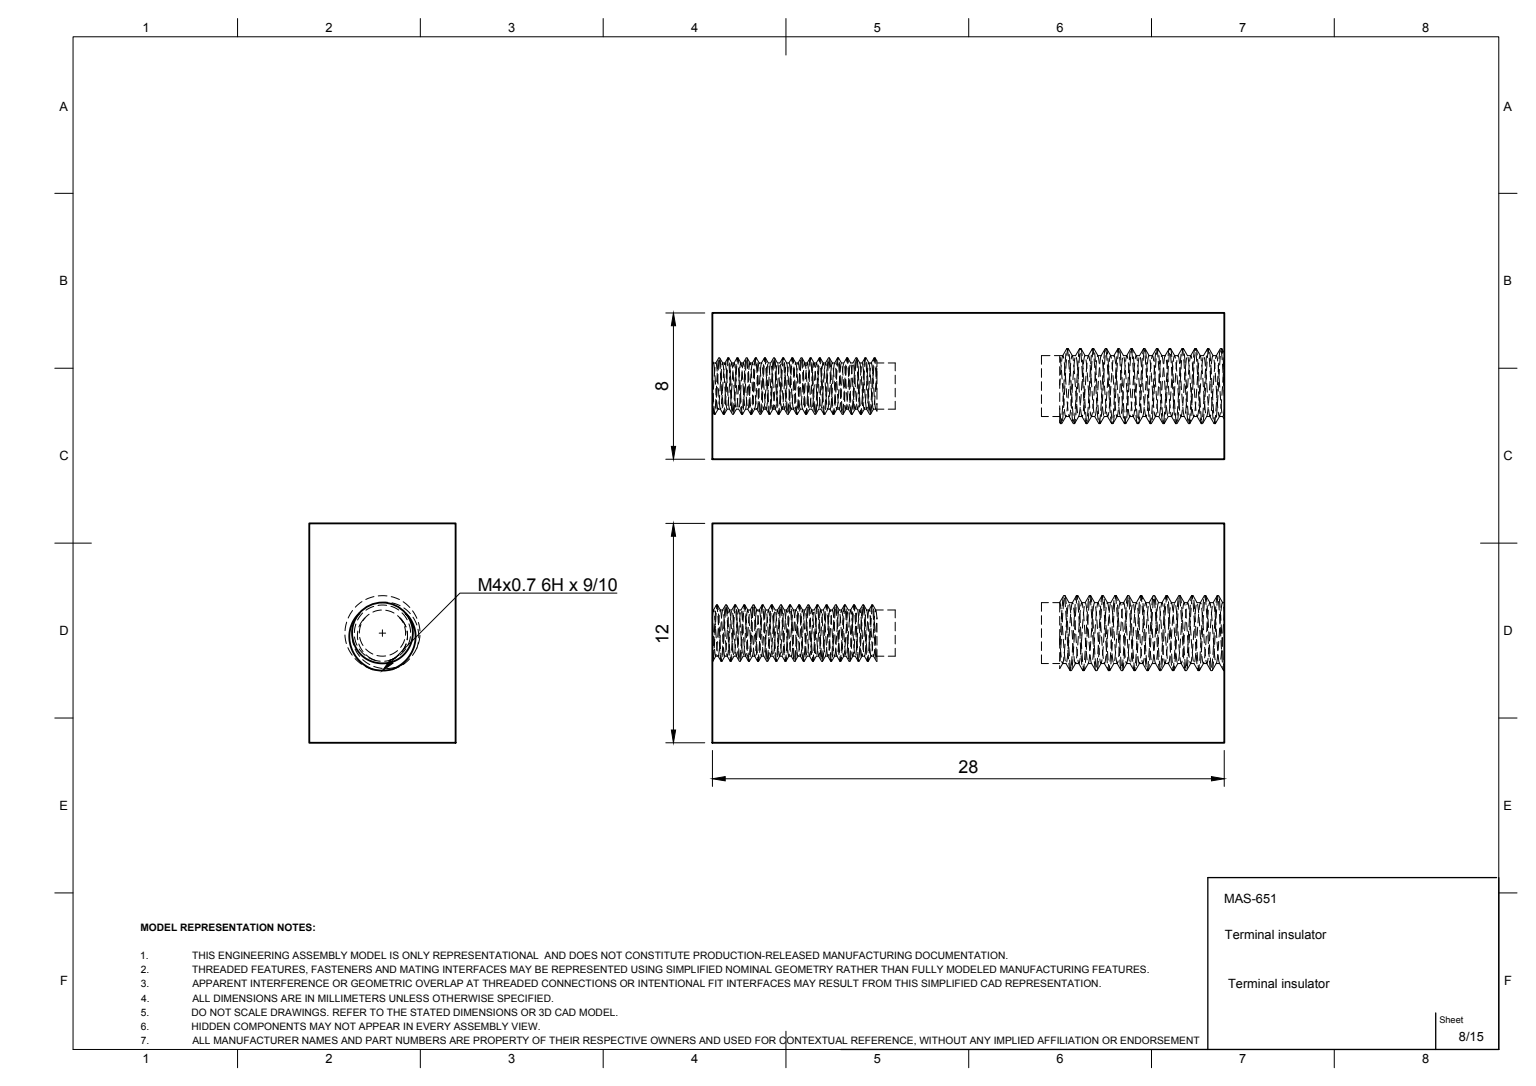
ISO-10303-21;
HEADER;
/* Generated by software containing ST-Developer
 * from STEP Tools, Inc. (www.steptools.com) 
 */

FILE_DESCRIPTION(
/* description */ ('Independent direct-acting normally-closed roller-plunger limit-switch
 CAD. Removable cover, insulated terminal supports, captured bus/conta
ct bridge, native Coil return spring, integral lower travel stop, reus
able instanced hardware and free roller. Manual geometric contact open
ing4mm; no snap-action/contact-force, electrical/current/voltage, envi
ronmental seal, safety-switch, wear, load or life certification. Exter
nal wiring and anchors omitted; fits and application engineering requi
red.'),
/* implementation_level */ '2;1');

FILE_NAME(
/* name */ 'Terminal insulator.step',
/* time_stamp */ '2026-11-08T07:32:43-08:00',
/* author */ (''),
/* organization */ (''),
/* preprocessor_version */ 'ST-DEVELOPER v20.2',
/* originating_system */ 'Autodesk Translation Framework v15.17.0.0',
/* authorisation */ '');

FILE_SCHEMA (('AUTOMOTIVE_DESIGN { 1 0 10303 214 3 1 1 }'));
ENDSEC;

DATA;
#10=MECHANICAL_DESIGN_GEOMETRIC_PRESENTATION_REPRESENTATION('',(#182),#36482);
#148=SHAPE_REPRESENTATION_RELATIONSHIP('SRR','None',#36561,#165);
#165=ADVANCED_BREP_SHAPE_REPRESENTATION('',(#199),#36471);
#182=STYLED_ITEM('',(#36655),#199);
#199=MANIFOLD_SOLID_BREP('Body1',#9773);
#222=B_SPLINE_SURFACE_WITH_KNOTS('',3,3,((#25543,#25544,#25545,#25546,#25547,
#25548,#25549,#25550,#25551,#25552,#25553,#25554,#25555,#25556,#25557,#25558,
#25559,#25560,#25561,#25562,#25563,#25564,#25565,#25566,#25567,#25568,#25569,
#25570,#25571,#25572,#25573,#25574,#25575,#25576,#25577,#25578,#25579,#25580,
#25581,#25582,#25583,#25584,#25585,#25586,#25587,#25588,#25589,#25590,#25591,
#25592,#25593,#25594,#25595,#25596,#25597,#25598,#25599,#25600,#25601,#25602,
#25603,#25604,#25605,#25606,#25607,#25608,#25609,#25610,#25611,#25612,#25613,
#25614,#25615,#25616,#25617,#25618,#25619,#25620,#25621,#25622,#25623,#25624,
#25625,#25626,#25627,#25628,#25629,#25630,#25631,#25632,#25633,#25634,#25635,
#25636,#25637,#25638,#25639,#25640,#25641,#25642,#25643,#25644,#25645,#25646,
#25647,#25648,#25649,#25650,#25651,#25652,#25653,#25654,#25655,#25656,#25657,
#25658,#25659,#25660,#25661),(#25662,#25663,#25664,#25665,#25666,#25667,
#25668,#25669,#25670,#25671,#25672,#25673,#25674,#25675,#25676,#25677,#25678,
#25679,#25680,#25681,#25682,#25683,#25684,#25685,#25686,#25687,#25688,#25689,
#25690,#25691,#25692,#25693,#25694,#25695,#25696,#25697,#25698,#25699,#25700,
#25701,#25702,#25703,#25704,#25705,#25706,#25707,#25708,#25709,#25710,#25711,
#25712,#25713,#25714,#25715,#25716,#25717,#25718,#25719,#25720,#25721,#25722,
#25723,#25724,#25725,#25726,#25727,#25728,#25729,#25730,#25731,#25732,#25733,
#25734,#25735,#25736,#25737,#25738,#25739,#25740,#25741,#25742,#25743,#25744,
#25745,#25746,#25747,#25748,#25749,#25750,#25751,#25752,#25753,#25754,#25755,
#25756,#25757,#25758,#25759,#25760,#25761,#25762,#25763,#25764,#25765,#25766,
#25767,#25768,#25769,#25770,#25771,#25772,#25773,#25774,#25775,#25776,#25777,
#25778,#25779,#25780),(#25781,#25782,#25783,#25784,#25785,#25786,#25787,
#25788,#25789,#25790,#25791,#25792,#25793,#25794,#25795,#25796,#25797,#25798,
#25799,#25800,#25801,#25802,#25803,#25804,#25805,#25806,#25807,#25808,#25809,
#25810,#25811,#25812,#25813,#25814,#25815,#25816,#25817,#25818,#25819,#25820,
#25821,#25822,#25823,#25824,#25825,#25826,#25827,#25828,#25829,#25830,#25831,
#25832,#25833,#25834,#25835,#25836,#25837,#25838,#25839,#25840,#25841,#25842,
#25843,#25844,#25845,#25846,#25847,#25848,#25849,#25850,#25851,#25852,#25853,
#25854,#25855,#25856,#25857,#25858,#25859,#25860,#25861,#25862,#25863,#25864,
#25865,#25866,#25867,#25868,#25869,#25870,#25871,#25872,#25873,#25874,#25875,
#25876,#25877,#25878,#25879,#25880,#25881,#25882,#25883,#25884,#25885,#25886,
#25887,#25888,#25889,#25890,#25891,#25892,#25893,#25894,#25895,#25896,#25897,
#25898,#25899),(#25900,#25901,#25902,#25903,#25904,#25905,#25906,#25907,
#25908,#25909,#25910,#25911,#25912,#25913,#25914,#25915,#25916,#25917,#25918,
#25919,#25920,#25921,#25922,#25923,#25924,#25925,#25926,#25927,#25928,#25929,
#25930,#25931,#25932,#25933,#25934,#25935,#25936,#25937,#25938,#25939,#25940,
#25941,#25942,#25943,#25944,#25945,#25946,#25947,#25948,#25949,#25950,#25951,
#25952,#25953,#25954,#25955,#25956,#25957,#25958,#25959,#25960,#25961,#25962,
#25963,#25964,#25965,#25966,#25967,#25968,#25969,#25970,#25971,#25972,#25973,
#25974,#25975,#25976,#25977,#25978,#25979,#25980,#25981,#25982,#25983,#25984,
#25985,#25986,#25987,#25988,#25989,#25990,#25991,#25992,#25993,#25994,#25995,
#25996,#25997,#25998,#25999,#26000,#26001,#26002,#26003,#26004,#26005,#26006,
#26007,#26008,#26009,#26010,#26011,#26012,#26013,#26014,#26015,#26016,#26017,
#26018)),.UNSPECIFIED.,.F.,.F.,.F.,(4,4),(4,1,1,1,1,1,1,1,1,1,1,1,1,1,1,
1,1,1,1,1,1,1,1,1,1,1,1,1,1,1,1,1,1,1,1,1,1,1,1,1,1,1,1,1,1,1,1,1,1,1,1,
1,1,1,1,1,1,1,1,1,1,1,1,1,1,1,1,1,1,1,1,1,1,1,1,1,1,1,1,1,1,1,1,1,1,1,1,
1,1,1,1,1,1,1,1,1,1,1,1,1,1,1,1,1,1,1,1,1,1,1,1,1,1,1,1,1,4),(0.,0.0321584099938621),
(11.8553612635792,12.8477570223809,13.8401527811825,14.8325485399841,15.8249442987858,
16.8173400575874,17.809735816389,18.8021315751907,19.7945273339923,20.7869230927939,
21.7793188515956,22.7717146103972,23.7641103691988,24.7565061280005,25.7489018868021,
26.7412976456037,27.7336934044054,28.726089163207,29.7184849220086,30.7108806808103,
31.7032764396119,32.6956721984135,33.6880679572152,34.6804637160168,35.6728594748184,
36.6652552336201,37.6576509924217,38.6500467512233,39.642442510025,40.6348382688266,
41.6272340276282,42.6196297864299,43.6120255452315,44.6044213040331,45.5968170628348,
46.5892128216364,47.581608580438,48.5740043392397,49.5664000980413,50.5587958568429,
51.5511916156446,52.5435873744462,53.5359831332478,54.5283788920495,55.5207746508511,
56.5131704096527,57.5055661684544,58.497961927256,59.4903576860576,60.4827534448593,
61.4751492036609,62.4675449624625,63.4599407212642,64.4523364800658,65.4447322388674,
66.4371279976691,67.4295237564707,68.4219195152723,69.4143152740739,70.4067110328756,
71.3991067916772,72.3915025504788,73.3838983092805,74.3762940680821,75.3686898268838,
76.3610855856854,77.353481344487,78.3458771032886,79.3382728620903,80.3306686208919,
81.3230643796935,82.3154601384952,83.3078558972968,84.3002516560985,85.2926474149001,
86.2850431737017,87.2774389325033,88.269834691305,89.2622304501066,90.2546262089082,
91.2470219677099,92.2394177265115,93.2318134853131,94.2242092441148,95.2166050029164,
96.209000761718,97.2013965205197,98.1937922793213,99.1861880381229,100.178583796925,
101.170979555726,102.163375314528,103.155771073329,104.148166832131,105.140562590933,
106.132958349734,107.125354108536,108.117749867338,109.110145626139,110.102541384941,
111.094937143743,112.087332902544,113.079728661346,114.072124420147,115.064520178949,
116.056915937751,117.049311696552,118.041707455354,119.034103214156,120.026498972957,
121.018894731759,122.01129049056,123.003686249362,123.996082008164,124.988477766965,
125.980873525767,126.973269284569),.UNSPECIFIED.);
#223=B_SPLINE_SURFACE_WITH_KNOTS('',3,3,((#26093,#26094,#26095,#26096,#26097,
#26098,#26099,#26100,#26101,#26102,#26103,#26104,#26105,#26106,#26107,#26108,
#26109,#26110,#26111,#26112,#26113,#26114,#26115,#26116,#26117,#26118,#26119,
#26120,#26121,#26122,#26123,#26124,#26125,#26126,#26127,#26128,#26129,#26130,
#26131,#26132,#26133,#26134,#26135,#26136,#26137,#26138,#26139,#26140,#26141,
#26142,#26143,#26144,#26145,#26146,#26147,#26148,#26149,#26150,#26151,#26152,
#26153,#26154,#26155,#26156,#26157,#26158,#26159,#26160,#26161,#26162,#26163,
#26164,#26165,#26166,#26167,#26168,#26169,#26170,#26171,#26172,#26173,#26174,
#26175,#26176,#26177,#26178,#26179,#26180,#26181,#26182,#26183,#26184,#26185,
#26186,#26187,#26188,#26189,#26190,#26191,#26192,#26193,#26194,#26195,#26196,
#26197,#26198,#26199,#26200,#26201,#26202,#26203,#26204,#26205,#26206,#26207,
#26208,#26209,#26210,#26211),(#26212,#26213,#26214,#26215,#26216,#26217,
#26218,#26219,#26220,#26221,#26222,#26223,#26224,#26225,#26226,#26227,#26228,
#26229,#26230,#26231,#26232,#26233,#26234,#26235,#26236,#26237,#26238,#26239,
#26240,#26241,#26242,#26243,#26244,#26245,#26246,#26247,#26248,#26249,#26250,
#26251,#26252,#26253,#26254,#26255,#26256,#26257,#26258,#26259,#26260,#26261,
#26262,#26263,#26264,#26265,#26266,#26267,#26268,#26269,#26270,#26271,#26272,
#26273,#26274,#26275,#26276,#26277,#26278,#26279,#26280,#26281,#26282,#26283,
#26284,#26285,#26286,#26287,#26288,#26289,#26290,#26291,#26292,#26293,#26294,
#26295,#26296,#26297,#26298,#26299,#26300,#26301,#26302,#26303,#26304,#26305,
#26306,#26307,#26308,#26309,#26310,#26311,#26312,#26313,#26314,#26315,#26316,
#26317,#26318,#26319,#26320,#26321,#26322,#26323,#26324,#26325,#26326,#26327,
#26328,#26329,#26330),(#26331,#26332,#26333,#26334,#26335,#26336,#26337,
#26338,#26339,#26340,#26341,#26342,#26343,#26344,#26345,#26346,#26347,#26348,
#26349,#26350,#26351,#26352,#26353,#26354,#26355,#26356,#26357,#26358,#26359,
#26360,#26361,#26362,#26363,#26364,#26365,#26366,#26367,#26368,#26369,#26370,
#26371,#26372,#26373,#26374,#26375,#26376,#26377,#26378,#26379,#26380,#26381,
#26382,#26383,#26384,#26385,#26386,#26387,#26388,#26389,#26390,#26391,#26392,
#26393,#26394,#26395,#26396,#26397,#26398,#26399,#26400,#26401,#26402,#26403,
#26404,#26405,#26406,#26407,#26408,#26409,#26410,#26411,#26412,#26413,#26414,
#26415,#26416,#26417,#26418,#26419,#26420,#26421,#26422,#26423,#26424,#26425,
#26426,#26427,#26428,#26429,#26430,#26431,#26432,#26433,#26434,#26435,#26436,
#26437,#26438,#26439,#26440,#26441,#26442,#26443,#26444,#26445,#26446,#26447,
#26448,#26449),(#26450,#26451,#26452,#26453,#26454,#26455,#26456,#26457,
#26458,#26459,#26460,#26461,#26462,#26463,#26464,#26465,#26466,#26467,#26468,
#26469,#26470,#26471,#26472,#26473,#26474,#26475,#26476,#26477,#26478,#26479,
#26480,#26481,#26482,#26483,#26484,#26485,#26486,#26487,#26488,#26489,#26490,
#26491,#26492,#26493,#26494,#26495,#26496,#26497,#26498,#26499,#26500,#26501,
#26502,#26503,#26504,#26505,#26506,#26507,#26508,#26509,#26510,#26511,#26512,
#26513,#26514,#26515,#26516,#26517,#26518,#26519,#26520,#26521,#26522,#26523,
#26524,#26525,#26526,#26527,#26528,#26529,#26530,#26531,#26532,#26533,#26534,
#26535,#26536,#26537,#26538,#26539,#26540,#26541,#26542,#26543,#26544,#26545,
#26546,#26547,#26548,#26549,#26550,#26551,#26552,#26553,#26554,#26555,#26556,
#26557,#26558,#26559,#26560,#26561,#26562,#26563,#26564,#26565,#26566,#26567,
#26568)),.UNSPECIFIED.,.F.,.F.,.F.,(4,4),(4,1,1,1,1,1,1,1,1,1,1,1,1,1,1,
1,1,1,1,1,1,1,1,1,1,1,1,1,1,1,1,1,1,1,1,1,1,1,1,1,1,1,1,1,1,1,1,1,1,1,1,
1,1,1,1,1,1,1,1,1,1,1,1,1,1,1,1,1,1,1,1,1,1,1,1,1,1,1,1,1,1,1,1,1,1,1,1,
1,1,1,1,1,1,1,1,1,1,1,1,1,1,1,1,1,1,1,1,1,1,1,1,1,1,1,1,1,4),(0.,0.0321584099938621),
(14.3984001269718,15.3907958857734,16.383191644575,17.3755874033767,18.3679831621783,
19.3603789209799,20.3527746797816,21.3451704385832,22.3375661973848,23.3299619561865,
24.3223577149881,25.3147534737897,26.3071492325914,27.299544991393,28.2919407501946,
29.2843365089963,30.2767322677979,31.2691280265995,32.2615237854012,33.2539195442028,
34.2463153030044,35.2387110618061,36.2311068206077,37.2235025794093,38.215898338211,
39.2082940970126,40.2006898558142,41.1930856146159,42.1854813734175,43.1778771322191,
44.1702728910208,45.1626686498224,46.155064408624,47.1474601674257,48.1398559262273,
49.1322516850289,50.1246474438306,51.1170432026322,52.1094389614338,53.1018347202355,
54.0942304790371,55.0866262378387,56.0790219966403,57.071417755442,58.0638135142436,
59.0562092730452,60.0486050318469,61.0410007906485,62.0333965494501,63.0257923082518,
64.0181880670534,65.010583825855,66.0029795846567,66.9953753434583,67.9877711022599,
68.9801668610616,69.9725626198632,70.9649583786648,71.9573541374665,72.9497498962681,
73.9421456550697,74.9345414138714,75.926937172673,76.9193329314746,77.9117286902763,
78.9041244490779,79.8965202078795,80.8889159666812,81.8813117254828,82.8737074842844,
83.8661032430861,84.8584990018877,85.8508947606893,86.8432905194909,87.8356862782926,
88.8280820370942,89.8204777958959,90.8128735546975,91.8052693134991,92.7976650723007,
93.7900608311024,94.782456589904,95.7748523487057,96.7672481075073,97.7596438663089,
98.7520396251105,99.7444353839122,100.736831142714,101.729226901515,102.721622660317,
103.714018419119,104.70641417792,105.698809936722,106.691205695524,107.683601454325,
108.675997213127,109.668392971929,110.66078873073,111.653184489532,112.645580248333,
113.637976007135,114.630371765937,115.622767524738,116.61516328354,117.607559042342,
118.599954801143,119.592350559945,120.584746318746,121.577142077548,122.56953783635,
123.561933595151,124.554329353953,125.546725112755,126.539120871556,127.531516630358,
128.52391238916,129.516308147961),.UNSPECIFIED.);
#224=B_SPLINE_SURFACE_WITH_KNOTS('',3,3,((#26775,#26776,#26777,#26778,#26779,
#26780,#26781,#26782,#26783,#26784,#26785,#26786,#26787,#26788,#26789,#26790,
#26791,#26792,#26793,#26794,#26795,#26796,#26797,#26798,#26799,#26800,#26801,
#26802,#26803,#26804,#26805,#26806,#26807,#26808,#26809,#26810,#26811,#26812,
#26813,#26814,#26815,#26816,#26817,#26818,#26819,#26820,#26821,#26822,#26823,
#26824,#26825,#26826,#26827,#26828,#26829,#26830,#26831,#26832,#26833,#26834,
#26835,#26836,#26837,#26838,#26839,#26840,#26841,#26842,#26843,#26844,#26845,
#26846,#26847,#26848,#26849,#26850,#26851,#26852,#26853,#26854,#26855,#26856,
#26857,#26858,#26859,#26860),(#26861,#26862,#26863,#26864,#26865,#26866,
#26867,#26868,#26869,#26870,#26871,#26872,#26873,#26874,#26875,#26876,#26877,
#26878,#26879,#26880,#26881,#26882,#26883,#26884,#26885,#26886,#26887,#26888,
#26889,#26890,#26891,#26892,#26893,#26894,#26895,#26896,#26897,#26898,#26899,
#26900,#26901,#26902,#26903,#26904,#26905,#26906,#26907,#26908,#26909,#26910,
#26911,#26912,#26913,#26914,#26915,#26916,#26917,#26918,#26919,#26920,#26921,
#26922,#26923,#26924,#26925,#26926,#26927,#26928,#26929,#26930,#26931,#26932,
#26933,#26934,#26935,#26936,#26937,#26938,#26939,#26940,#26941,#26942,#26943,
#26944,#26945,#26946),(#26947,#26948,#26949,#26950,#26951,#26952,#26953,
#26954,#26955,#26956,#26957,#26958,#26959,#26960,#26961,#26962,#26963,#26964,
#26965,#26966,#26967,#26968,#26969,#26970,#26971,#26972,#26973,#26974,#26975,
#26976,#26977,#26978,#26979,#26980,#26981,#26982,#26983,#26984,#26985,#26986,
#26987,#26988,#26989,#26990,#26991,#26992,#26993,#26994,#26995,#26996,#26997,
#26998,#26999,#27000,#27001,#27002,#27003,#27004,#27005,#27006,#27007,#27008,
#27009,#27010,#27011,#27012,#27013,#27014,#27015,#27016,#27017,#27018,#27019,
#27020,#27021,#27022,#27023,#27024,#27025,#27026,#27027,#27028,#27029,#27030,
#27031,#27032),(#27033,#27034,#27035,#27036,#27037,#27038,#27039,#27040,
#27041,#27042,#27043,#27044,#27045,#27046,#27047,#27048,#27049,#27050,#27051,
#27052,#27053,#27054,#27055,#27056,#27057,#27058,#27059,#27060,#27061,#27062,
#27063,#27064,#27065,#27066,#27067,#27068,#27069,#27070,#27071,#27072,#27073,
#27074,#27075,#27076,#27077,#27078,#27079,#27080,#27081,#27082,#27083,#27084,
#27085,#27086,#27087,#27088,#27089,#27090,#27091,#27092,#27093,#27094,#27095,
#27096,#27097,#27098,#27099,#27100,#27101,#27102,#27103,#27104,#27105,#27106,
#27107,#27108,#27109,#27110,#27111,#27112,#27113,#27114,#27115,#27116,#27117,
#27118)),.UNSPECIFIED.,.F.,.F.,.F.,(4,4),(4,1,1,1,1,1,1,1,1,1,1,1,1,1,1,
1,1,1,1,1,1,1,1,1,1,1,1,1,1,1,1,1,1,1,1,1,1,1,1,1,1,1,1,1,1,1,1,1,1,1,1,
1,1,1,1,1,1,1,1,1,1,1,1,1,1,1,1,1,1,1,1,1,1,1,1,1,1,1,1,1,1,1,1,4),(0.,
0.0448889834294934),(11.8615800042567,12.8591513772396,13.8567227502225,
14.8542941232054,15.8518654961884,16.8494368691713,17.8470082421542,18.8445796151372,
19.8421509881201,20.839722361103,21.837293734086,22.8348651070689,23.8324364800518,
24.8300078530348,25.8275792260177,26.8251505990006,27.8227219719836,28.8202933449665,
29.8178647179494,30.8154360909324,31.8130074639153,32.8105788368982,33.8081502098812,
34.8057215828641,35.803292955847,36.80086432883,37.7984357018129,38.7960070747958,
39.7935784477788,40.7911498207617,41.7887211937446,42.7862925667276,43.7838639397105,
44.7814353126934,45.7790066856764,46.7765780586593,47.7741494316422,48.7717208046252,
49.7692921776081,50.766863550591,51.764434923574,52.7620062965569,53.7595776695398,
54.7571490425228,55.7547204155057,56.7522917884886,57.7498631614716,58.7474345344545,
59.7450059074374,60.7425772804204,61.7401486534033,62.7377200263862,63.7352913993692,
64.7328627723521,65.730434145335,66.728005518318,67.7255768913009,68.7231482642838,
69.7207196372668,70.7182910102497,71.7158623832326,72.7134337562156,73.7110051291985,
74.7085765021814,75.7061478751643,76.7037192481473,77.7012906211302,78.6988619941132,
79.6964333670961,80.694004740079,81.691576113062,82.6891474860449,83.6867188590278,
84.6842902320108,85.6818616049937,86.6794329779766,87.6770043509595,88.6745757239425,
89.6721470969254,90.6697184699083,91.6672898428913,92.6648612158742,93.6624325888571,
94.6600039618401),.UNSPECIFIED.);
#225=B_SPLINE_SURFACE_WITH_KNOTS('',3,3,((#27196,#27197,#27198,#27199,#27200,
#27201,#27202,#27203,#27204,#27205,#27206,#27207,#27208,#27209,#27210,#27211,
#27212,#27213,#27214,#27215,#27216,#27217,#27218,#27219,#27220,#27221,#27222,
#27223,#27224,#27225,#27226,#27227,#27228,#27229,#27230,#27231,#27232,#27233,
#27234,#27235,#27236,#27237,#27238,#27239,#27240,#27241,#27242,#27243,#27244,
#27245,#27246,#27247,#27248,#27249,#27250,#27251,#27252,#27253,#27254,#27255,
#27256,#27257,#27258,#27259,#27260,#27261,#27262,#27263,#27264,#27265,#27266,
#27267,#27268,#27269,#27270,#27271,#27272,#27273,#27274,#27275,#27276,#27277,
#27278,#27279,#27280,#27281),(#27282,#27283,#27284,#27285,#27286,#27287,
#27288,#27289,#27290,#27291,#27292,#27293,#27294,#27295,#27296,#27297,#27298,
#27299,#27300,#27301,#27302,#27303,#27304,#27305,#27306,#27307,#27308,#27309,
#27310,#27311,#27312,#27313,#27314,#27315,#27316,#27317,#27318,#27319,#27320,
#27321,#27322,#27323,#27324,#27325,#27326,#27327,#27328,#27329,#27330,#27331,
#27332,#27333,#27334,#27335,#27336,#27337,#27338,#27339,#27340,#27341,#27342,
#27343,#27344,#27345,#27346,#27347,#27348,#27349,#27350,#27351,#27352,#27353,
#27354,#27355,#27356,#27357,#27358,#27359,#27360,#27361,#27362,#27363,#27364,
#27365,#27366,#27367),(#27368,#27369,#27370,#27371,#27372,#27373,#27374,
#27375,#27376,#27377,#27378,#27379,#27380,#27381,#27382,#27383,#27384,#27385,
#27386,#27387,#27388,#27389,#27390,#27391,#27392,#27393,#27394,#27395,#27396,
#27397,#27398,#27399,#27400,#27401,#27402,#27403,#27404,#27405,#27406,#27407,
#27408,#27409,#27410,#27411,#27412,#27413,#27414,#27415,#27416,#27417,#27418,
#27419,#27420,#27421,#27422,#27423,#27424,#27425,#27426,#27427,#27428,#27429,
#27430,#27431,#27432,#27433,#27434,#27435,#27436,#27437,#27438,#27439,#27440,
#27441,#27442,#27443,#27444,#27445,#27446,#27447,#27448,#27449,#27450,#27451,
#27452,#27453),(#27454,#27455,#27456,#27457,#27458,#27459,#27460,#27461,
#27462,#27463,#27464,#27465,#27466,#27467,#27468,#27469,#27470,#27471,#27472,
#27473,#27474,#27475,#27476,#27477,#27478,#27479,#27480,#27481,#27482,#27483,
#27484,#27485,#27486,#27487,#27488,#27489,#27490,#27491,#27492,#27493,#27494,
#27495,#27496,#27497,#27498,#27499,#27500,#27501,#27502,#27503,#27504,#27505,
#27506,#27507,#27508,#27509,#27510,#27511,#27512,#27513,#27514,#27515,#27516,
#27517,#27518,#27519,#27520,#27521,#27522,#27523,#27524,#27525,#27526,#27527,
#27528,#27529,#27530,#27531,#27532,#27533,#27534,#27535,#27536,#27537,#27538,
#27539)),.UNSPECIFIED.,.F.,.F.,.F.,(4,4),(4,1,1,1,1,1,1,1,1,1,1,1,1,1,1,
1,1,1,1,1,1,1,1,1,1,1,1,1,1,1,1,1,1,1,1,1,1,1,1,1,1,1,1,1,1,1,1,1,1,1,1,
1,1,1,1,1,1,1,1,1,1,1,1,1,1,1,1,1,1,1,1,1,1,1,1,1,1,1,1,1,1,1,1,4),(0.,
0.0448889834294934),(14.3981410127769,15.3957123857598,16.3932837587428,
17.3908551317257,18.3884265047086,19.3859978776916,20.3835692506745,21.3811406236574,
22.3787119966404,23.3762833696233,24.3738547426062,25.3714261155892,26.3689974885721,
27.366568861555,28.364140234538,29.3617116075209,30.3592829805038,31.3568543534868,
32.3544257264697,33.3519970994526,34.3495684724355,35.3471398454185,36.3447112184014,
37.3422825913843,38.3398539643673,39.3374253373502,40.3349967103331,41.3325680833161,
42.330139456299,43.3277108292819,44.3252822022649,45.3228535752478,46.3204249482307,
47.3179963212137,48.3155676941966,49.3131390671795,50.3107104401625,51.3082818131454,
52.3058531861283,53.3034245591113,54.3009959320942,55.2985673050771,56.2961386780601,
57.293710051043,58.2912814240259,59.2888527970089,60.2864241699918,61.2839955429747,
62.2815669159577,63.2791382889406,64.2767096619235,65.2742810349065,66.2718524078894,
67.2694237808723,68.2669951538553,69.2645665268382,70.2621378998211,71.2597092728041,
72.257280645787,73.2548520187699,74.2524233917529,75.2499947647358,76.2475661377187,
77.2451375107017,78.2427088836846,79.2402802566675,80.2378516296505,81.2354230026334,
82.2329943756163,83.2305657485993,84.2281371215822,85.2257084945651,86.2232798675481,
87.220851240531,88.2184226135139,89.2159939864969,90.2135653594798,91.2111367324627,
92.2087081054457,93.2062794784286,94.2038508514115,95.2014222243944,96.1989935973774,
97.1965649703603),.UNSPECIFIED.);
#282=FACE_BOUND('',#1357,.T.);
#283=FACE_BOUND('',#1359,.T.);
#368=PLANE('',#10387);
#369=PLANE('',#10390);
#370=PLANE('',#10391);
#371=PLANE('',#10394);
#372=PLANE('',#10395);
#373=PLANE('',#10396);
#374=PLANE('',#10397);
#375=PLANE('',#10398);
#376=PLANE('',#10399);
#377=PLANE('',#10400);
#694=FACE_OUTER_BOUND('',#1279,.T.);
#695=FACE_OUTER_BOUND('',#1280,.T.);
#696=FACE_OUTER_BOUND('',#1281,.T.);
#697=FACE_OUTER_BOUND('',#1282,.T.);
#698=FACE_OUTER_BOUND('',#1283,.T.);
#699=FACE_OUTER_BOUND('',#1284,.T.);
#700=FACE_OUTER_BOUND('',#1285,.T.);
#701=FACE_OUTER_BOUND('',#1286,.T.);
#702=FACE_OUTER_BOUND('',#1287,.T.);
#703=FACE_OUTER_BOUND('',#1288,.T.);
#704=FACE_OUTER_BOUND('',#1289,.T.);
#705=FACE_OUTER_BOUND('',#1290,.T.);
#706=FACE_OUTER_BOUND('',#1291,.T.);
#707=FACE_OUTER_BOUND('',#1292,.T.);
#708=FACE_OUTER_BOUND('',#1293,.T.);
#709=FACE_OUTER_BOUND('',#1294,.T.);
#710=FACE_OUTER_BOUND('',#1295,.T.);
#711=FACE_OUTER_BOUND('',#1296,.T.);
#712=FACE_OUTER_BOUND('',#1297,.T.);
#713=FACE_OUTER_BOUND('',#1298,.T.);
#714=FACE_OUTER_BOUND('',#1299,.T.);
#715=FACE_OUTER_BOUND('',#1300,.T.);
#716=FACE_OUTER_BOUND('',#1301,.T.);
#717=FACE_OUTER_BOUND('',#1302,.T.);
#718=FACE_OUTER_BOUND('',#1303,.T.);
#719=FACE_OUTER_BOUND('',#1304,.T.);
#720=FACE_OUTER_BOUND('',#1305,.T.);
#721=FACE_OUTER_BOUND('',#1306,.T.);
#722=FACE_OUTER_BOUND('',#1307,.T.);
#723=FACE_OUTER_BOUND('',#1308,.T.);
#724=FACE_OUTER_BOUND('',#1309,.T.);
#725=FACE_OUTER_BOUND('',#1310,.T.);
#726=FACE_OUTER_BOUND('',#1311,.T.);
#727=FACE_OUTER_BOUND('',#1312,.T.);
#728=FACE_OUTER_BOUND('',#1313,.T.);
#729=FACE_OUTER_BOUND('',#1314,.T.);
#730=FACE_OUTER_BOUND('',#1315,.T.);
#731=FACE_OUTER_BOUND('',#1316,.T.);
#732=FACE_OUTER_BOUND('',#1317,.T.);
#733=FACE_OUTER_BOUND('',#1318,.T.);
#734=FACE_OUTER_BOUND('',#1319,.T.);
#735=FACE_OUTER_BOUND('',#1320,.T.);
#736=FACE_OUTER_BOUND('',#1321,.T.);
#737=FACE_OUTER_BOUND('',#1322,.T.);
#738=FACE_OUTER_BOUND('',#1323,.T.);
#739=FACE_OUTER_BOUND('',#1324,.T.);
#740=FACE_OUTER_BOUND('',#1325,.T.);
#741=FACE_OUTER_BOUND('',#1326,.T.);
#742=FACE_OUTER_BOUND('',#1327,.T.);
#743=FACE_OUTER_BOUND('',#1328,.T.);
#744=FACE_OUTER_BOUND('',#1329,.T.);
#745=FACE_OUTER_BOUND('',#1330,.T.);
#746=FACE_OUTER_BOUND('',#1331,.T.);
#747=FACE_OUTER_BOUND('',#1332,.T.);
#748=FACE_OUTER_BOUND('',#1333,.T.);
#749=FACE_OUTER_BOUND('',#1334,.T.);
#750=FACE_OUTER_BOUND('',#1335,.T.);
#751=FACE_OUTER_BOUND('',#1336,.T.);
#752=FACE_OUTER_BOUND('',#1337,.T.);
#753=FACE_OUTER_BOUND('',#1338,.T.);
#754=FACE_OUTER_BOUND('',#1339,.T.);
#755=FACE_OUTER_BOUND('',#1340,.T.);
#756=FACE_OUTER_BOUND('',#1341,.T.);
#757=FACE_OUTER_BOUND('',#1342,.T.);
#758=FACE_OUTER_BOUND('',#1343,.T.);
#759=FACE_OUTER_BOUND('',#1344,.T.);
#760=FACE_OUTER_BOUND('',#1345,.T.);
#761=FACE_OUTER_BOUND('',#1346,.T.);
#762=FACE_OUTER_BOUND('',#1347,.T.);
#763=FACE_OUTER_BOUND('',#1348,.T.);
#764=FACE_OUTER_BOUND('',#1349,.T.);
#765=FACE_OUTER_BOUND('',#1350,.T.);
#766=FACE_OUTER_BOUND('',#1351,.T.);
#767=FACE_OUTER_BOUND('',#1352,.T.);
#768=FACE_OUTER_BOUND('',#1353,.T.);
#769=FACE_OUTER_BOUND('',#1354,.T.);
#770=FACE_OUTER_BOUND('',#1355,.T.);
#771=FACE_OUTER_BOUND('',#1356,.T.);
#772=FACE_OUTER_BOUND('',#1358,.T.);
#1279=EDGE_LOOP('',(#7366,#7367,#7368,#7369,#7370,#7371,#7372,#7373));
#1280=EDGE_LOOP('',(#7374,#7375,#7376,#7377));
#1281=EDGE_LOOP('',(#7378,#7379,#7380,#7381));
#1282=EDGE_LOOP('',(#7382,#7383,#7384,#7385));
#1283=EDGE_LOOP('',(#7386,#7387,#7388,#7389));
#1284=EDGE_LOOP('',(#7390,#7391,#7392,#7393));
#1285=EDGE_LOOP('',(#7394,#7395,#7396,#7397));
#1286=EDGE_LOOP('',(#7398,#7399,#7400,#7401));
#1287=EDGE_LOOP('',(#7402,#7403,#7404,#7405));
#1288=EDGE_LOOP('',(#7406,#7407,#7408,#7409));
#1289=EDGE_LOOP('',(#7410,#7411,#7412,#7413));
#1290=EDGE_LOOP('',(#7414,#7415,#7416,#7417));
#1291=EDGE_LOOP('',(#7418,#7419,#7420,#7421));
#1292=EDGE_LOOP('',(#7422,#7423,#7424,#7425));
#1293=EDGE_LOOP('',(#7426,#7427,#7428,#7429));
#1294=EDGE_LOOP('',(#7430,#7431,#7432,#7433));
#1295=EDGE_LOOP('',(#7434,#7435,#7436,#7437));
#1296=EDGE_LOOP('',(#7438,#7439,#7440,#7441));
#1297=EDGE_LOOP('',(#7442,#7443,#7444,#7445));
#1298=EDGE_LOOP('',(#7446,#7447,#7448,#7449));
#1299=EDGE_LOOP('',(#7450,#7451,#7452,#7453));
#1300=EDGE_LOOP('',(#7454,#7455,#7456,#7457));
#1301=EDGE_LOOP('',(#7458,#7459,#7460,#7461));
#1302=EDGE_LOOP('',(#7462,#7463,#7464,#7465));
#1303=EDGE_LOOP('',(#7466,#7467,#7468,#7469));
#1304=EDGE_LOOP('',(#7470,#7471,#7472,#7473,#7474,#7475,#7476,#7477));
#1305=EDGE_LOOP('',(#7478,#7479,#7480,#7481));
#1306=EDGE_LOOP('',(#7482,#7483,#7484,#7485));
#1307=EDGE_LOOP('',(#7486,#7487,#7488,#7489));
#1308=EDGE_LOOP('',(#7490,#7491,#7492,#7493));
#1309=EDGE_LOOP('',(#7494,#7495,#7496,#7497));
#1310=EDGE_LOOP('',(#7498,#7499,#7500,#7501));
#1311=EDGE_LOOP('',(#7502,#7503,#7504,#7505));
#1312=EDGE_LOOP('',(#7506,#7507,#7508,#7509));
#1313=EDGE_LOOP('',(#7510,#7511,#7512,#7513));
#1314=EDGE_LOOP('',(#7514,#7515,#7516,#7517));
#1315=EDGE_LOOP('',(#7518,#7519,#7520,#7521));
#1316=EDGE_LOOP('',(#7522,#7523,#7524,#7525));
#1317=EDGE_LOOP('',(#7526,#7527,#7528,#7529));
#1318=EDGE_LOOP('',(#7530,#7531,#7532,#7533));
#1319=EDGE_LOOP('',(#7534,#7535,#7536,#7537));
#1320=EDGE_LOOP('',(#7538,#7539,#7540,#7541));
#1321=EDGE_LOOP('',(#7542,#7543,#7544,#7545));
#1322=EDGE_LOOP('',(#7546,#7547,#7548,#7549));
#1323=EDGE_LOOP('',(#7550,#7551,#7552,#7553));
#1324=EDGE_LOOP('',(#7554,#7555,#7556,#7557));
#1325=EDGE_LOOP('',(#7558,#7559,#7560,#7561));
#1326=EDGE_LOOP('',(#7562,#7563,#7564,#7565));
#1327=EDGE_LOOP('',(#7566,#7567,#7568,#7569));
#1328=EDGE_LOOP('',(#7570,#7571,#7572,#7573));
#1329=EDGE_LOOP('',(#7574,#7575,#7576,#7577));
#1330=EDGE_LOOP('',(#7578,#7579,#7580,#7581));
#1331=EDGE_LOOP('',(#7582,#7583,#7584,#7585));
#1332=EDGE_LOOP('',(#7586,#7587,#7588,#7589));
#1333=EDGE_LOOP('',(#7590,#7591,#7592,#7593));
#1334=EDGE_LOOP('',(#7594,#7595,#7596,#7597));
#1335=EDGE_LOOP('',(#7598,#7599,#7600,#7601));
#1336=EDGE_LOOP('',(#7602,#7603,#7604,#7605));
#1337=EDGE_LOOP('',(#7606,#7607,#7608,#7609));
#1338=EDGE_LOOP('',(#7610,#7611,#7612,#7613));
#1339=EDGE_LOOP('',(#7614,#7615,#7616,#7617));
#1340=EDGE_LOOP('',(#7618,#7619,#7620,#7621,#7622));
#1341=EDGE_LOOP('',(#7623,#7624,#7625,#7626));
#1342=EDGE_LOOP('',(#7627,#7628,#7629,#7630,#7631,#7632,#7633,#7634,#7635,
#7636,#7637,#7638,#7639,#7640,#7641,#7642,#7643,#7644,#7645,#7646,#7647,
#7648,#7649,#7650,#7651,#7652,#7653,#7654,#7655,#7656,#7657,#7658,#7659,
#7660,#7661,#7662,#7663,#7664,#7665,#7666));
#1343=EDGE_LOOP('',(#7667,#7668,#7669,#7670,#7671,#7672,#7673,#7674,#7675,
#7676,#7677,#7678,#7679,#7680,#7681,#7682,#7683,#7684,#7685,#7686,#7687,
#7688,#7689,#7690,#7691,#7692,#7693,#7694,#7695,#7696,#7697,#7698,#7699,
#7700,#7701,#7702,#7703,#7704,#7705,#7706));
#1344=EDGE_LOOP('',(#7707,#7708,#7709,#7710));
#1345=EDGE_LOOP('',(#7711));
#1346=EDGE_LOOP('',(#7712,#7713,#7714,#7715));
#1347=EDGE_LOOP('',(#7716,#7717,#7718,#7719));
#1348=EDGE_LOOP('',(#7720,#7721,#7722,#7723,#7724,#7725,#7726,#7727,#7728,
#7729,#7730,#7731,#7732,#7733,#7734,#7735,#7736,#7737,#7738,#7739,#7740,
#7741,#7742,#7743,#7744,#7745,#7746,#7747,#7748,#7749));
#1349=EDGE_LOOP('',(#7750,#7751,#7752,#7753,#7754,#7755,#7756,#7757,#7758,
#7759,#7760,#7761,#7762,#7763,#7764,#7765,#7766,#7767,#7768,#7769,#7770,
#7771,#7772,#7773,#7774,#7775,#7776,#7777,#7778));
#1350=EDGE_LOOP('',(#7779,#7780,#7781,#7782));
#1351=EDGE_LOOP('',(#7783));
#1352=EDGE_LOOP('',(#7784,#7785,#7786,#7787));
#1353=EDGE_LOOP('',(#7788,#7789,#7790,#7791));
#1354=EDGE_LOOP('',(#7792,#7793,#7794,#7795));
#1355=EDGE_LOOP('',(#7796,#7797,#7798,#7799));
#1356=EDGE_LOOP('',(#7800,#7801,#7802,#7803));
#1357=EDGE_LOOP('',(#7804,#7805,#7806,#7807));
#1358=EDGE_LOOP('',(#7808,#7809,#7810,#7811));
#1359=EDGE_LOOP('',(#7812,#7813,#7814,#7815));
#1674=CIRCLE('',#10316,0.1666);
#1675=CIRCLE('',#10317,0.1666);
#1676=CIRCLE('',#10329,0.1666);
#1677=CIRCLE('',#10331,0.205475);
#1678=CIRCLE('',#10344,0.205475);
#1679=CIRCLE('',#10346,0.12645);
#1680=CIRCLE('',#10347,0.12645);
#1681=CIRCLE('',#10348,0.12645);
#1682=CIRCLE('',#10366,0.12645);
#1683=CIRCLE('',#10368,0.1543);
#1684=CIRCLE('',#10386,0.1543);
#2054=B_SPLINE_CURVE_WITH_KNOTS('',3,(#23212,#23213,#23214,#23215,#23216,
#23217,#23218,#23219,#23220,#23221,#23222,#23223,#23224,#23225,#23226,#23227,
#23228,#23229,#23230,#23231,#23232,#23233),.UNSPECIFIED.,.F.,.F.,(4,3,3,
3,3,3,3,4),(76.7080459413271,76.8129957196858,77.8105670926688,78.8081384656517,
79.8057098386346,80.8032812116176,81.8008525846005,82.7984239575834),
 .UNSPECIFIED.);
#2055=B_SPLINE_CURVE_WITH_KNOTS('',3,(#23237,#23238,#23239,#23240,#23241,
#23242,#23243),.UNSPECIFIED.,.F.,.F.,(4,3,4),(-80.783811092309,-79.8057098386346,
-79.2446069498474),.UNSPECIFIED.);
#2056=B_SPLINE_CURVE_WITH_KNOTS('',3,(#23247,#23248,#23249,#23250,#23251,
#23252,#23253,#23254,#23255,#23256,#23257,#23258,#23259,#23260,#23261,#23262,
#23263,#23264,#23265,#23266,#23267,#23268),.UNSPECIFIED.,.F.,.F.,(4,3,3,
3,3,3,3,4),(-79.2446069498474,-78.8081384656517,-77.8105670926688,-76.8129957196858,
-75.8154243467029,-74.81785297372,-73.820281600737,-72.9614216426678),
 .UNSPECIFIED.);
#2057=B_SPLINE_CURVE_WITH_KNOTS('',3,(#23273,#23274,#23275,#23276,#23277,
#23278,#23279,#23280,#23281,#23282,#23283,#23284,#23285,#23286,#23287,#23288,
#23289,#23290,#23291,#23292,#23293,#23294),.UNSPECIFIED.,.F.,.F.,(4,3,3,
3,3,3,3,4),(70.4248606341475,70.8275674817882,71.8251388547712,72.8227102277541,
73.820281600737,74.81785297372,75.8154243467029,76.7080459413271),
 .UNSPECIFIED.);
#2058=B_SPLINE_CURVE_WITH_KNOTS('',3,(#23295,#23296,#23297,#23298,#23299,
#23300,#23301,#23302,#23303,#23304,#23305,#23306,#23307,#23308,#23309,#23310,
#23311,#23312,#23313,#23314,#23315,#23316,#23317,#23318,#23319),
 .UNSPECIFIED.,.F.,.F.,(4,3,3,3,3,3,3,3,4),(-72.9614216426678,-72.8227102277541,
-71.8251388547712,-70.8275674817882,-69.8299961088053,-68.8324247358224,
-67.8348533628394,-66.8372819898565,-66.6782363354882),.UNSPECIFIED.);
#2059=B_SPLINE_CURVE_WITH_KNOTS('',3,(#23324,#23325,#23326,#23327,#23328,
#23329,#23330,#23331,#23332,#23333,#23334,#23335,#23336,#23337,#23338,#23339,
#23340,#23341,#23342,#23343,#23344,#23345),.UNSPECIFIED.,.F.,.F.,(4,3,3,
3,3,3,3,4),(64.1416753269679,64.8421392438906,65.8397106168736,66.8372819898565,
67.8348533628394,68.8324247358224,69.8299961088053,70.4248606341475),
 .UNSPECIFIED.);
#2060=B_SPLINE_CURVE_WITH_KNOTS('',3,(#23346,#23347,#23348,#23349,#23350,
#23351,#23352,#23353,#23354,#23355,#23356,#23357,#23358,#23359,#23360,#23361,
#23362,#23363,#23364,#23365,#23366,#23367),.UNSPECIFIED.,.F.,.F.,(4,3,3,
3,3,3,3,4),(-66.6782363354882,-65.8397106168736,-64.8421392438907,-63.8445678709077,
-62.8469964979248,-61.8494251249419,-60.8518537519589,-60.3950510283086),
 .UNSPECIFIED.);
#2061=B_SPLINE_CURVE_WITH_KNOTS('',3,(#23372,#23373,#23374,#23375,#23376,
#23377,#23378,#23379,#23380,#23381,#23382,#23383,#23384,#23385,#23386,#23387,
#23388,#23389,#23390,#23391,#23392,#23393),.UNSPECIFIED.,.F.,.F.,(4,3,3,
3,3,3,3,4),(57.8584900197883,58.856711005993,59.854282378976,60.8518537519589,
61.8494251249418,62.8469964979247,63.8445678709077,64.1416753269679),
 .UNSPECIFIED.);
#2062=B_SPLINE_CURVE_WITH_KNOTS('',3,(#23394,#23395,#23396,#23397,#23398,
#23399,#23400,#23401,#23402,#23403,#23404,#23405,#23406,#23407,#23408,#23409,
#23410,#23411,#23412,#23413,#23414,#23415),.UNSPECIFIED.,.F.,.F.,(4,3,3,
3,3,3,3,4),(-60.3950510283086,-59.854282378976,-58.856711005993,-57.8591396330101,
-56.8615682600272,-55.8639968870442,-54.8664255140613,-54.111865721129),
 .UNSPECIFIED.);
#2063=B_SPLINE_CURVE_WITH_KNOTS('',3,(#23420,#23421,#23422,#23423,#23424,
#23425,#23426,#23427,#23428,#23429,#23430,#23431,#23432,#23433,#23434,#23435,
#23436,#23437,#23438,#23439,#23440,#23441),.UNSPECIFIED.,.F.,.F.,(4,3,3,
3,3,3,3,4),(51.5753047126087,51.8737113951125,52.8712827680954,53.8688541410784,
54.8664255140613,55.8639968870442,56.8615682600272,57.8584900197883),
 .UNSPECIFIED.);
#2064=B_SPLINE_CURVE_WITH_KNOTS('',3,(#23442,#23443,#23444,#23445,#23446,
#23447,#23448,#23449,#23450,#23451,#23452,#23453,#23454,#23455,#23456,#23457,
#23458,#23459,#23460,#23461,#23462,#23463,#23464,#23465,#23466),
 .UNSPECIFIED.,.F.,.F.,(4,3,3,3,3,3,3,3,4),(-54.111865721129,-53.8688541410784,
-52.8712827680954,-51.8737113951125,-50.8761400221296,-49.8785686491466,
-48.8809972761637,-47.8834259031808,-47.8286804139494),.UNSPECIFIED.);
#2065=B_SPLINE_CURVE_WITH_KNOTS('',3,(#23471,#23472,#23473,#23474,#23475,
#23476,#23477,#23478,#23479,#23480,#23481,#23482,#23483,#23484,#23485,#23486,
#23487,#23488,#23489,#23490,#23491,#23492),.UNSPECIFIED.,.F.,.F.,(4,3,3,
3,3,3,3,4),(45.2921194054291,45.8882831572149,46.8858545301978,47.8834259031808,
48.8809972761637,49.8785686491466,50.8761400221296,51.5753047126087),
 .UNSPECIFIED.);
#2066=B_SPLINE_CURVE_WITH_KNOTS('',3,(#23493,#23494,#23495,#23496,#23497,
#23498,#23499,#23500,#23501,#23502,#23503,#23504,#23505,#23506,#23507,#23508,
#23509,#23510,#23511,#23512,#23513,#23514),.UNSPECIFIED.,.F.,.F.,(4,3,3,
3,3,3,3,4),(-47.8286804139494,-46.8858545301979,-45.8882831572149,-44.890711784232,
-43.893140411249,-42.8955690382661,-41.8979976652832,-41.5454951067698),
 .UNSPECIFIED.);
#2067=B_SPLINE_CURVE_WITH_KNOTS('',3,(#23519,#23520,#23521,#23522,#23523,
#23524,#23525,#23526,#23527,#23528,#23529,#23530,#23531,#23532,#23533,#23534,
#23535,#23536,#23537,#23538,#23539,#23540),.UNSPECIFIED.,.F.,.F.,(4,3,3,
3,3,3,3,4),(39.0089340982495,39.9028549193173,40.9004262923002,41.8979976652832,
42.8955690382661,43.893140411249,44.890711784232,45.2921194054291),
 .UNSPECIFIED.);
#2068=B_SPLINE_CURVE_WITH_KNOTS('',3,(#23541,#23542,#23543,#23544,#23545,
#23546,#23547,#23548,#23549,#23550,#23551,#23552,#23553,#23554,#23555,#23556,
#23557,#23558,#23559,#23560,#23561,#23562),.UNSPECIFIED.,.F.,.F.,(4,3,3,
3,3,3,3,4),(-41.5454951067698,-40.9004262923003,-39.9028549193173,-38.9052835463344,
-37.9077121733515,-36.9101408003685,-35.9125694273856,-35.2623097995902),
 .UNSPECIFIED.);
#2069=B_SPLINE_CURVE_WITH_KNOTS('',3,(#23567,#23568,#23569,#23570,#23571,
#23572,#23573,#23574,#23575,#23576,#23577,#23578,#23579,#23580,#23581,#23582,
#23583,#23584,#23585,#23586,#23587,#23588,#23589,#23590,#23591),
 .UNSPECIFIED.,.F.,.F.,(4,3,3,3,3,3,3,3,4),(32.7257487910699,32.9198553084368,
33.9174266814197,34.9149980544027,35.9125694273856,36.9101408003685,37.9077121733514,
38.9052835463344,39.0089340982495),.UNSPECIFIED.);
#2070=B_SPLINE_CURVE_WITH_KNOTS('',3,(#23592,#23593,#23594,#23595,#23596,
#23597,#23598,#23599,#23600,#23601,#23602,#23603,#23604,#23605,#23606,#23607,
#23608,#23609,#23610,#23611,#23612,#23613),.UNSPECIFIED.,.F.,.F.,(4,3,3,
3,3,3,3,4),(-35.2623097995902,-34.9149980544027,-33.9174266814197,-32.9198553084368,
-31.9222839354538,-30.9247125624709,-29.927141189488,-28.9791244924106),
 .UNSPECIFIED.);
#2071=B_SPLINE_CURVE_WITH_KNOTS('',3,(#23618,#23619,#23620,#23621,#23622,
#23623,#23624,#23625,#23626,#23627,#23628,#23629,#23630,#23631,#23632,#23633,
#23634,#23635,#23636,#23637,#23638,#23639),.UNSPECIFIED.,.F.,.F.,(4,3,3,
3,3,3,3,4),(26.4425634838903,26.9344270705392,27.9319984435221,28.929569816505,
29.927141189488,30.9247125624709,31.9222839354538,32.7257487910699),
 .UNSPECIFIED.);
#2072=B_SPLINE_CURVE_WITH_KNOTS('',3,(#23640,#23641,#23642,#23643,#23644,
#23645,#23646,#23647,#23648,#23649,#23650,#23651,#23652,#23653,#23654,#23655,
#23656,#23657,#23658,#23659,#23660,#23661,#23662,#23663,#23664),
 .UNSPECIFIED.,.F.,.F.,(4,3,3,3,3,3,3,3,4),(-28.9791244924106,-28.929569816505,
-27.9319984435221,-26.9344270705392,-25.9368556975562,-24.9392843245733,
-23.9417129515904,-22.9441415786075,-22.695939185231),.UNSPECIFIED.);
#2073=B_SPLINE_CURVE_WITH_KNOTS('',3,(#23669,#23670,#23671,#23672,#23673,
#23674,#23675,#23676,#23677,#23678,#23679,#23680,#23681,#23682,#23683,#23684,
#23685,#23686,#23687,#23688,#23689,#23690),.UNSPECIFIED.,.F.,.F.,(4,3,3,
3,3,3,3,4),(20.1593781767107,20.9489988326416,21.9465702056245,22.9441415786074,
23.9417129515904,24.9392843245733,25.9368556975562,26.4425634838903),
 .UNSPECIFIED.);
#2074=B_SPLINE_CURVE_WITH_KNOTS('',3,(#23691,#23692,#23693,#23694,#23695,
#23696,#23697,#23698,#23699,#23700,#23701,#23702,#23703,#23704,#23705,#23706,
#23707,#23708,#23709,#23710,#23711,#23712),.UNSPECIFIED.,.F.,.F.,(4,3,3,
3,3,3,3,4),(-22.695939185231,-21.9465702056245,-20.9489988326416,-19.9514274596586,
-18.9538560866757,-17.9562847136928,-16.9587133407099,-16.4127538780514),
 .UNSPECIFIED.);
#2075=B_SPLINE_CURVE_WITH_KNOTS('',3,(#23717,#23718,#23719,#23720,#23721,
#23722,#23723,#23724,#23725,#23726,#23727,#23728,#23729,#23730,#23731,#23732,
#23733,#23734,#23735,#23736,#23737,#23738,#23739,#23740,#23741),
 .UNSPECIFIED.,.F.,.F.,(4,3,3,3,3,3,3,3,4),(13.8761928695311,13.9659992217611,
14.963570594744,15.9611419677269,16.9587133407099,17.9562847136928,18.9538560866757,
19.9514274596586,20.1593781767107),.UNSPECIFIED.);
#2076=B_SPLINE_CURVE_WITH_KNOTS('',3,(#23742,#23743,#23744,#23745,#23746,
#23747,#23748,#23749,#23750,#23751,#23752,#23753,#23754,#23755,#23756,#23757,
#23758,#23759,#23760,#23761,#23762,#23763),.UNSPECIFIED.,.F.,.F.,(4,3,3,
3,3,3,3,4),(-16.4127538780514,-15.9611419677269,-14.963570594744,-13.9659992217611,
-12.9684278487781,-11.9708564757952,-10.9732851028123,-10.1295685708718),
 .UNSPECIFIED.);
#2077=B_SPLINE_CURVE_WITH_KNOTS('',3,(#23769,#23770,#23771,#23772,#23773,
#23774,#23775,#23776,#23777,#23778,#23779,#23780,#23781),.UNSPECIFIED.,
 .F.,.F.,(4,3,3,3,4),(-3.84638326369226,-2.9927141189488,-1.99514274596587,
-0.997571372982931,0.),.UNSPECIFIED.);
#2078=B_SPLINE_CURVE_WITH_KNOTS('',3,(#23784,#23785,#23786,#23787,#23788,
#23789,#23790,#23791,#23792,#23793,#23794,#23795,#23796,#23797,#23798,#23799,
#23800,#23801,#23802),.UNSPECIFIED.,.F.,.F.,(4,3,3,3,3,3,4),(2.01461286527445,
2.9927141189488,3.99028549193173,4.98785686491467,5.9854282378976,6.98299961088053,
7.59300756235155),.UNSPECIFIED.);
#2079=B_SPLINE_CURVE_WITH_KNOTS('',3,(#23808,#23809,#23810,#23811,#23812,
#23813,#23814),.UNSPECIFIED.,.F.,.F.,(4,1,1,1,4),(91.106186954104,91.6672898428913,
92.6648612158742,93.6624325888571,94.6600039618401),.UNSPECIFIED.);
#2080=B_SPLINE_CURVE_WITH_KNOTS('',3,(#23817,#23818,#23819,#23820,#23821,
#23822,#23823,#23824),.UNSPECIFIED.,.F.,.F.,(4,1,1,1,1,4),(91.106186954104,
91.2111367324627,92.2087081054457,93.2062794784286,94.2038508514115,95.1819521050859),
 .UNSPECIFIED.);
#2081=B_SPLINE_CURVE_WITH_KNOTS('',3,(#23829,#23830,#23831,#23832,#23833,
#23834,#23835,#23836,#23837,#23838),.UNSPECIFIED.,.F.,.F.,(4,1,1,1,1,1,
1,4),(84.8230016469244,85.6818616049937,86.6794329779766,87.6770043509595,
88.6745757239425,89.6721470969254,90.6697184699083,91.106186954104),
 .UNSPECIFIED.);
#2082=B_SPLINE_CURVE_WITH_KNOTS('',3,(#23839,#23840,#23841,#23842,#23843,
#23844,#23845,#23846,#23847,#23848),.UNSPECIFIED.,.F.,.F.,(4,1,1,1,1,1,
1,4),(84.8230016469244,85.2257084945651,86.2232798675481,87.220851240531,
88.2184226135139,89.2159939864969,90.2135653594798,91.106186954104),
 .UNSPECIFIED.);
#2083=B_SPLINE_CURVE_WITH_KNOTS('',3,(#23853,#23854,#23855,#23856,#23857,
#23858,#23859,#23860,#23861,#23862,#23863),.UNSPECIFIED.,.F.,.F.,(4,1,1,
1,1,1,1,1,4),(78.5398163397448,78.6988619941132,79.6964333670961,80.694004740079,
81.691576113062,82.6891474860449,83.6867188590278,84.6842902320108,84.8230016469244),
 .UNSPECIFIED.);
#2084=B_SPLINE_CURVE_WITH_KNOTS('',3,(#23864,#23865,#23866,#23867,#23868,
#23869,#23870,#23871,#23872,#23873),.UNSPECIFIED.,.F.,.F.,(4,1,1,1,1,1,
1,4),(78.5398163397448,79.2402802566675,80.2378516296505,81.2354230026334,
82.2329943756163,83.2305657485993,84.2281371215822,84.8230016469244),
 .UNSPECIFIED.);
#2085=B_SPLINE_CURVE_WITH_KNOTS('',3,(#23878,#23879,#23880,#23881,#23882,
#23883,#23884,#23885,#23886,#23887),.UNSPECIFIED.,.F.,.F.,(4,1,1,1,1,1,
1,4),(72.2566310325652,72.7134337562156,73.7110051291985,74.7085765021814,
75.7061478751643,76.7037192481473,77.7012906211302,78.5398163397448),
 .UNSPECIFIED.);
#2086=B_SPLINE_CURVE_WITH_KNOTS('',3,(#23888,#23889,#23890,#23891,#23892,
#23893,#23894,#23895,#23896,#23897,#23898),.UNSPECIFIED.,.F.,.F.,(4,1,1,
1,1,1,1,1,4),(72.2566310325652,72.257280645787,73.2548520187699,74.2524233917529,
75.2499947647358,76.2475661377187,77.2451375107017,78.2427088836846,78.5398163397448),
 .UNSPECIFIED.);
#2087=B_SPLINE_CURVE_WITH_KNOTS('',3,(#23903,#23904,#23905,#23906,#23907,
#23908,#23909,#23910,#23911,#23912),.UNSPECIFIED.,.F.,.F.,(4,1,1,1,1,1,
1,4),(65.9734457253856,66.728005518318,67.7255768913009,68.7231482642838,
69.7207196372668,70.7182910102497,71.7158623832326,72.2566310325652),
 .UNSPECIFIED.);
#2088=B_SPLINE_CURVE_WITH_KNOTS('',3,(#23913,#23914,#23915,#23916,#23917,
#23918,#23919,#23920,#23921,#23922),.UNSPECIFIED.,.F.,.F.,(4,1,1,1,1,1,
1,4),(65.9734457253856,66.2718524078894,67.2694237808723,68.2669951538553,
69.2645665268382,70.2621378998211,71.2597092728041,72.2566310325652),
 .UNSPECIFIED.);
#2089=B_SPLINE_CURVE_WITH_KNOTS('',3,(#23927,#23928,#23929,#23930,#23931,
#23932,#23933,#23934,#23935,#23936,#23937),.UNSPECIFIED.,.F.,.F.,(4,1,1,
1,1,1,1,1,4),(59.690260418206,59.7450059074374,60.7425772804204,61.7401486534033,
62.7377200263862,63.7352913993692,64.7328627723521,65.730434145335,65.9734457253856),
 .UNSPECIFIED.);
#2090=B_SPLINE_CURVE_WITH_KNOTS('',3,(#23938,#23939,#23940,#23941,#23942,
#23943,#23944,#23945,#23946,#23947),.UNSPECIFIED.,.F.,.F.,(4,1,1,1,1,1,
1,4),(59.690260418206,60.2864241699918,61.2839955429747,62.2815669159577,
63.2791382889406,64.2767096619235,65.2742810349065,65.9734457253856),
 .UNSPECIFIED.);
#2091=B_SPLINE_CURVE_WITH_KNOTS('',3,(#23952,#23953,#23954,#23955,#23956,
#23957,#23958,#23959,#23960,#23961),.UNSPECIFIED.,.F.,.F.,(4,1,1,1,1,1,
1,4),(53.4070751110264,53.7595776695398,54.7571490425228,55.7547204155057,
56.7522917884886,57.7498631614716,58.7474345344545,59.690260418206),
 .UNSPECIFIED.);
#2092=B_SPLINE_CURVE_WITH_KNOTS('',3,(#23962,#23963,#23964,#23965,#23966,
#23967,#23968,#23969,#23970,#23971),.UNSPECIFIED.,.F.,.F.,(4,1,1,1,1,1,
1,4),(53.4070751110264,54.3009959320942,55.2985673050771,56.2961386780601,
57.293710051043,58.2912814240259,59.2888527970089,59.690260418206),
 .UNSPECIFIED.);
#2093=B_SPLINE_CURVE_WITH_KNOTS('',3,(#23976,#23977,#23978,#23979,#23980,
#23981,#23982,#23983,#23984,#23985),.UNSPECIFIED.,.F.,.F.,(4,1,1,1,1,1,
1,4),(47.1238898038468,47.7741494316422,48.7717208046252,49.7692921776081,
50.766863550591,51.764434923574,52.7620062965569,53.4070751110264),
 .UNSPECIFIED.);
#2094=B_SPLINE_CURVE_WITH_KNOTS('',3,(#23986,#23987,#23988,#23989,#23990,
#23991,#23992,#23993,#23994,#23995,#23996),.UNSPECIFIED.,.F.,.F.,(4,1,1,
1,1,1,1,1,4),(47.1238898038468,47.3179963212137,48.3155676941966,49.3131390671795,
50.3107104401625,51.3082818131454,52.3058531861283,53.3034245591113,53.4070751110264),
 .UNSPECIFIED.);
#2095=B_SPLINE_CURVE_WITH_KNOTS('',3,(#24001,#24002,#24003,#24004,#24005,
#24006,#24007,#24008,#24009,#24010),.UNSPECIFIED.,.F.,.F.,(4,1,1,1,1,1,
1,4),(40.8407044966673,41.7887211937446,42.7862925667276,43.7838639397105,
44.7814353126934,45.7790066856764,46.7765780586593,47.1238898038468),
 .UNSPECIFIED.);
#2096=B_SPLINE_CURVE_WITH_KNOTS('',3,(#24011,#24012,#24013,#24014,#24015,
#24016,#24017,#24018,#24019,#24020),.UNSPECIFIED.,.F.,.F.,(4,1,1,1,1,1,
1,4),(40.8407044966673,41.3325680833161,42.330139456299,43.3277108292819,
44.3252822022649,45.3228535752478,46.3204249482307,47.1238898038468),
 .UNSPECIFIED.);
#2097=B_SPLINE_CURVE_WITH_KNOTS('',3,(#24025,#24026,#24027,#24028,#24029,
#24030,#24031,#24032,#24033,#24034,#24035),.UNSPECIFIED.,.F.,.F.,(4,1,1,
1,1,1,1,1,4),(34.5575191894876,34.8057215828641,35.803292955847,36.80086432883,
37.7984357018129,38.7960070747958,39.7935784477788,40.7911498207617,40.8407044966673),
 .UNSPECIFIED.);
#2098=B_SPLINE_CURVE_WITH_KNOTS('',3,(#24036,#24037,#24038,#24039,#24040,
#24041,#24042,#24043,#24044,#24045),.UNSPECIFIED.,.F.,.F.,(4,1,1,1,1,1,
1,4),(34.5575191894876,35.3471398454185,36.3447112184014,37.3422825913843,
38.3398539643673,39.3374253373502,40.3349967103331,40.8407044966673),
 .UNSPECIFIED.);
#2099=B_SPLINE_CURVE_WITH_KNOTS('',3,(#24050,#24051,#24052,#24053,#24054,
#24055,#24056,#24057,#24058,#24059),.UNSPECIFIED.,.F.,.F.,(4,1,1,1,1,1,
1,4),(28.2743338823081,28.8202933449665,29.8178647179494,30.8154360909324,
31.8130074639153,32.8105788368982,33.8081502098812,34.5575191894876),
 .UNSPECIFIED.);
#2100=B_SPLINE_CURVE_WITH_KNOTS('',3,(#24060,#24061,#24062,#24063,#24064,
#24065,#24066,#24067,#24068,#24069,#24070),.UNSPECIFIED.,.F.,.F.,(4,1,1,
1,1,1,1,1,4),(28.2743338823081,28.364140234538,29.3617116075209,30.3592829805038,
31.3568543534868,32.3544257264697,33.3519970994526,34.3495684724355,34.5575191894876),
 .UNSPECIFIED.);
#2101=B_SPLINE_CURVE_WITH_KNOTS('',3,(#24075,#24076,#24077,#24078,#24079,
#24080,#24081,#24082,#24083,#24084),.UNSPECIFIED.,.F.,.F.,(4,1,1,1,1,1,
1,4),(21.9911485751285,22.8348651070689,23.8324364800518,24.8300078530348,
25.8275792260177,26.8251505990006,27.8227219719836,28.2743338823081),
 .UNSPECIFIED.);
#2102=B_SPLINE_CURVE_WITH_KNOTS('',3,(#24085,#24086,#24087,#24088,#24089,
#24090,#24091,#24092,#24093,#24094),.UNSPECIFIED.,.F.,.F.,(4,1,1,1,1,1,
1,4),(21.9911485751285,22.3787119966404,23.3762833696233,24.3738547426062,
25.3714261155892,26.3689974885721,27.366568861555,28.2743338823081),
 .UNSPECIFIED.);
#2103=B_SPLINE_CURVE_WITH_KNOTS('',3,(#24100,#24101,#24102,#24103,#24104),
 .UNSPECIFIED.,.F.,.F.,(4,1,4),(14.3981410127769,15.3957123857598,15.7079632679489),
 .UNSPECIFIED.);
#2104=B_SPLINE_CURVE_WITH_KNOTS('',3,(#24107,#24108,#24109,#24110,#24111),
 .UNSPECIFIED.,.F.,.F.,(4,1,4),(13.8761928695311,14.8542941232054,15.7079632679489),
 .UNSPECIFIED.);
#2105=B_SPLINE_CURVE_WITH_KNOTS('',3,(#24117,#24118,#24119,#24120),
 .UNSPECIFIED.,.F.,.F.,(4,4),(114.40689867021,115.117908020989),
 .UNSPECIFIED.);
#2106=B_SPLINE_CURVE_WITH_KNOTS('',3,(#24128,#24129,#24130,#24131,#24132,
#24133,#24134,#24135,#24136,#24137),.UNSPECIFIED.,.F.,.F.,(4,3,3,4),(-113.097335529232,
-112.140720744584,-111.148324985783,-110.666752226423),.UNSPECIFIED.);
#2107=B_SPLINE_CURVE_WITH_KNOTS('',3,(#24142,#24143,#24144,#24145,#24146,
#24147,#24148,#24149,#24150,#24151,#24152,#24153,#24154,#24155,#24156,#24157,
#24158,#24159,#24160,#24161,#24162,#24163,#24164,#24165,#24166),
 .UNSPECIFIED.,.F.,.F.,(4,3,3,3,3,3,3,3,4),(108.12371336303,108.171137709378,
109.16353346818,110.155929226981,111.148324985783,112.140720744584,113.133116503386,
114.125512262188,114.40689867021),.UNSPECIFIED.);
#2108=B_SPLINE_CURVE_WITH_KNOTS('',3,(#24167,#24168,#24169,#24170,#24171,
#24172,#24173,#24174,#24175,#24176,#24177,#24178,#24179,#24180,#24181,#24182,
#24183,#24184,#24185,#24186,#24187,#24188),.UNSPECIFIED.,.F.,.F.,(4,3,3,
3,3,3,3,4),(-110.666752226423,-110.155929226981,-109.16353346818,-108.171137709378,
-107.178741950576,-106.186346191775,-105.193950432973,-104.383566919243),
 .UNSPECIFIED.);
#2109=B_SPLINE_CURVE_WITH_KNOTS('',3,(#24193,#24194,#24195,#24196,#24197,
#24198,#24199,#24200,#24201,#24202,#24203,#24204,#24205,#24206,#24207,#24208,
#24209,#24210,#24211,#24212,#24213,#24214),.UNSPECIFIED.,.F.,.F.,(4,3,3,
3,3,3,3,4),(101.84052805585,102.216763156568,103.20915891537,104.201554674171,
105.193950432973,106.186346191775,107.178741950576,108.12371336303),
 .UNSPECIFIED.);
#2110=B_SPLINE_CURVE_WITH_KNOTS('',3,(#24215,#24216,#24217,#24218,#24219,
#24220,#24221,#24222,#24223,#24224,#24225,#24226,#24227,#24228,#24229,#24230,
#24231,#24232,#24233,#24234,#24235,#24236,#24237,#24238,#24239),
 .UNSPECIFIED.,.F.,.F.,(4,3,3,3,3,3,3,3,4),(-104.383566919243,-104.201554674171,
-103.20915891537,-102.216763156568,-101.224367397767,-100.231971638965,
-99.2395758801633,-98.2471801213616,-98.1003816120635),.UNSPECIFIED.);
#2111=B_SPLINE_CURVE_WITH_KNOTS('',3,(#24244,#24245,#24246,#24247,#24248,
#24249,#24250,#24251,#24252,#24253,#24254,#24255,#24256,#24257,#24258,#24259,
#24260,#24261,#24262,#24263,#24264,#24265),.UNSPECIFIED.,.F.,.F.,(4,3,3,
3,3,3,3,4),(95.5573427486709,96.2623886037584,97.25478436256,98.2471801213616,
99.2395758801633,100.231971638965,101.224367397767,101.84052805585),
 .UNSPECIFIED.);
#2112=B_SPLINE_CURVE_WITH_KNOTS('',3,(#24266,#24267,#24268,#24269,#24270,
#24271,#24272,#24273,#24274,#24275,#24276,#24277,#24278,#24279,#24280,#24281,
#24282,#24283,#24284,#24285,#24286,#24287),.UNSPECIFIED.,.F.,.F.,(4,3,3,
3,3,3,3,4),(-98.1003816120635,-97.25478436256,-96.2623886037584,-95.2699928449567,
-94.2775970861551,-93.2852013273535,-92.2928055685519,-91.8171963048839),
 .UNSPECIFIED.);
#2113=B_SPLINE_CURVE_WITH_KNOTS('',3,(#24292,#24293,#24294,#24295,#24296,
#24297,#24298,#24299,#24300,#24301,#24302,#24303,#24304,#24305,#24306,#24307,
#24308,#24309,#24310,#24311,#24312,#24313,#24314,#24315,#24316),
 .UNSPECIFIED.,.F.,.F.,(4,3,3,3,3,3,3,3,4),(89.2741574414912,89.3156182921469,
90.3080140509486,91.3004098097502,92.2928055685518,93.2852013273535,94.2775970861551,
95.2699928449567,95.5573427486709),.UNSPECIFIED.);
#2114=B_SPLINE_CURVE_WITH_KNOTS('',3,(#24317,#24318,#24319,#24320,#24321,
#24322,#24323,#24324,#24325,#24326,#24327,#24328,#24329,#24330,#24331,#24332,
#24333,#24334,#24335,#24336,#24337,#24338),.UNSPECIFIED.,.F.,.F.,(4,3,3,
3,3,3,3,4),(-91.8171963048839,-91.3004098097502,-90.3080140509486,-89.315618292147,
-88.3232225333453,-87.3308267745437,-86.338431015742,-85.5340109977043),
 .UNSPECIFIED.);
#2115=B_SPLINE_CURVE_WITH_KNOTS('',3,(#24343,#24344,#24345,#24346,#24347,
#24348,#24349,#24350,#24351,#24352,#24353,#24354,#24355,#24356,#24357,#24358,
#24359,#24360,#24361,#24362,#24363,#24364),.UNSPECIFIED.,.F.,.F.,(4,3,3,
3,3,3,3,4),(82.9909721343117,83.3612437393372,84.3536394981388,85.3460352569404,
86.338431015742,87.3308267745437,88.3232225333453,89.2741574414912),
 .UNSPECIFIED.);
#2116=B_SPLINE_CURVE_WITH_KNOTS('',3,(#24365,#24366,#24367,#24368,#24369,
#24370,#24371,#24372,#24373,#24374,#24375,#24376,#24377,#24378,#24379,#24380,
#24381,#24382,#24383,#24384,#24385,#24386,#24387,#24388,#24389),
 .UNSPECIFIED.,.F.,.F.,(4,3,3,3,3,3,3,3,4),(-85.5340109977043,-85.3460352569404,
-84.3536394981388,-83.3612437393372,-82.3688479805355,-81.3764522217339,
-80.3840564629323,-79.3916607041306,-79.2508256905247),.UNSPECIFIED.);
#2117=B_SPLINE_CURVE_WITH_KNOTS('',3,(#24394,#24395,#24396,#24397,#24398,
#24399,#24400,#24401,#24402,#24403,#24404,#24405,#24406,#24407,#24408,#24409,
#24410,#24411,#24412,#24413,#24414,#24415),.UNSPECIFIED.,.F.,.F.,(4,3,3,
3,3,3,3,4),(76.7077868271321,77.4068691865273,78.399264945329,79.3916607041306,
80.3840564629322,81.3764522217339,82.3688479805355,82.9909721343117),
 .UNSPECIFIED.);
#2118=B_SPLINE_CURVE_WITH_KNOTS('',3,(#24416,#24417,#24418,#24419,#24420,
#24421,#24422,#24423,#24424,#24425,#24426,#24427,#24428,#24429,#24430,#24431,
#24432,#24433,#24434,#24435,#24436,#24437),.UNSPECIFIED.,.F.,.F.,(4,3,3,
3,3,3,3,4),(-79.2508256905247,-78.399264945329,-77.4068691865274,-76.4144734277257,
-75.4220776689241,-74.4296819101224,-73.4372861513208,-72.9676403833451),
 .UNSPECIFIED.);
#2119=B_SPLINE_CURVE_WITH_KNOTS('',3,(#24442,#24443,#24444,#24445,#24446,
#24447,#24448,#24449,#24450,#24451,#24452,#24453,#24454,#24455,#24456,#24457,
#24458,#24459,#24460,#24461,#24462,#24463,#24464,#24465,#24466),
 .UNSPECIFIED.,.F.,.F.,(4,3,3,3,3,3,3,3,4),(70.4246015199525,70.4600988749159,
71.4524946337175,72.4448903925192,73.4372861513208,74.4296819101224,75.4220776689241,
76.4144734277257,76.7077868271321),.UNSPECIFIED.);
#2120=B_SPLINE_CURVE_WITH_KNOTS('',3,(#24467,#24468,#24469,#24470,#24471,
#24472,#24473,#24474,#24475,#24476,#24477,#24478,#24479,#24480,#24481,#24482,
#24483,#24484,#24485,#24486,#24487,#24488),.UNSPECIFIED.,.F.,.F.,(4,3,3,
3,3,3,3,4),(-72.9676403833451,-72.4448903925192,-71.4524946337175,-70.4600988749159,
-69.4677031161143,-68.4753073573127,-67.482911598511,-66.6844550761655),
 .UNSPECIFIED.);
#2121=B_SPLINE_CURVE_WITH_KNOTS('',3,(#24493,#24494,#24495,#24496,#24497,
#24498,#24499,#24500,#24501,#24502,#24503,#24504,#24505,#24506,#24507,#24508,
#24509,#24510,#24511,#24512,#24513,#24514),.UNSPECIFIED.,.F.,.F.,(4,3,3,
3,3,3,3,4),(64.1414162127729,64.5057243221061,65.4981200809078,66.4905158397094,
67.482911598511,68.4753073573126,69.4677031161143,70.4246015199525),
 .UNSPECIFIED.);
#2122=B_SPLINE_CURVE_WITH_KNOTS('',3,(#24515,#24516,#24517,#24518,#24519,
#24520,#24521,#24522,#24523,#24524,#24525,#24526,#24527,#24528,#24529,#24530,
#24531,#24532,#24533,#24534,#24535,#24536,#24537,#24538,#24539),
 .UNSPECIFIED.,.F.,.F.,(4,3,3,3,3,3,3,3,4),(-66.6844550761655,-66.4905158397094,
-65.4981200809078,-64.5057243221061,-63.5133285633045,-62.5209328045029,
-61.5285370457012,-60.5361412868996,-60.4012697689859),.UNSPECIFIED.);
#2123=B_SPLINE_CURVE_WITH_KNOTS('',3,(#24544,#24545,#24546,#24547,#24548,
#24549,#24550,#24551,#24552,#24553,#24554,#24555,#24556,#24557,#24558,#24559,
#24560,#24561,#24562,#24563,#24564,#24565),.UNSPECIFIED.,.F.,.F.,(4,3,3,
3,3,3,3,4),(57.8582309055933,58.5513497692963,59.543745528098,60.5361412868996,
61.5285370457012,62.5209328045029,63.5133285633045,64.1414162127729),
 .UNSPECIFIED.);
#2124=B_SPLINE_CURVE_WITH_KNOTS('',3,(#24566,#24567,#24568,#24569,#24570,
#24571,#24572,#24573,#24574,#24575,#24576,#24577,#24578,#24579,#24580,#24581,
#24582,#24583,#24584,#24585,#24586,#24587),.UNSPECIFIED.,.F.,.F.,(4,3,3,
3,3,3,3,4),(-60.4012697689859,-59.543745528098,-58.5513497692964,-57.5589540104947,
-56.5665582516931,-55.5741624928914,-54.5817667340898,-54.1180844618063),
 .UNSPECIFIED.);
#2125=B_SPLINE_CURVE_WITH_KNOTS('',3,(#24592,#24593,#24594,#24595,#24596,
#24597,#24598,#24599,#24600,#24601,#24602,#24603,#24604,#24605,#24606,#24607,
#24608,#24609,#24610,#24611,#24612,#24613,#24614,#24615,#24616),
 .UNSPECIFIED.,.F.,.F.,(4,3,3,3,3,3,3,3,4),(51.5750455984137,51.6045794576849,
52.5969752164865,53.5893709752882,54.5817667340898,55.5741624928914,56.5665582516931,
57.5589540104947,57.8582309055933),.UNSPECIFIED.);
#2126=B_SPLINE_CURVE_WITH_KNOTS('',3,(#24617,#24618,#24619,#24620,#24621,
#24622,#24623,#24624,#24625,#24626,#24627,#24628,#24629,#24630,#24631,#24632,
#24633,#24634,#24635,#24636,#24637,#24638),.UNSPECIFIED.,.F.,.F.,(4,3,3,
3,3,3,3,4),(-54.1180844618063,-53.5893709752882,-52.5969752164865,-51.6045794576849,
-50.6121836988833,-49.6197879400816,-48.62739218128,-47.8348991546267),
 .UNSPECIFIED.);
#2127=B_SPLINE_CURVE_WITH_KNOTS('',3,(#24643,#24644,#24645,#24646,#24647,
#24648,#24649,#24650,#24651,#24652,#24653,#24654,#24655,#24656,#24657,#24658,
#24659,#24660,#24661,#24662,#24663,#24664),.UNSPECIFIED.,.F.,.F.,(4,3,3,
3,3,3,3,4),(45.2918602912341,45.6502049048751,46.6426006636767,47.6349964224784,
48.62739218128,49.6197879400816,50.6121836988833,51.5750455984137),
 .UNSPECIFIED.);
#2128=B_SPLINE_CURVE_WITH_KNOTS('',3,(#24665,#24666,#24667,#24668,#24669,
#24670,#24671,#24672,#24673,#24674,#24675,#24676,#24677,#24678,#24679,#24680,
#24681,#24682,#24683,#24684,#24685,#24686,#24687,#24688,#24689),
 .UNSPECIFIED.,.F.,.F.,(4,3,3,3,3,3,3,3,4),(-47.8348991546267,-47.6349964224784,
-46.6426006636767,-45.6502049048751,-44.6578091460735,-43.6654133872718,
-42.6730176284702,-41.6806218696686,-41.5517138474472),.UNSPECIFIED.);
#2129=B_SPLINE_CURVE_WITH_KNOTS('',3,(#24694,#24695,#24696,#24697,#24698,
#24699,#24700,#24701,#24702,#24703,#24704,#24705,#24706,#24707,#24708,#24709,
#24710,#24711,#24712,#24713,#24714,#24715),.UNSPECIFIED.,.F.,.F.,(4,3,3,
3,3,3,3,4),(39.0086749840545,39.6958303520653,40.6882261108669,41.6806218696686,
42.6730176284702,43.6654133872718,44.6578091460735,45.2918602912341),
 .UNSPECIFIED.);
#2130=B_SPLINE_CURVE_WITH_KNOTS('',3,(#24716,#24717,#24718,#24719,#24720,
#24721,#24722,#24723,#24724,#24725,#24726,#24727,#24728,#24729,#24730,#24731,
#24732,#24733,#24734,#24735,#24736,#24737),.UNSPECIFIED.,.F.,.F.,(4,3,3,
3,3,3,3,4),(-41.5517138474472,-40.6882261108669,-39.6958303520653,-38.7034345932637,
-37.711038834462,-36.7186430756604,-35.7262473168588,-35.2685285402675),
 .UNSPECIFIED.);
#2131=B_SPLINE_CURVE_WITH_KNOTS('',3,(#24742,#24743,#24744,#24745,#24746,
#24747,#24748,#24749,#24750,#24751,#24752,#24753,#24754,#24755,#24756,#24757,
#24758,#24759,#24760,#24761,#24762,#24763,#24764,#24765,#24766),
 .UNSPECIFIED.,.F.,.F.,(4,3,3,3,3,3,3,3,4),(32.725489676875,32.7490600404539,
33.7414557992555,34.7338515580571,35.7262473168588,36.7186430756604,37.711038834462,
38.7034345932637,39.0086749840545),.UNSPECIFIED.);
#2132=B_SPLINE_CURVE_WITH_KNOTS('',3,(#24767,#24768,#24769,#24770,#24771,
#24772,#24773,#24774,#24775,#24776,#24777,#24778,#24779,#24780,#24781,#24782,
#24783,#24784,#24785,#24786,#24787,#24788),.UNSPECIFIED.,.F.,.F.,(4,3,3,
3,3,3,3,4),(-35.2685285402675,-34.7338515580572,-33.7414557992555,-32.7490600404539,
-31.7566642816523,-30.7642685228506,-29.771872764049,-28.985343233088),
 .UNSPECIFIED.);
#2133=B_SPLINE_CURVE_WITH_KNOTS('',3,(#24793,#24794,#24795,#24796,#24797,
#24798,#24799,#24800,#24801,#24802,#24803,#24804,#24805,#24806,#24807,#24808,
#24809,#24810,#24811,#24812,#24813,#24814),.UNSPECIFIED.,.F.,.F.,(4,3,3,
3,3,3,3,4),(26.4423043696953,26.7946854876441,27.7870812464457,28.7794770052473,
29.771872764049,30.7642685228506,31.7566642816522,32.725489676875),
 .UNSPECIFIED.);
#2134=B_SPLINE_CURVE_WITH_KNOTS('',3,(#24815,#24816,#24817,#24818,#24819,
#24820,#24821,#24822,#24823,#24824,#24825,#24826,#24827,#24828,#24829,#24830,
#24831,#24832,#24833,#24834,#24835,#24836,#24837,#24838,#24839),
 .UNSPECIFIED.,.F.,.F.,(4,3,3,3,3,3,3,3,4),(-28.985343233088,-28.7794770052474,
-27.7870812464457,-26.7946854876441,-25.8022897288425,-24.8098939700408,
-23.8174982112392,-22.8251024524376,-22.7021579259084),.UNSPECIFIED.);
#2135=B_SPLINE_CURVE_WITH_KNOTS('',3,(#24844,#24845,#24846,#24847,#24848,
#24849,#24850,#24851,#24852,#24853,#24854,#24855,#24856,#24857,#24858,#24859,
#24860,#24861,#24862,#24863,#24864,#24865),.UNSPECIFIED.,.F.,.F.,(4,3,3,
3,3,3,3,4),(20.1591190625158,20.8403109348343,21.8327066936359,22.8251024524376,
23.8174982112392,24.8098939700408,25.8022897288424,26.4423043696953),
 .UNSPECIFIED.);
#2136=B_SPLINE_CURVE_WITH_KNOTS('',3,(#24866,#24867,#24868,#24869,#24870,
#24871,#24872,#24873,#24874,#24875,#24876,#24877,#24878,#24879,#24880,#24881,
#24882,#24883,#24884,#24885,#24886,#24887),.UNSPECIFIED.,.F.,.F.,(4,3,3,
3,3,3,3,4),(-22.7021579259084,-21.8327066936359,-20.8403109348343,-19.8479151760327,
-18.855519417231,-17.8631236584294,-16.8707278996278,-16.4189726187288),
 .UNSPECIFIED.);
#2137=B_SPLINE_CURVE_WITH_KNOTS('',3,(#24892,#24893,#24894,#24895,#24896,
#24897,#24898,#24899,#24900,#24901,#24902,#24903,#24904,#24905,#24906,#24907,
#24908,#24909,#24910,#24911,#24912,#24913,#24914,#24915,#24916),
 .UNSPECIFIED.,.F.,.F.,(4,3,3,3,3,3,3,3,4),(13.8759337553361,13.8935406232229,
14.8859363820245,15.8783321408261,16.8707278996278,17.8631236584294,18.855519417231,
19.8479151760327,20.1591190625158),.UNSPECIFIED.);
#2138=B_SPLINE_CURVE_WITH_KNOTS('',3,(#24917,#24918,#24919,#24920,#24921,
#24922,#24923,#24924,#24925,#24926,#24927,#24928,#24929,#24930,#24931,#24932,
#24933,#24934,#24935,#24936,#24937,#24938),.UNSPECIFIED.,.F.,.F.,(4,3,3,
3,3,3,3,4),(-16.4189726187288,-15.8783321408261,-14.8859363820245,-13.8935406232229,
-12.9011448644212,-11.9087491056196,-10.916353346818,-10.1357873115492),
 .UNSPECIFIED.);
#2139=B_SPLINE_CURVE_WITH_KNOTS('',3,(#24944,#24945,#24946,#24947,#24948,
#24949,#24950,#24951,#24952,#24953,#24954,#24955,#24956),.UNSPECIFIED.,
 .F.,.F.,(4,3,3,3,4),(-3.85260200436961,-2.9771872764049,-1.98479151760327,
-0.992395758801633,0.),.UNSPECIFIED.);
#2140=B_SPLINE_CURVE_WITH_KNOTS('',3,(#24959,#24960,#24961,#24962,#24963,
#24964,#24965,#24966,#24967,#24968,#24969,#24970,#24971,#24972,#24973,#24974,
#24975,#24976,#24977),.UNSPECIFIED.,.F.,.F.,(4,3,3,3,3,3,4),(2.0205724917569,
2.9771872764049,3.96958303520653,4.96197879400816,5.9543745528098,6.94677031161143,
7.59274844815659),.UNSPECIFIED.);
#2141=B_SPLINE_CURVE_WITH_KNOTS('',3,(#24983,#24984,#24985,#24986,#24987,
#24988,#24989,#24990),.UNSPECIFIED.,.F.,.F.,(4,1,1,1,1,4),(122.522113490002,
123.003686249362,123.996082008164,124.988477766965,125.980873525767,126.973269284569),
 .UNSPECIFIED.);
#2142=B_SPLINE_CURVE_WITH_KNOTS('',3,(#24993,#24994,#24995,#24996,#24997,
#24998,#24999,#25000,#25001),.UNSPECIFIED.,.F.,.F.,(4,1,1,1,1,1,4),(122.522113490002,
122.56953783635,123.561933595151,124.554329353953,125.546725112755,126.539120871556,
127.495735656204),.UNSPECIFIED.);
#2143=B_SPLINE_CURVE_WITH_KNOTS('',3,(#25006,#25007,#25008,#25009,#25010,
#25011,#25012,#25013,#25014,#25015),.UNSPECIFIED.,.F.,.F.,(4,1,1,1,1,1,
1,4),(116.238928182822,117.049311696552,118.041707455354,119.034103214156,
120.026498972957,121.018894731759,122.01129049056,122.522113490002),
 .UNSPECIFIED.);
#2144=B_SPLINE_CURVE_WITH_KNOTS('',3,(#25016,#25017,#25018,#25019,#25020,
#25021,#25022,#25023,#25024,#25025),.UNSPECIFIED.,.F.,.F.,(4,1,1,1,1,1,
1,4),(116.238928182822,116.61516328354,117.607559042342,118.599954801143,
119.592350559945,120.584746318746,121.577142077548,122.522113490002),
 .UNSPECIFIED.);
#2145=B_SPLINE_CURVE_WITH_KNOTS('',3,(#25030,#25031,#25032,#25033,#25034,
#25035,#25036,#25037,#25038,#25039,#25040),.UNSPECIFIED.,.F.,.F.,(4,1,1,
1,1,1,1,1,4),(109.955742875643,110.102541384941,111.094937143743,112.087332902544,
113.079728661346,114.072124420147,115.064520178949,116.056915937751,116.238928182822),
 .UNSPECIFIED.);
#2146=B_SPLINE_CURVE_WITH_KNOTS('',3,(#25041,#25042,#25043,#25044,#25045,
#25046,#25047,#25048,#25049,#25050),.UNSPECIFIED.,.F.,.F.,(4,1,1,1,1,1,
1,4),(109.955742875643,110.66078873073,111.653184489532,112.645580248333,
113.637976007135,114.630371765937,115.622767524738,116.238928182822),
 .UNSPECIFIED.);
#2147=B_SPLINE_CURVE_WITH_KNOTS('',3,(#25055,#25056,#25057,#25058,#25059,
#25060,#25061,#25062,#25063,#25064),.UNSPECIFIED.,.F.,.F.,(4,1,1,1,1,1,
1,4),(103.672557568463,104.148166832131,105.140562590933,106.132958349734,
107.125354108536,108.117749867338,109.110145626139,109.955742875643),
 .UNSPECIFIED.);
#2148=B_SPLINE_CURVE_WITH_KNOTS('',3,(#25065,#25066,#25067,#25068,#25069,
#25070,#25071,#25072,#25073,#25074,#25075),.UNSPECIFIED.,.F.,.F.,(4,1,1,
1,1,1,1,1,4),(103.672557568463,103.714018419119,104.70641417792,105.698809936722,
106.691205695524,107.683601454325,108.675997213127,109.668392971929,109.955742875643),
 .UNSPECIFIED.);
#2149=B_SPLINE_CURVE_WITH_KNOTS('',3,(#25080,#25081,#25082,#25083,#25084,
#25085,#25086,#25087,#25088,#25089),.UNSPECIFIED.,.F.,.F.,(4,1,1,1,1,1,
1,4),(97.3893722612835,98.1937922793213,99.1861880381229,100.178583796925,
101.170979555726,102.163375314528,103.155771073329,103.672557568463),
 .UNSPECIFIED.);
#2150=B_SPLINE_CURVE_WITH_KNOTS('',3,(#25090,#25091,#25092,#25093,#25094,
#25095,#25096,#25097,#25098,#25099),.UNSPECIFIED.,.F.,.F.,(4,1,1,1,1,1,
1,4),(97.3893722612835,97.7596438663089,98.7520396251105,99.7444353839122,
100.736831142714,101.729226901515,102.721622660317,103.672557568463),
 .UNSPECIFIED.);
#2151=B_SPLINE_CURVE_WITH_KNOTS('',3,(#25104,#25105,#25106,#25107,#25108,
#25109,#25110,#25111,#25112,#25113,#25114),.UNSPECIFIED.,.F.,.F.,(4,1,1,
1,1,1,1,1,4),(91.106186954104,91.2470219677099,92.2394177265115,93.2318134853131,
94.2242092441148,95.2166050029164,96.209000761718,97.2013965205197,97.3893722612835),
 .UNSPECIFIED.);
#2152=B_SPLINE_CURVE_WITH_KNOTS('',3,(#25115,#25116,#25117,#25118,#25119,
#25120,#25121,#25122,#25123,#25124),.UNSPECIFIED.,.F.,.F.,(4,1,1,1,1,1,
1,4),(91.106186954104,91.8052693134991,92.7976650723007,93.7900608311024,
94.782456589904,95.7748523487057,96.7672481075073,97.3893722612835),
 .UNSPECIFIED.);
#2153=B_SPLINE_CURVE_WITH_KNOTS('',3,(#25129,#25130,#25131,#25132,#25133,
#25134,#25135,#25136,#25137,#25138),.UNSPECIFIED.,.F.,.F.,(4,1,1,1,1,1,
1,4),(84.8230016469243,85.2926474149001,86.2850431737017,87.2774389325033,
88.269834691305,89.2622304501066,90.2546262089082,91.106186954104),
 .UNSPECIFIED.);
#2154=B_SPLINE_CURVE_WITH_KNOTS('',3,(#25139,#25140,#25141,#25142,#25143,
#25144,#25145,#25146,#25147,#25148,#25149),.UNSPECIFIED.,.F.,.F.,(4,1,1,
1,1,1,1,1,4),(84.8230016469243,84.8584990018877,85.8508947606893,86.8432905194909,
87.8356862782926,88.8280820370942,89.8204777958959,90.8128735546975,91.106186954104),
 .UNSPECIFIED.);
#2155=B_SPLINE_CURVE_WITH_KNOTS('',3,(#25154,#25155,#25156,#25157,#25158,
#25159,#25160,#25161,#25162,#25163),.UNSPECIFIED.,.F.,.F.,(4,1,1,1,1,1,
1,4),(78.5398163397448,79.3382728620903,80.3306686208919,81.3230643796935,
82.3154601384952,83.3078558972968,84.3002516560985,84.8230016469243),
 .UNSPECIFIED.);
#2156=B_SPLINE_CURVE_WITH_KNOTS('',3,(#25164,#25165,#25166,#25167,#25168,
#25169,#25170,#25171,#25172,#25173),.UNSPECIFIED.,.F.,.F.,(4,1,1,1,1,1,
1,4),(78.5398163397448,78.9041244490779,79.8965202078795,80.8889159666812,
81.8813117254828,82.8737074842844,83.8661032430861,84.8230016469243),
 .UNSPECIFIED.);
#2157=B_SPLINE_CURVE_WITH_KNOTS('',3,(#25178,#25179,#25180,#25181,#25182,
#25183,#25184,#25185,#25186,#25187,#25188),.UNSPECIFIED.,.F.,.F.,(4,1,1,
1,1,1,1,1,4),(72.2566310325651,72.3915025504788,73.3838983092805,74.3762940680821,
75.3686898268838,76.3610855856854,77.353481344487,78.3458771032886,78.5398163397448),
 .UNSPECIFIED.);
#2158=B_SPLINE_CURVE_WITH_KNOTS('',3,(#25189,#25190,#25191,#25192,#25193,
#25194,#25195,#25196,#25197,#25198),.UNSPECIFIED.,.F.,.F.,(4,1,1,1,1,1,
1,4),(72.2566310325651,72.9497498962681,73.9421456550697,74.9345414138714,
75.926937172673,76.9193329314746,77.9117286902763,78.5398163397448),
 .UNSPECIFIED.);
#2159=B_SPLINE_CURVE_WITH_KNOTS('',3,(#25203,#25204,#25205,#25206,#25207,
#25208,#25209,#25210,#25211,#25212),.UNSPECIFIED.,.F.,.F.,(4,1,1,1,1,1,
1,4),(65.9734457253856,66.4371279976691,67.4295237564707,68.4219195152723,
69.4143152740739,70.4067110328756,71.3991067916772,72.2566310325651),
 .UNSPECIFIED.);
#2160=B_SPLINE_CURVE_WITH_KNOTS('',3,(#25213,#25214,#25215,#25216,#25217,
#25218,#25219,#25220,#25221,#25222,#25223),.UNSPECIFIED.,.F.,.F.,(4,1,1,
1,1,1,1,1,4),(65.9734457253856,66.0029795846567,66.9953753434583,67.9877711022599,
68.9801668610616,69.9725626198632,70.9649583786648,71.9573541374665,72.2566310325651),
 .UNSPECIFIED.);
#2161=B_SPLINE_CURVE_WITH_KNOTS('',3,(#25228,#25229,#25230,#25231,#25232,
#25233,#25234,#25235,#25236,#25237),.UNSPECIFIED.,.F.,.F.,(4,1,1,1,1,1,
1,4),(59.690260418206,60.4827534448593,61.4751492036609,62.4675449624625,
63.4599407212642,64.4523364800658,65.4447322388674,65.9734457253856),
 .UNSPECIFIED.);
#2162=B_SPLINE_CURVE_WITH_KNOTS('',3,(#25238,#25239,#25240,#25241,#25242,
#25243,#25244,#25245,#25246,#25247),.UNSPECIFIED.,.F.,.F.,(4,1,1,1,1,1,
1,4),(59.690260418206,60.0486050318469,61.0410007906485,62.0333965494501,
63.0257923082518,64.0181880670534,65.010583825855,65.9734457253856),
 .UNSPECIFIED.);
#2163=B_SPLINE_CURVE_WITH_KNOTS('',3,(#25252,#25253,#25254,#25255,#25256,
#25257,#25258,#25259,#25260,#25261,#25262),.UNSPECIFIED.,.F.,.F.,(4,1,1,
1,1,1,1,1,4),(53.4070751110264,53.5359831332478,54.5283788920495,55.5207746508511,
56.5131704096527,57.5055661684544,58.497961927256,59.4903576860576,59.690260418206),
 .UNSPECIFIED.);
#2164=B_SPLINE_CURVE_WITH_KNOTS('',3,(#25263,#25264,#25265,#25266,#25267,
#25268,#25269,#25270,#25271,#25272),.UNSPECIFIED.,.F.,.F.,(4,1,1,1,1,1,
1,4),(53.4070751110264,54.0942304790371,55.0866262378387,56.0790219966403,
57.071417755442,58.0638135142436,59.0562092730452,59.690260418206),
 .UNSPECIFIED.);
#2165=B_SPLINE_CURVE_WITH_KNOTS('',3,(#25277,#25278,#25279,#25280,#25281,
#25282,#25283,#25284,#25285,#25286),.UNSPECIFIED.,.F.,.F.,(4,1,1,1,1,1,
1,4),(47.1238898038468,47.581608580438,48.5740043392397,49.5664000980413,
50.5587958568429,51.5511916156446,52.5435873744462,53.4070751110264),
 .UNSPECIFIED.);
#2166=B_SPLINE_CURVE_WITH_KNOTS('',3,(#25287,#25288,#25289,#25290,#25291,
#25292,#25293,#25294,#25295,#25296,#25297),.UNSPECIFIED.,.F.,.F.,(4,1,1,
1,1,1,1,1,4),(47.1238898038468,47.1474601674257,48.1398559262273,49.1322516850289,
50.1246474438306,51.1170432026322,52.1094389614338,53.1018347202355,53.4070751110264),
 .UNSPECIFIED.);
#2167=B_SPLINE_CURVE_WITH_KNOTS('',3,(#25302,#25303,#25304,#25305,#25306,
#25307,#25308,#25309,#25310,#25311),.UNSPECIFIED.,.F.,.F.,(4,1,1,1,1,1,
1,4),(40.8407044966672,41.6272340276282,42.6196297864299,43.6120255452315,
44.6044213040331,45.5968170628348,46.5892128216364,47.1238898038468),
 .UNSPECIFIED.);
#2168=B_SPLINE_CURVE_WITH_KNOTS('',3,(#25312,#25313,#25314,#25315,#25316,
#25317,#25318,#25319,#25320,#25321),.UNSPECIFIED.,.F.,.F.,(4,1,1,1,1,1,
1,4),(40.8407044966672,41.1930856146159,42.1854813734175,43.1778771322191,
44.1702728910208,45.1626686498224,46.155064408624,47.1238898038468),
 .UNSPECIFIED.);
#2169=B_SPLINE_CURVE_WITH_KNOTS('',3,(#25326,#25327,#25328,#25329,#25330,
#25331,#25332,#25333,#25334,#25335,#25336),.UNSPECIFIED.,.F.,.F.,(4,1,1,
1,1,1,1,1,4),(34.5575191894876,34.6804637160168,35.6728594748184,36.6652552336201,
37.6576509924217,38.6500467512233,39.642442510025,40.6348382688266,40.8407044966672),
 .UNSPECIFIED.);
#2170=B_SPLINE_CURVE_WITH_KNOTS('',3,(#25337,#25338,#25339,#25340,#25341,
#25342,#25343,#25344,#25345,#25346),.UNSPECIFIED.,.F.,.F.,(4,1,1,1,1,1,
1,4),(34.5575191894876,35.2387110618061,36.2311068206077,37.2235025794093,
38.215898338211,39.2082940970126,40.2006898558142,40.8407044966672),
 .UNSPECIFIED.);
#2171=B_SPLINE_CURVE_WITH_KNOTS('',3,(#25351,#25352,#25353,#25354,#25355,
#25356,#25357,#25358,#25359,#25360),.UNSPECIFIED.,.F.,.F.,(4,1,1,1,1,1,
1,4),(28.274333882308,28.726089163207,29.7184849220086,30.7108806808103,
31.7032764396119,32.6956721984135,33.6880679572152,34.5575191894876),
 .UNSPECIFIED.);
#2172=B_SPLINE_CURVE_WITH_KNOTS('',3,(#25361,#25362,#25363,#25364,#25365,
#25366,#25367,#25368,#25369,#25370,#25371),.UNSPECIFIED.,.F.,.F.,(4,1,1,
1,1,1,1,1,4),(28.274333882308,28.2919407501946,29.2843365089963,30.2767322677979,
31.2691280265995,32.2615237854012,33.2539195442028,34.2463153030044,34.5575191894876),
 .UNSPECIFIED.);
#2173=B_SPLINE_CURVE_WITH_KNOTS('',3,(#25376,#25377,#25378,#25379,#25380,
#25381,#25382,#25383,#25384,#25385),.UNSPECIFIED.,.F.,.F.,(4,1,1,1,1,1,
1,4),(21.9911485751284,22.7717146103972,23.7641103691988,24.7565061280005,
25.7489018868021,26.7412976456037,27.7336934044054,28.274333882308),
 .UNSPECIFIED.);
#2174=B_SPLINE_CURVE_WITH_KNOTS('',3,(#25386,#25387,#25388,#25389,#25390,
#25391,#25392,#25393,#25394,#25395),.UNSPECIFIED.,.F.,.F.,(4,1,1,1,1,1,
1,4),(21.9911485751284,22.3375661973848,23.3299619561865,24.3223577149881,
25.3147534737897,26.3071492325914,27.299544991393,28.274333882308),
 .UNSPECIFIED.);
#2175=B_SPLINE_CURVE_WITH_KNOTS('',3,(#25401,#25402,#25403,#25404,#25405),
 .UNSPECIFIED.,.F.,.F.,(4,1,4),(14.3984001269718,15.3907958857734,15.7079632679489),
 .UNSPECIFIED.);
#2176=B_SPLINE_CURVE_WITH_KNOTS('',3,(#25408,#25409,#25410,#25411,#25412),
 .UNSPECIFIED.,.F.,.F.,(4,1,4),(13.8759337553361,14.8325485399841,15.7079632679489),
 .UNSPECIFIED.);
#2177=B_SPLINE_CURVE_WITH_KNOTS('',3,(#25414,#25415,#25416,#25417,#25418,
#25419,#25420,#25421,#25422,#25423,#25424,#25425,#25426,#25427,#25428,#25429,
#25430,#25431,#25432,#25433,#25434,#25435,#25436,#25437,#25438,#25439,#25440,
#25441,#25442,#25443,#25444,#25445,#25446,#25447,#25448,#25449,#25450,#25451,
#25452,#25453,#25454,#25455,#25456,#25457,#25458,#25459,#25460,#25461,#25462,
#25463,#25464,#25465),.UNSPECIFIED.,.F.,.F.,(4,3,3,3,3,3,3,3,3,3,3,3,3,
3,3,3,3,4),(-0.286347380332279,-0.266347789416864,-0.254098115456061,-0.230501751705225,
-0.216536610693349,-0.18668269284242,-0.173443188538191,-0.164130900566406,
-0.152678732927651,-0.129952909210668,-0.116365164485228,-0.106745630798174,
-0.0814440134366876,-0.0640046809373957,-0.0520446962100768,-0.0197039455308333,
-0.00553916135222766,0.),.UNSPECIFIED.);
#2178=B_SPLINE_CURVE_WITH_KNOTS('',3,(#25466,#25467,#25468,#25469,#25470,
#25471,#25472,#25473,#25474,#25475,#25476,#25477,#25478,#25479,#25480,#25481,
#25482,#25483,#25484,#25485,#25486,#25487,#25488,#25489,#25490,#25491,#25492,
#25493,#25494,#25495,#25496,#25497,#25498,#25499,#25500,#25501,#25502,#25503,
#25504,#25505,#25506,#25507,#25508,#25509,#25510,#25511,#25512,#25513,#25514,
#25515,#25516,#25517,#25518,#25519,#25520),.UNSPECIFIED.,.F.,.F.,(4,3,3,
3,3,3,3,3,3,3,3,3,3,3,3,3,3,3,4),(-0.2851428039951,-0.264876660632172,-0.2498967274825,
-0.236025660645345,-0.214587312757531,-0.204671023974553,-0.173775777047669,
-0.160111619860766,-0.150128525406277,-0.138317788758425,-0.118237251615849,
-0.10321155298755,-0.092840846421164,-0.0707715126256338,-0.0558839316601653,
-0.043797399607841,-0.0161434201156718,-0.00456351123904309,0.),
 .UNSPECIFIED.);
#2179=B_SPLINE_CURVE_WITH_KNOTS('',3,(#25522,#25523,#25524,#25525,#25526,
#25527,#25528,#25529,#25530,#25531,#25532),.UNSPECIFIED.,.F.,.F.,(4,1,1,
1,1,1,1,1,4),(15.7079632679489,15.8249442987858,16.8173400575874,17.809735816389,
18.8021315751907,19.7945273339923,20.7869230927939,21.7793188515956,21.9911485751284),
 .UNSPECIFIED.);
#2180=B_SPLINE_CURVE_WITH_KNOTS('',3,(#25533,#25534,#25535,#25536,#25537,
#25538,#25539,#25540,#25541,#25542),.UNSPECIFIED.,.F.,.F.,(4,1,1,1,1,1,
1,4),(15.7079632679489,16.383191644575,17.3755874033767,18.3679831621783,
19.3603789209799,20.3527746797816,21.3451704385832,21.9911485751284),
 .UNSPECIFIED.);
#2181=B_SPLINE_CURVE_WITH_KNOTS('',3,(#26019,#26020,#26021,#26022,#26023,
#26024,#26025,#26026,#26027,#26028,#26029,#26030,#26031,#26032,#26033,#26034,
#26035,#26036,#26037,#26038,#26039,#26040,#26041,#26042,#26043,#26044,#26045,
#26046,#26047,#26048,#26049,#26050,#26051,#26052,#26053,#26054,#26055,#26056,
#26057,#26058,#26059,#26060,#26061,#26062,#26063,#26064,#26065,#26066,#26067),
 .UNSPECIFIED.,.F.,.F.,(4,3,3,3,3,3,3,3,3,3,3,3,3,3,3,3,4),(0.,0.027427935344833,
0.0485975213880563,0.057338544085104,0.0868715743464506,0.0993492225585254,
0.10874754786483,0.133259321258805,0.148225404936155,0.157073224224447,
0.187711488807199,0.203788900709552,0.214227532674886,0.239511221647469,
0.25730153039039,0.279626282555456,0.285142803995123),.UNSPECIFIED.);
#2182=B_SPLINE_CURVE_WITH_KNOTS('',3,(#26068,#26069,#26070,#26071,#26072,
#26073,#26074,#26075,#26076,#26077,#26078,#26079,#26080,#26081,#26082,#26083,
#26084,#26085,#26086,#26087,#26088,#26089,#26090,#26091,#26092),
 .UNSPECIFIED.,.F.,.F.,(4,3,3,3,3,3,3,3,4),(-10.1357873115492,-9.92395758801633,
-8.9315618292147,-7.93916607041306,-6.94677031161143,-5.9543745528098,-4.96197879400816,
-3.96958303520653,-3.85260200436961),.UNSPECIFIED.);
#2183=B_SPLINE_CURVE_WITH_KNOTS('',3,(#26569,#26570,#26571,#26572,#26573,
#26574,#26575,#26576,#26577,#26578,#26579,#26580,#26581,#26582,#26583,#26584,
#26585,#26586,#26587,#26588,#26589,#26590),.UNSPECIFIED.,.F.,.F.,(4,3,3,
3,3,3,3,4),(7.59274844815659,7.93916607041306,8.9315618292147,9.92395758801632,
10.916353346818,11.9087491056196,12.9011448644212,13.8759337553361),
 .UNSPECIFIED.);
#2184=B_SPLINE_CURVE_WITH_KNOTS('',3,(#26591,#26592,#26593,#26594,#26595,
#26596,#26597,#26598,#26599,#26600,#26601,#26602,#26603,#26604,#26605,#26606,
#26607,#26608,#26609,#26610,#26611,#26612,#26613,#26614,#26615,#26616,#26617,
#26618,#26619,#26620,#26621,#26622,#26623,#26624,#26625,#26626,#26627,#26628,
#26629,#26630,#26631,#26632,#26633,#26634,#26635,#26636,#26637,#26638,#26639),
 .UNSPECIFIED.,.F.,.F.,(4,3,3,3,3,3,3,3,3,3,3,3,3,3,3,3,4),(0.,0.0320359961493654,
0.0578351282991586,0.0686833515155324,0.0999463544758613,0.113502099149543,
0.123023834848469,0.14759884188358,0.169881710030997,0.180117784856696,
0.205530503004595,0.220530951880297,0.231030371326071,0.247789211594336,
0.263619336128737,0.281768657448294,0.286347380332258),.UNSPECIFIED.);
#2185=B_SPLINE_CURVE_WITH_KNOTS('',3,(#26643,#26644,#26645,#26646,#26647,
#26648,#26649,#26650,#26651,#26652,#26653,#26654,#26655,#26656,#26657,#26658,
#26659,#26660,#26661,#26662,#26663,#26664,#26665,#26666,#26667,#26668,#26669,
#26670,#26671,#26672,#26673,#26674,#26675,#26676,#26677,#26678,#26679,#26680,
#26681,#26682,#26683,#26684,#26685,#26686,#26687,#26688,#26689,#26690,#26691,
#26692,#26693,#26694,#26695,#26696,#26697),.UNSPECIFIED.,.F.,.F.,(4,3,3,
3,3,3,3,3,3,3,3,3,3,3,3,3,3,3,4),(-0.378621596831434,-0.353562249903933,
-0.339726595154467,-0.324795073175994,-0.299958563910779,-0.289109739323556,
-0.25235894447449,-0.234461207277299,-0.219335840287605,-0.20082949567809,
-0.174834335133969,-0.155874235881852,-0.144961055903939,-0.109724944879178,
-0.089723852283725,-0.0773553386782937,-0.0372306048514265,-0.00401661180489575,
0.),.UNSPECIFIED.);
#2186=B_SPLINE_CURVE_WITH_KNOTS('',3,(#26698,#26699,#26700,#26701,#26702,
#26703,#26704,#26705,#26706,#26707,#26708,#26709,#26710,#26711,#26712,#26713,
#26714,#26715,#26716,#26717,#26718,#26719,#26720,#26721,#26722,#26723,#26724,
#26725,#26726,#26727,#26728,#26729,#26730,#26731,#26732,#26733,#26734,#26735,
#26736,#26737,#26738,#26739,#26740,#26741,#26742,#26743,#26744,#26745,#26746,
#26747,#26748,#26749,#26750,#26751,#26752),.UNSPECIFIED.,.F.,.F.,(4,3,3,
3,3,3,3,3,3,3,3,3,3,3,3,3,3,3,4),(-0.376940817211603,-0.35160224691684,
-0.332515709335319,-0.31822436103578,-0.288310916204436,-0.272711478712379,
-0.234501138719602,-0.216951876329547,-0.20548608487052,-0.180854828870935,
-0.153741722238776,-0.136717958714649,-0.126362699189128,-0.0955896266494597,
-0.0668165609022854,-0.0558907541314208,-0.0219997397314357,-0.00327040903045418,
0.),.UNSPECIFIED.);
#2187=B_SPLINE_CURVE_WITH_KNOTS('',3,(#26754,#26755,#26756,#26757,#26758,
#26759,#26760,#26761,#26762,#26763,#26764),.UNSPECIFIED.,.F.,.F.,(4,1,1,
1,1,1,1,1,4),(15.7079632679489,15.8518654961884,16.8494368691713,17.8470082421542,
18.8445796151372,19.8421509881201,20.839722361103,21.837293734086,21.9911485751285),
 .UNSPECIFIED.);
#2188=B_SPLINE_CURVE_WITH_KNOTS('',3,(#26765,#26766,#26767,#26768,#26769,
#26770,#26771,#26772,#26773,#26774),.UNSPECIFIED.,.F.,.F.,(4,1,1,1,1,1,
1,4),(15.7079632679489,16.3932837587428,17.3908551317257,18.3884265047086,
19.3859978776916,20.3835692506745,21.3811406236574,21.9911485751285),
 .UNSPECIFIED.);
#2189=B_SPLINE_CURVE_WITH_KNOTS('',3,(#27119,#27120,#27121,#27122,#27123,
#27124,#27125,#27126,#27127,#27128,#27129,#27130,#27131,#27132,#27133,#27134,
#27135,#27136,#27137,#27138,#27139,#27140,#27141,#27142,#27143,#27144,#27145,
#27146,#27147,#27148,#27149,#27150,#27151,#27152,#27153,#27154,#27155,#27156,
#27157,#27158,#27159,#27160,#27161,#27162,#27163,#27164,#27165,#27166,#27167,
#27168,#27169,#27170),.UNSPECIFIED.,.F.,.F.,(4,3,3,3,3,3,3,3,3,3,3,3,3,
3,3,3,3,4),(0.,0.0336989330766502,0.058737806914676,0.0734856897216009,
0.109795026944167,0.13287001176372,0.143641059388719,0.177205256270034,
0.195910789941764,0.207613330853891,0.24488927972035,0.269584354829063,
0.282495236861346,0.310139624218381,0.327566593080831,0.34255192583909,
0.372940760482297,0.376940817211641),.UNSPECIFIED.);
#2190=B_SPLINE_CURVE_WITH_KNOTS('',3,(#27171,#27172,#27173,#27174,#27175,
#27176,#27177,#27178,#27179,#27180,#27181,#27182,#27183,#27184,#27185,#27186,
#27187,#27188,#27189,#27190,#27191,#27192,#27193,#27194,#27195),
 .UNSPECIFIED.,.F.,.F.,(4,3,3,3,3,3,3,3,4),(-10.1295685708718,-9.97571372982933,
-8.9781423568464,-7.98057098386346,-6.98299961088053,-5.9854282378976,-4.98785686491466,
-3.99028549193173,-3.84638326369226),.UNSPECIFIED.);
#2191=B_SPLINE_CURVE_WITH_KNOTS('',3,(#27540,#27541,#27542,#27543,#27544,
#27545,#27546,#27547,#27548,#27549,#27550,#27551,#27552,#27553,#27554,#27555,
#27556,#27557,#27558,#27559,#27560,#27561),.UNSPECIFIED.,.F.,.F.,(4,3,3,
3,3,3,3,4),(7.59300756235155,7.98057098386346,8.9781423568464,9.97571372982933,
10.9732851028123,11.9708564757952,12.9684278487781,13.8761928695311),
 .UNSPECIFIED.);
#2192=B_SPLINE_CURVE_WITH_KNOTS('',3,(#27562,#27563,#27564,#27565,#27566,
#27567,#27568,#27569,#27570,#27571,#27572,#27573,#27574,#27575,#27576,#27577,
#27578,#27579,#27580,#27581,#27582,#27583,#27584,#27585,#27586,#27587,#27588,
#27589,#27590,#27591,#27592,#27593,#27594,#27595,#27596,#27597,#27598,#27599,
#27600,#27601,#27602,#27603,#27604,#27605,#27606,#27607,#27608,#27609,#27610,
#27611,#27612,#27613),.UNSPECIFIED.,.F.,.F.,(4,3,3,3,3,3,3,3,3,3,3,3,3,
3,3,3,3,4),(0.,0.0396836996751474,0.0598295377036724,0.0776045542344442,
0.089287041955902,0.127960856426141,0.1530367876033,0.165008599097631,0.197163594226426,
0.224449840232547,0.234157399588655,0.269452851616206,0.2876129966593,0.30541494242687,
0.333061769489462,0.34722178230466,0.375339207698859,0.378621596831421),
 .UNSPECIFIED.);
#2727=LINE('',#23210,#3301);
#2728=LINE('',#23245,#3302);
#2729=LINE('',#23272,#3303);
#2730=LINE('',#23323,#3304);
#2731=LINE('',#23371,#3305);
#2732=LINE('',#23419,#3306);
#2733=LINE('',#23470,#3307);
#2734=LINE('',#23518,#3308);
#2735=LINE('',#23566,#3309);
#2736=LINE('',#23617,#3310);
#2737=LINE('',#23668,#3311);
#2738=LINE('',#23716,#3312);
#2739=LINE('',#23767,#3313);
#2740=LINE('',#23806,#3314);
#2741=LINE('',#23828,#3315);
#2742=LINE('',#23852,#3316);
#2743=LINE('',#23877,#3317);
#2744=LINE('',#23902,#3318);
#2745=LINE('',#23926,#3319);
#2746=LINE('',#23951,#3320);
#2747=LINE('',#23975,#3321);
#2748=LINE('',#24000,#3322);
#2749=LINE('',#24024,#3323);
#2750=LINE('',#24049,#3324);
#2751=LINE('',#24074,#3325);
#2752=LINE('',#24098,#3326);
#2753=LINE('',#24115,#3327);
#2754=LINE('',#24124,#3328);
#2755=LINE('',#24141,#3329);
#2756=LINE('',#24192,#3330);
#2757=LINE('',#24243,#3331);
#2758=LINE('',#24291,#3332);
#2759=LINE('',#24342,#3333);
#2760=LINE('',#24393,#3334);
#2761=LINE('',#24441,#3335);
#2762=LINE('',#24492,#3336);
#2763=LINE('',#24543,#3337);
#2764=LINE('',#24591,#3338);
#2765=LINE('',#24642,#3339);
#2766=LINE('',#24693,#3340);
#2767=LINE('',#24741,#3341);
#2768=LINE('',#24792,#3342);
#2769=LINE('',#24843,#3343);
#2770=LINE('',#24891,#3344);
#2771=LINE('',#24942,#3345);
#2772=LINE('',#24981,#3346);
#2773=LINE('',#25005,#3347);
#2774=LINE('',#25029,#3348);
#2775=LINE('',#25054,#3349);
#2776=LINE('',#25079,#3350);
#2777=LINE('',#25103,#3351);
#2778=LINE('',#25128,#3352);
#2779=LINE('',#25153,#3353);
#2780=LINE('',#25177,#3354);
#2781=LINE('',#25202,#3355);
#2782=LINE('',#25227,#3356);
#2783=LINE('',#25251,#3357);
#2784=LINE('',#25276,#3358);
#2785=LINE('',#25301,#3359);
#2786=LINE('',#25325,#3360);
#2787=LINE('',#25350,#3361);
#2788=LINE('',#25375,#3362);
#2789=LINE('',#25399,#3363);
#2790=LINE('',#27619,#3364);
#2791=LINE('',#27621,#3365);
#2792=LINE('',#27623,#3366);
#2793=LINE('',#27624,#3367);
#2794=LINE('',#27627,#3368);
#2795=LINE('',#27629,#3369);
#2796=LINE('',#27630,#3370);
#2797=LINE('',#27633,#3371);
#2798=LINE('',#27635,#3372);
#2799=LINE('',#27636,#3373);
#2800=LINE('',#27638,#3374);
#2801=LINE('',#27639,#3375);
#3301=VECTOR('',#11660,0.2);
#3302=VECTOR('',#11663,0.2);
#3303=VECTOR('',#11668,0.2);
#3304=VECTOR('',#11671,0.2);
#3305=VECTOR('',#11674,0.2);
#3306=VECTOR('',#11677,0.2);
#3307=VECTOR('',#11680,0.2);
#3308=VECTOR('',#11683,0.2);
#3309=VECTOR('',#11686,0.2);
#3310=VECTOR('',#11689,0.2);
#3311=VECTOR('',#11692,0.2);
#3312=VECTOR('',#11695,0.2);
#3313=VECTOR('',#11698,0.2);
#3314=VECTOR('',#11703,0.205475);
#3315=VECTOR('',#11708,0.205475);
#3316=VECTOR('',#11711,0.205475);
#3317=VECTOR('',#11714,0.205475);
#3318=VECTOR('',#11717,0.205475);
#3319=VECTOR('',#11720,0.205475);
#3320=VECTOR('',#11723,0.205475);
#3321=VECTOR('',#11726,0.205475);
#3322=VECTOR('',#11729,0.205475);
#3323=VECTOR('',#11732,0.205475);
#3324=VECTOR('',#11735,0.205475);
#3325=VECTOR('',#11738,0.205475);
#3326=VECTOR('',#11741,0.205475);
#3327=VECTOR('',#11746,0.15);
#3328=VECTOR('',#11749,0.15);
#3329=VECTOR('',#11756,0.15);
#3330=VECTOR('',#11759,0.15);
#3331=VECTOR('',#11762,0.15);
#3332=VECTOR('',#11765,0.15);
#3333=VECTOR('',#11768,0.15);
#3334=VECTOR('',#11771,0.15);
#3335=VECTOR('',#11774,0.15);
#3336=VECTOR('',#11777,0.15);
#3337=VECTOR('',#11780,0.15);
#3338=VECTOR('',#11783,0.15);
#3339=VECTOR('',#11786,0.15);
#3340=VECTOR('',#11789,0.15);
#3341=VECTOR('',#11792,0.15);
#3342=VECTOR('',#11795,0.15);
#3343=VECTOR('',#11798,0.15);
#3344=VECTOR('',#11801,0.15);
#3345=VECTOR('',#11804,0.15);
#3346=VECTOR('',#11809,0.1543);
#3347=VECTOR('',#11814,0.1543);
#3348=VECTOR('',#11817,0.1543);
#3349=VECTOR('',#11820,0.1543);
#3350=VECTOR('',#11823,0.1543);
#3351=VECTOR('',#11826,0.1543);
#3352=VECTOR('',#11829,0.1543);
#3353=VECTOR('',#11832,0.1543);
#3354=VECTOR('',#11835,0.1543);
#3355=VECTOR('',#11838,0.1543);
#3356=VECTOR('',#11841,0.1543);
#3357=VECTOR('',#11844,0.1543);
#3358=VECTOR('',#11847,0.1543);
#3359=VECTOR('',#11850,0.1543);
#3360=VECTOR('',#11853,0.1543);
#3361=VECTOR('',#11856,0.1543);
#3362=VECTOR('',#11859,0.1543);
#3363=VECTOR('',#11862,0.1543);
#3364=VECTOR('',#11883,1.);
#3365=VECTOR('',#11884,1.);
#3366=VECTOR('',#11885,1.);
#3367=VECTOR('',#11886,1.);
#3368=VECTOR('',#11889,1.);
#3369=VECTOR('',#11890,1.);
#3370=VECTOR('',#11891,1.);
#3371=VECTOR('',#11894,1.);
#3372=VECTOR('',#11895,1.);
#3373=VECTOR('',#11896,1.);
#3374=VECTOR('',#11899,1.);
#3375=VECTOR('',#11900,1.);
#4051=VERTEX_POINT('',#23208);
#4052=VERTEX_POINT('',#23209);
#4053=VERTEX_POINT('',#23211);
#4054=VERTEX_POINT('',#23234);
#4055=VERTEX_POINT('',#23236);
#4056=VERTEX_POINT('',#23244);
#4057=VERTEX_POINT('',#23270);
#4058=VERTEX_POINT('',#23271);
#4059=VERTEX_POINT('',#23321);
#4060=VERTEX_POINT('',#23322);
#4061=VERTEX_POINT('',#23369);
#4062=VERTEX_POINT('',#23370);
#4063=VERTEX_POINT('',#23417);
#4064=VERTEX_POINT('',#23418);
#4065=VERTEX_POINT('',#23468);
#4066=VERTEX_POINT('',#23469);
#4067=VERTEX_POINT('',#23516);
#4068=VERTEX_POINT('',#23517);
#4069=VERTEX_POINT('',#23564);
#4070=VERTEX_POINT('',#23565);
#4071=VERTEX_POINT('',#23615);
#4072=VERTEX_POINT('',#23616);
#4073=VERTEX_POINT('',#23666);
#4074=VERTEX_POINT('',#23667);
#4075=VERTEX_POINT('',#23714);
#4076=VERTEX_POINT('',#23715);
#4077=VERTEX_POINT('',#23765);
#4078=VERTEX_POINT('',#23766);
#4079=VERTEX_POINT('',#23768);
#4080=VERTEX_POINT('',#23782);
#4081=VERTEX_POINT('',#23804);
#4082=VERTEX_POINT('',#23805);
#4083=VERTEX_POINT('',#23807);
#4084=VERTEX_POINT('',#23815);
#4085=VERTEX_POINT('',#23826);
#4086=VERTEX_POINT('',#23827);
#4087=VERTEX_POINT('',#23850);
#4088=VERTEX_POINT('',#23851);
#4089=VERTEX_POINT('',#23875);
#4090=VERTEX_POINT('',#23876);
#4091=VERTEX_POINT('',#23900);
#4092=VERTEX_POINT('',#23901);
#4093=VERTEX_POINT('',#23924);
#4094=VERTEX_POINT('',#23925);
#4095=VERTEX_POINT('',#23949);
#4096=VERTEX_POINT('',#23950);
#4097=VERTEX_POINT('',#23973);
#4098=VERTEX_POINT('',#23974);
#4099=VERTEX_POINT('',#23998);
#4100=VERTEX_POINT('',#23999);
#4101=VERTEX_POINT('',#24022);
#4102=VERTEX_POINT('',#24023);
#4103=VERTEX_POINT('',#24047);
#4104=VERTEX_POINT('',#24048);
#4105=VERTEX_POINT('',#24072);
#4106=VERTEX_POINT('',#24073);
#4107=VERTEX_POINT('',#24096);
#4108=VERTEX_POINT('',#24097);
#4109=VERTEX_POINT('',#24099);
#4110=VERTEX_POINT('',#24105);
#4111=VERTEX_POINT('',#24113);
#4112=VERTEX_POINT('',#24114);
#4113=VERTEX_POINT('',#24116);
#4114=VERTEX_POINT('',#24121);
#4115=VERTEX_POINT('',#24123);
#4116=VERTEX_POINT('',#24126);
#4117=VERTEX_POINT('',#24139);
#4118=VERTEX_POINT('',#24140);
#4119=VERTEX_POINT('',#24190);
#4120=VERTEX_POINT('',#24191);
#4121=VERTEX_POINT('',#24241);
#4122=VERTEX_POINT('',#24242);
#4123=VERTEX_POINT('',#24289);
#4124=VERTEX_POINT('',#24290);
#4125=VERTEX_POINT('',#24340);
#4126=VERTEX_POINT('',#24341);
#4127=VERTEX_POINT('',#24391);
#4128=VERTEX_POINT('',#24392);
#4129=VERTEX_POINT('',#24439);
#4130=VERTEX_POINT('',#24440);
#4131=VERTEX_POINT('',#24490);
#4132=VERTEX_POINT('',#24491);
#4133=VERTEX_POINT('',#24541);
#4134=VERTEX_POINT('',#24542);
#4135=VERTEX_POINT('',#24589);
#4136=VERTEX_POINT('',#24590);
#4137=VERTEX_POINT('',#24640);
#4138=VERTEX_POINT('',#24641);
#4139=VERTEX_POINT('',#24691);
#4140=VERTEX_POINT('',#24692);
#4141=VERTEX_POINT('',#24739);
#4142=VERTEX_POINT('',#24740);
#4143=VERTEX_POINT('',#24790);
#4144=VERTEX_POINT('',#24791);
#4145=VERTEX_POINT('',#24841);
#4146=VERTEX_POINT('',#24842);
#4147=VERTEX_POINT('',#24889);
#4148=VERTEX_POINT('',#24890);
#4149=VERTEX_POINT('',#24940);
#4150=VERTEX_POINT('',#24941);
#4151=VERTEX_POINT('',#24943);
#4152=VERTEX_POINT('',#24957);
#4153=VERTEX_POINT('',#24979);
#4154=VERTEX_POINT('',#24980);
#4155=VERTEX_POINT('',#24982);
#4156=VERTEX_POINT('',#24991);
#4157=VERTEX_POINT('',#25003);
#4158=VERTEX_POINT('',#25004);
#4159=VERTEX_POINT('',#25027);
#4160=VERTEX_POINT('',#25028);
#4161=VERTEX_POINT('',#25052);
#4162=VERTEX_POINT('',#25053);
#4163=VERTEX_POINT('',#25077);
#4164=VERTEX_POINT('',#25078);
#4165=VERTEX_POINT('',#25101);
#4166=VERTEX_POINT('',#25102);
#4167=VERTEX_POINT('',#25126);
#4168=VERTEX_POINT('',#25127);
#4169=VERTEX_POINT('',#25151);
#4170=VERTEX_POINT('',#25152);
#4171=VERTEX_POINT('',#25175);
#4172=VERTEX_POINT('',#25176);
#4173=VERTEX_POINT('',#25200);
#4174=VERTEX_POINT('',#25201);
#4175=VERTEX_POINT('',#25225);
#4176=VERTEX_POINT('',#25226);
#4177=VERTEX_POINT('',#25249);
#4178=VERTEX_POINT('',#25250);
#4179=VERTEX_POINT('',#25274);
#4180=VERTEX_POINT('',#25275);
#4181=VERTEX_POINT('',#25299);
#4182=VERTEX_POINT('',#25300);
#4183=VERTEX_POINT('',#25323);
#4184=VERTEX_POINT('',#25324);
#4185=VERTEX_POINT('',#25348);
#4186=VERTEX_POINT('',#25349);
#4187=VERTEX_POINT('',#25373);
#4188=VERTEX_POINT('',#25374);
#4189=VERTEX_POINT('',#25397);
#4190=VERTEX_POINT('',#25398);
#4191=VERTEX_POINT('',#25400);
#4192=VERTEX_POINT('',#25406);
#4193=VERTEX_POINT('',#27617);
#4194=VERTEX_POINT('',#27618);
#4195=VERTEX_POINT('',#27620);
#4196=VERTEX_POINT('',#27622);
#4197=VERTEX_POINT('',#27626);
#4198=VERTEX_POINT('',#27628);
#4199=VERTEX_POINT('',#27632);
#4200=VERTEX_POINT('',#27634);
#5239=EDGE_CURVE('',#4051,#4052,#2727,.T.);
#5240=EDGE_CURVE('',#4052,#4053,#2054,.T.);
#5241=EDGE_CURVE('',#4053,#4054,#1674,.T.);
#5242=EDGE_CURVE('',#4054,#4055,#2055,.T.);
#5243=EDGE_CURVE('',#4055,#4056,#2728,.T.);
#5244=EDGE_CURVE('',#4056,#4056,#1675,.F.);
#5245=EDGE_CURVE('',#4055,#4051,#2056,.T.);
#5246=EDGE_CURVE('',#4057,#4058,#2729,.T.);
#5247=EDGE_CURVE('',#4058,#4052,#2057,.T.);
#5248=EDGE_CURVE('',#4051,#4057,#2058,.T.);
#5249=EDGE_CURVE('',#4059,#4060,#2730,.T.);
#5250=EDGE_CURVE('',#4060,#4058,#2059,.T.);
#5251=EDGE_CURVE('',#4057,#4059,#2060,.T.);
#5252=EDGE_CURVE('',#4061,#4062,#2731,.T.);
#5253=EDGE_CURVE('',#4062,#4060,#2061,.T.);
#5254=EDGE_CURVE('',#4059,#4061,#2062,.T.);
#5255=EDGE_CURVE('',#4063,#4064,#2732,.T.);
#5256=EDGE_CURVE('',#4064,#4062,#2063,.T.);
#5257=EDGE_CURVE('',#4061,#4063,#2064,.T.);
#5258=EDGE_CURVE('',#4065,#4066,#2733,.T.);
#5259=EDGE_CURVE('',#4066,#4064,#2065,.T.);
#5260=EDGE_CURVE('',#4063,#4065,#2066,.T.);
#5261=EDGE_CURVE('',#4067,#4068,#2734,.T.);
#5262=EDGE_CURVE('',#4068,#4066,#2067,.T.);
#5263=EDGE_CURVE('',#4065,#4067,#2068,.T.);
#5264=EDGE_CURVE('',#4069,#4070,#2735,.T.);
#5265=EDGE_CURVE('',#4070,#4068,#2069,.T.);
#5266=EDGE_CURVE('',#4067,#4069,#2070,.T.);
#5267=EDGE_CURVE('',#4071,#4072,#2736,.T.);
#5268=EDGE_CURVE('',#4072,#4070,#2071,.T.);
#5269=EDGE_CURVE('',#4069,#4071,#2072,.T.);
#5270=EDGE_CURVE('',#4073,#4074,#2737,.T.);
#5271=EDGE_CURVE('',#4074,#4072,#2073,.T.);
#5272=EDGE_CURVE('',#4071,#4073,#2074,.T.);
#5273=EDGE_CURVE('',#4075,#4076,#2738,.T.);
#5274=EDGE_CURVE('',#4076,#4074,#2075,.T.);
#5275=EDGE_CURVE('',#4073,#4075,#2076,.T.);
#5276=EDGE_CURVE('',#4077,#4078,#2739,.T.);
#5277=EDGE_CURVE('',#4077,#4079,#2077,.T.);
#5278=EDGE_CURVE('',#4080,#4079,#1676,.F.);
#5279=EDGE_CURVE('',#4080,#4078,#2078,.T.);
#5280=EDGE_CURVE('',#4081,#4082,#2740,.T.);
#5281=EDGE_CURVE('',#4082,#4083,#2079,.T.);
#5282=EDGE_CURVE('',#4084,#4083,#1677,.T.);
#5283=EDGE_CURVE('',#4081,#4084,#2080,.T.);
#5284=EDGE_CURVE('',#4085,#4086,#2741,.T.);
#5285=EDGE_CURVE('',#4086,#4082,#2081,.T.);
#5286=EDGE_CURVE('',#4085,#4081,#2082,.T.);
#5287=EDGE_CURVE('',#4087,#4088,#2742,.T.);
#5288=EDGE_CURVE('',#4088,#4086,#2083,.T.);
#5289=EDGE_CURVE('',#4087,#4085,#2084,.T.);
#5290=EDGE_CURVE('',#4089,#4090,#2743,.T.);
#5291=EDGE_CURVE('',#4090,#4088,#2085,.T.);
#5292=EDGE_CURVE('',#4089,#4087,#2086,.T.);
#5293=EDGE_CURVE('',#4091,#4092,#2744,.T.);
#5294=EDGE_CURVE('',#4092,#4090,#2087,.T.);
#5295=EDGE_CURVE('',#4091,#4089,#2088,.T.);
#5296=EDGE_CURVE('',#4093,#4094,#2745,.T.);
#5297=EDGE_CURVE('',#4094,#4092,#2089,.T.);
#5298=EDGE_CURVE('',#4093,#4091,#2090,.T.);
#5299=EDGE_CURVE('',#4095,#4096,#2746,.T.);
#5300=EDGE_CURVE('',#4096,#4094,#2091,.T.);
#5301=EDGE_CURVE('',#4095,#4093,#2092,.T.);
#5302=EDGE_CURVE('',#4097,#4098,#2747,.T.);
#5303=EDGE_CURVE('',#4098,#4096,#2093,.T.);
#5304=EDGE_CURVE('',#4097,#4095,#2094,.T.);
#5305=EDGE_CURVE('',#4099,#4100,#2748,.T.);
#5306=EDGE_CURVE('',#4100,#4098,#2095,.T.);
#5307=EDGE_CURVE('',#4099,#4097,#2096,.T.);
#5308=EDGE_CURVE('',#4101,#4102,#2749,.T.);
#5309=EDGE_CURVE('',#4102,#4100,#2097,.T.);
#5310=EDGE_CURVE('',#4101,#4099,#2098,.T.);
#5311=EDGE_CURVE('',#4103,#4104,#2750,.T.);
#5312=EDGE_CURVE('',#4104,#4102,#2099,.T.);
#5313=EDGE_CURVE('',#4103,#4101,#2100,.T.);
#5314=EDGE_CURVE('',#4105,#4106,#2751,.T.);
#5315=EDGE_CURVE('',#4106,#4104,#2101,.T.);
#5316=EDGE_CURVE('',#4105,#4103,#2102,.T.);
#5317=EDGE_CURVE('',#4107,#4108,#2752,.T.);
#5318=EDGE_CURVE('',#4109,#4107,#2103,.T.);
#5319=EDGE_CURVE('',#4110,#4109,#1678,.T.);
#5320=EDGE_CURVE('',#4110,#4108,#2104,.T.);
#5321=EDGE_CURVE('',#4111,#4112,#2753,.T.);
#5322=EDGE_CURVE('',#4112,#4113,#2105,.T.);
#5323=EDGE_CURVE('',#4113,#4114,#1679,.T.);
#5324=EDGE_CURVE('',#4114,#4115,#2754,.T.);
#5325=EDGE_CURVE('',#4115,#4115,#1680,.F.);
#5326=EDGE_CURVE('',#4114,#4116,#1681,.T.);
#5327=EDGE_CURVE('',#4116,#4111,#2106,.T.);
#5328=EDGE_CURVE('',#4117,#4118,#2755,.T.);
#5329=EDGE_CURVE('',#4118,#4112,#2107,.T.);
#5330=EDGE_CURVE('',#4111,#4117,#2108,.T.);
#5331=EDGE_CURVE('',#4119,#4120,#2756,.T.);
#5332=EDGE_CURVE('',#4120,#4118,#2109,.T.);
#5333=EDGE_CURVE('',#4117,#4119,#2110,.T.);
#5334=EDGE_CURVE('',#4121,#4122,#2757,.T.);
#5335=EDGE_CURVE('',#4122,#4120,#2111,.T.);
#5336=EDGE_CURVE('',#4119,#4121,#2112,.T.);
#5337=EDGE_CURVE('',#4123,#4124,#2758,.T.);
#5338=EDGE_CURVE('',#4124,#4122,#2113,.T.);
#5339=EDGE_CURVE('',#4121,#4123,#2114,.T.);
#5340=EDGE_CURVE('',#4125,#4126,#2759,.T.);
#5341=EDGE_CURVE('',#4126,#4124,#2115,.T.);
#5342=EDGE_CURVE('',#4123,#4125,#2116,.T.);
#5343=EDGE_CURVE('',#4127,#4128,#2760,.T.);
#5344=EDGE_CURVE('',#4128,#4126,#2117,.T.);
#5345=EDGE_CURVE('',#4125,#4127,#2118,.T.);
#5346=EDGE_CURVE('',#4129,#4130,#2761,.T.);
#5347=EDGE_CURVE('',#4130,#4128,#2119,.T.);
#5348=EDGE_CURVE('',#4127,#4129,#2120,.T.);
#5349=EDGE_CURVE('',#4131,#4132,#2762,.T.);
#5350=EDGE_CURVE('',#4132,#4130,#2121,.T.);
#5351=EDGE_CURVE('',#4129,#4131,#2122,.T.);
#5352=EDGE_CURVE('',#4133,#4134,#2763,.T.);
#5353=EDGE_CURVE('',#4134,#4132,#2123,.T.);
#5354=EDGE_CURVE('',#4131,#4133,#2124,.T.);
#5355=EDGE_CURVE('',#4135,#4136,#2764,.T.);
#5356=EDGE_CURVE('',#4136,#4134,#2125,.T.);
#5357=EDGE_CURVE('',#4133,#4135,#2126,.T.);
#5358=EDGE_CURVE('',#4137,#4138,#2765,.T.);
#5359=EDGE_CURVE('',#4138,#4136,#2127,.T.);
#5360=EDGE_CURVE('',#4135,#4137,#2128,.T.);
#5361=EDGE_CURVE('',#4139,#4140,#2766,.T.);
#5362=EDGE_CURVE('',#4140,#4138,#2129,.T.);
#5363=EDGE_CURVE('',#4137,#4139,#2130,.T.);
#5364=EDGE_CURVE('',#4141,#4142,#2767,.T.);
#5365=EDGE_CURVE('',#4142,#4140,#2131,.T.);
#5366=EDGE_CURVE('',#4139,#4141,#2132,.T.);
#5367=EDGE_CURVE('',#4143,#4144,#2768,.T.);
#5368=EDGE_CURVE('',#4144,#4142,#2133,.T.);
#5369=EDGE_CURVE('',#4141,#4143,#2134,.T.);
#5370=EDGE_CURVE('',#4145,#4146,#2769,.T.);
#5371=EDGE_CURVE('',#4146,#4144,#2135,.T.);
#5372=EDGE_CURVE('',#4143,#4145,#2136,.T.);
#5373=EDGE_CURVE('',#4147,#4148,#2770,.T.);
#5374=EDGE_CURVE('',#4148,#4146,#2137,.T.);
#5375=EDGE_CURVE('',#4145,#4147,#2138,.T.);
#5376=EDGE_CURVE('',#4149,#4150,#2771,.T.);
#5377=EDGE_CURVE('',#4149,#4151,#2139,.T.);
#5378=EDGE_CURVE('',#4152,#4151,#1682,.T.);
#5379=EDGE_CURVE('',#4152,#4150,#2140,.T.);
#5380=EDGE_CURVE('',#4153,#4154,#2772,.T.);
#5381=EDGE_CURVE('',#4154,#4155,#2141,.T.);
#5382=EDGE_CURVE('',#4156,#4155,#1683,.T.);
#5383=EDGE_CURVE('',#4153,#4156,#2142,.T.);
#5384=EDGE_CURVE('',#4157,#4158,#2773,.T.);
#5385=EDGE_CURVE('',#4158,#4154,#2143,.T.);
#5386=EDGE_CURVE('',#4157,#4153,#2144,.T.);
#5387=EDGE_CURVE('',#4159,#4160,#2774,.T.);
#5388=EDGE_CURVE('',#4160,#4158,#2145,.T.);
#5389=EDGE_CURVE('',#4159,#4157,#2146,.T.);
#5390=EDGE_CURVE('',#4161,#4162,#2775,.T.);
#5391=EDGE_CURVE('',#4162,#4160,#2147,.T.);
#5392=EDGE_CURVE('',#4161,#4159,#2148,.T.);
#5393=EDGE_CURVE('',#4163,#4164,#2776,.T.);
#5394=EDGE_CURVE('',#4164,#4162,#2149,.T.);
#5395=EDGE_CURVE('',#4163,#4161,#2150,.T.);
#5396=EDGE_CURVE('',#4165,#4166,#2777,.T.);
#5397=EDGE_CURVE('',#4166,#4164,#2151,.T.);
#5398=EDGE_CURVE('',#4165,#4163,#2152,.T.);
#5399=EDGE_CURVE('',#4167,#4168,#2778,.T.);
#5400=EDGE_CURVE('',#4168,#4166,#2153,.T.);
#5401=EDGE_CURVE('',#4167,#4165,#2154,.T.);
#5402=EDGE_CURVE('',#4169,#4170,#2779,.T.);
#5403=EDGE_CURVE('',#4170,#4168,#2155,.T.);
#5404=EDGE_CURVE('',#4169,#4167,#2156,.T.);
#5405=EDGE_CURVE('',#4171,#4172,#2780,.T.);
#5406=EDGE_CURVE('',#4172,#4170,#2157,.T.);
#5407=EDGE_CURVE('',#4171,#4169,#2158,.T.);
#5408=EDGE_CURVE('',#4173,#4174,#2781,.T.);
#5409=EDGE_CURVE('',#4174,#4172,#2159,.T.);
#5410=EDGE_CURVE('',#4173,#4171,#2160,.T.);
#5411=EDGE_CURVE('',#4175,#4176,#2782,.T.);
#5412=EDGE_CURVE('',#4176,#4174,#2161,.T.);
#5413=EDGE_CURVE('',#4175,#4173,#2162,.T.);
#5414=EDGE_CURVE('',#4177,#4178,#2783,.T.);
#5415=EDGE_CURVE('',#4178,#4176,#2163,.T.);
#5416=EDGE_CURVE('',#4177,#4175,#2164,.T.);
#5417=EDGE_CURVE('',#4179,#4180,#2784,.T.);
#5418=EDGE_CURVE('',#4180,#4178,#2165,.T.);
#5419=EDGE_CURVE('',#4179,#4177,#2166,.T.);
#5420=EDGE_CURVE('',#4181,#4182,#2785,.T.);
#5421=EDGE_CURVE('',#4182,#4180,#2167,.T.);
#5422=EDGE_CURVE('',#4181,#4179,#2168,.T.);
#5423=EDGE_CURVE('',#4183,#4184,#2786,.T.);
#5424=EDGE_CURVE('',#4184,#4182,#2169,.T.);
#5425=EDGE_CURVE('',#4183,#4181,#2170,.T.);
#5426=EDGE_CURVE('',#4185,#4186,#2787,.T.);
#5427=EDGE_CURVE('',#4186,#4184,#2171,.T.);
#5428=EDGE_CURVE('',#4185,#4183,#2172,.T.);
#5429=EDGE_CURVE('',#4187,#4188,#2788,.T.);
#5430=EDGE_CURVE('',#4188,#4186,#2173,.T.);
#5431=EDGE_CURVE('',#4187,#4185,#2174,.T.);
#5432=EDGE_CURVE('',#4189,#4190,#2789,.T.);
#5433=EDGE_CURVE('',#4191,#4189,#2175,.T.);
#5434=EDGE_CURVE('',#4192,#4191,#1684,.T.);
#5435=EDGE_CURVE('',#4192,#4190,#2176,.T.);
#5436=EDGE_CURVE('',#4113,#4156,#2177,.T.);
#5437=EDGE_CURVE('',#4155,#4116,#2178,.T.);
#5438=EDGE_CURVE('',#4190,#4188,#2179,.T.);
#5439=EDGE_CURVE('',#4189,#4187,#2180,.T.);
#5440=EDGE_CURVE('',#4151,#4192,#2181,.T.);
#5441=EDGE_CURVE('',#4147,#4149,#2182,.T.);
#5442=EDGE_CURVE('',#4150,#4148,#2183,.T.);
#5443=EDGE_CURVE('',#4191,#4152,#2184,.T.);
#5444=EDGE_CURVE('',#4053,#4084,#2185,.T.);
#5445=EDGE_CURVE('',#4083,#4054,#2186,.T.);
#5446=EDGE_CURVE('',#4108,#4106,#2187,.T.);
#5447=EDGE_CURVE('',#4107,#4105,#2188,.T.);
#5448=EDGE_CURVE('',#4079,#4110,#2189,.T.);
#5449=EDGE_CURVE('',#4075,#4077,#2190,.T.);
#5450=EDGE_CURVE('',#4078,#4076,#2191,.T.);
#5451=EDGE_CURVE('',#4109,#4080,#2192,.T.);
#5452=EDGE_CURVE('',#4193,#4194,#2790,.T.);
#5453=EDGE_CURVE('',#4194,#4195,#2791,.T.);
#5454=EDGE_CURVE('',#4196,#4195,#2792,.T.);
#5455=EDGE_CURVE('',#4193,#4196,#2793,.T.);
#5456=EDGE_CURVE('',#4197,#4193,#2794,.T.);
#5457=EDGE_CURVE('',#4198,#4196,#2795,.T.);
#5458=EDGE_CURVE('',#4197,#4198,#2796,.T.);
#5459=EDGE_CURVE('',#4199,#4197,#2797,.T.);
#5460=EDGE_CURVE('',#4200,#4198,#2798,.T.);
#5461=EDGE_CURVE('',#4199,#4200,#2799,.T.);
#5462=EDGE_CURVE('',#4194,#4199,#2800,.T.);
#5463=EDGE_CURVE('',#4195,#4200,#2801,.T.);
#7366=ORIENTED_EDGE('',*,*,#5239,.T.);
#7367=ORIENTED_EDGE('',*,*,#5240,.T.);
#7368=ORIENTED_EDGE('',*,*,#5241,.T.);
#7369=ORIENTED_EDGE('',*,*,#5242,.T.);
#7370=ORIENTED_EDGE('',*,*,#5243,.T.);
#7371=ORIENTED_EDGE('',*,*,#5244,.T.);
#7372=ORIENTED_EDGE('',*,*,#5243,.F.);
#7373=ORIENTED_EDGE('',*,*,#5245,.T.);
#7374=ORIENTED_EDGE('',*,*,#5246,.T.);
#7375=ORIENTED_EDGE('',*,*,#5247,.T.);
#7376=ORIENTED_EDGE('',*,*,#5239,.F.);
#7377=ORIENTED_EDGE('',*,*,#5248,.T.);
#7378=ORIENTED_EDGE('',*,*,#5249,.T.);
#7379=ORIENTED_EDGE('',*,*,#5250,.T.);
#7380=ORIENTED_EDGE('',*,*,#5246,.F.);
#7381=ORIENTED_EDGE('',*,*,#5251,.T.);
#7382=ORIENTED_EDGE('',*,*,#5252,.T.);
#7383=ORIENTED_EDGE('',*,*,#5253,.T.);
#7384=ORIENTED_EDGE('',*,*,#5249,.F.);
#7385=ORIENTED_EDGE('',*,*,#5254,.T.);
#7386=ORIENTED_EDGE('',*,*,#5255,.T.);
#7387=ORIENTED_EDGE('',*,*,#5256,.T.);
#7388=ORIENTED_EDGE('',*,*,#5252,.F.);
#7389=ORIENTED_EDGE('',*,*,#5257,.T.);
#7390=ORIENTED_EDGE('',*,*,#5258,.T.);
#7391=ORIENTED_EDGE('',*,*,#5259,.T.);
#7392=ORIENTED_EDGE('',*,*,#5255,.F.);
#7393=ORIENTED_EDGE('',*,*,#5260,.T.);
#7394=ORIENTED_EDGE('',*,*,#5261,.T.);
#7395=ORIENTED_EDGE('',*,*,#5262,.T.);
#7396=ORIENTED_EDGE('',*,*,#5258,.F.);
#7397=ORIENTED_EDGE('',*,*,#5263,.T.);
#7398=ORIENTED_EDGE('',*,*,#5264,.T.);
#7399=ORIENTED_EDGE('',*,*,#5265,.T.);
#7400=ORIENTED_EDGE('',*,*,#5261,.F.);
#7401=ORIENTED_EDGE('',*,*,#5266,.T.);
#7402=ORIENTED_EDGE('',*,*,#5267,.T.);
#7403=ORIENTED_EDGE('',*,*,#5268,.T.);
#7404=ORIENTED_EDGE('',*,*,#5264,.F.);
#7405=ORIENTED_EDGE('',*,*,#5269,.T.);
#7406=ORIENTED_EDGE('',*,*,#5270,.T.);
#7407=ORIENTED_EDGE('',*,*,#5271,.T.);
#7408=ORIENTED_EDGE('',*,*,#5267,.F.);
#7409=ORIENTED_EDGE('',*,*,#5272,.T.);
#7410=ORIENTED_EDGE('',*,*,#5273,.T.);
#7411=ORIENTED_EDGE('',*,*,#5274,.T.);
#7412=ORIENTED_EDGE('',*,*,#5270,.F.);
#7413=ORIENTED_EDGE('',*,*,#5275,.T.);
#7414=ORIENTED_EDGE('',*,*,#5276,.F.);
#7415=ORIENTED_EDGE('',*,*,#5277,.T.);
#7416=ORIENTED_EDGE('',*,*,#5278,.F.);
#7417=ORIENTED_EDGE('',*,*,#5279,.T.);
#7418=ORIENTED_EDGE('',*,*,#5280,.T.);
#7419=ORIENTED_EDGE('',*,*,#5281,.T.);
#7420=ORIENTED_EDGE('',*,*,#5282,.F.);
#7421=ORIENTED_EDGE('',*,*,#5283,.F.);
#7422=ORIENTED_EDGE('',*,*,#5284,.T.);
#7423=ORIENTED_EDGE('',*,*,#5285,.T.);
#7424=ORIENTED_EDGE('',*,*,#5280,.F.);
#7425=ORIENTED_EDGE('',*,*,#5286,.F.);
#7426=ORIENTED_EDGE('',*,*,#5287,.T.);
#7427=ORIENTED_EDGE('',*,*,#5288,.T.);
#7428=ORIENTED_EDGE('',*,*,#5284,.F.);
#7429=ORIENTED_EDGE('',*,*,#5289,.F.);
#7430=ORIENTED_EDGE('',*,*,#5290,.T.);
#7431=ORIENTED_EDGE('',*,*,#5291,.T.);
#7432=ORIENTED_EDGE('',*,*,#5287,.F.);
#7433=ORIENTED_EDGE('',*,*,#5292,.F.);
#7434=ORIENTED_EDGE('',*,*,#5293,.T.);
#7435=ORIENTED_EDGE('',*,*,#5294,.T.);
#7436=ORIENTED_EDGE('',*,*,#5290,.F.);
#7437=ORIENTED_EDGE('',*,*,#5295,.F.);
#7438=ORIENTED_EDGE('',*,*,#5296,.T.);
#7439=ORIENTED_EDGE('',*,*,#5297,.T.);
#7440=ORIENTED_EDGE('',*,*,#5293,.F.);
#7441=ORIENTED_EDGE('',*,*,#5298,.F.);
#7442=ORIENTED_EDGE('',*,*,#5299,.T.);
#7443=ORIENTED_EDGE('',*,*,#5300,.T.);
#7444=ORIENTED_EDGE('',*,*,#5296,.F.);
#7445=ORIENTED_EDGE('',*,*,#5301,.F.);
#7446=ORIENTED_EDGE('',*,*,#5302,.T.);
#7447=ORIENTED_EDGE('',*,*,#5303,.T.);
#7448=ORIENTED_EDGE('',*,*,#5299,.F.);
#7449=ORIENTED_EDGE('',*,*,#5304,.F.);
#7450=ORIENTED_EDGE('',*,*,#5305,.T.);
#7451=ORIENTED_EDGE('',*,*,#5306,.T.);
#7452=ORIENTED_EDGE('',*,*,#5302,.F.);
#7453=ORIENTED_EDGE('',*,*,#5307,.F.);
#7454=ORIENTED_EDGE('',*,*,#5308,.T.);
#7455=ORIENTED_EDGE('',*,*,#5309,.T.);
#7456=ORIENTED_EDGE('',*,*,#5305,.F.);
#7457=ORIENTED_EDGE('',*,*,#5310,.F.);
#7458=ORIENTED_EDGE('',*,*,#5311,.T.);
#7459=ORIENTED_EDGE('',*,*,#5312,.T.);
#7460=ORIENTED_EDGE('',*,*,#5308,.F.);
#7461=ORIENTED_EDGE('',*,*,#5313,.F.);
#7462=ORIENTED_EDGE('',*,*,#5314,.T.);
#7463=ORIENTED_EDGE('',*,*,#5315,.T.);
#7464=ORIENTED_EDGE('',*,*,#5311,.F.);
#7465=ORIENTED_EDGE('',*,*,#5316,.F.);
#7466=ORIENTED_EDGE('',*,*,#5317,.F.);
#7467=ORIENTED_EDGE('',*,*,#5318,.F.);
#7468=ORIENTED_EDGE('',*,*,#5319,.F.);
#7469=ORIENTED_EDGE('',*,*,#5320,.T.);
#7470=ORIENTED_EDGE('',*,*,#5321,.T.);
#7471=ORIENTED_EDGE('',*,*,#5322,.T.);
#7472=ORIENTED_EDGE('',*,*,#5323,.T.);
#7473=ORIENTED_EDGE('',*,*,#5324,.T.);
#7474=ORIENTED_EDGE('',*,*,#5325,.T.);
#7475=ORIENTED_EDGE('',*,*,#5324,.F.);
#7476=ORIENTED_EDGE('',*,*,#5326,.T.);
#7477=ORIENTED_EDGE('',*,*,#5327,.T.);
#7478=ORIENTED_EDGE('',*,*,#5328,.T.);
#7479=ORIENTED_EDGE('',*,*,#5329,.T.);
#7480=ORIENTED_EDGE('',*,*,#5321,.F.);
#7481=ORIENTED_EDGE('',*,*,#5330,.T.);
#7482=ORIENTED_EDGE('',*,*,#5331,.T.);
#7483=ORIENTED_EDGE('',*,*,#5332,.T.);
#7484=ORIENTED_EDGE('',*,*,#5328,.F.);
#7485=ORIENTED_EDGE('',*,*,#5333,.T.);
#7486=ORIENTED_EDGE('',*,*,#5334,.T.);
#7487=ORIENTED_EDGE('',*,*,#5335,.T.);
#7488=ORIENTED_EDGE('',*,*,#5331,.F.);
#7489=ORIENTED_EDGE('',*,*,#5336,.T.);
#7490=ORIENTED_EDGE('',*,*,#5337,.T.);
#7491=ORIENTED_EDGE('',*,*,#5338,.T.);
#7492=ORIENTED_EDGE('',*,*,#5334,.F.);
#7493=ORIENTED_EDGE('',*,*,#5339,.T.);
#7494=ORIENTED_EDGE('',*,*,#5340,.T.);
#7495=ORIENTED_EDGE('',*,*,#5341,.T.);
#7496=ORIENTED_EDGE('',*,*,#5337,.F.);
#7497=ORIENTED_EDGE('',*,*,#5342,.T.);
#7498=ORIENTED_EDGE('',*,*,#5343,.T.);
#7499=ORIENTED_EDGE('',*,*,#5344,.T.);
#7500=ORIENTED_EDGE('',*,*,#5340,.F.);
#7501=ORIENTED_EDGE('',*,*,#5345,.T.);
#7502=ORIENTED_EDGE('',*,*,#5346,.T.);
#7503=ORIENTED_EDGE('',*,*,#5347,.T.);
#7504=ORIENTED_EDGE('',*,*,#5343,.F.);
#7505=ORIENTED_EDGE('',*,*,#5348,.T.);
#7506=ORIENTED_EDGE('',*,*,#5349,.T.);
#7507=ORIENTED_EDGE('',*,*,#5350,.T.);
#7508=ORIENTED_EDGE('',*,*,#5346,.F.);
#7509=ORIENTED_EDGE('',*,*,#5351,.T.);
#7510=ORIENTED_EDGE('',*,*,#5352,.T.);
#7511=ORIENTED_EDGE('',*,*,#5353,.T.);
#7512=ORIENTED_EDGE('',*,*,#5349,.F.);
#7513=ORIENTED_EDGE('',*,*,#5354,.T.);
#7514=ORIENTED_EDGE('',*,*,#5355,.T.);
#7515=ORIENTED_EDGE('',*,*,#5356,.T.);
#7516=ORIENTED_EDGE('',*,*,#5352,.F.);
#7517=ORIENTED_EDGE('',*,*,#5357,.T.);
#7518=ORIENTED_EDGE('',*,*,#5358,.T.);
#7519=ORIENTED_EDGE('',*,*,#5359,.T.);
#7520=ORIENTED_EDGE('',*,*,#5355,.F.);
#7521=ORIENTED_EDGE('',*,*,#5360,.T.);
#7522=ORIENTED_EDGE('',*,*,#5361,.T.);
#7523=ORIENTED_EDGE('',*,*,#5362,.T.);
#7524=ORIENTED_EDGE('',*,*,#5358,.F.);
#7525=ORIENTED_EDGE('',*,*,#5363,.T.);
#7526=ORIENTED_EDGE('',*,*,#5364,.T.);
#7527=ORIENTED_EDGE('',*,*,#5365,.T.);
#7528=ORIENTED_EDGE('',*,*,#5361,.F.);
#7529=ORIENTED_EDGE('',*,*,#5366,.T.);
#7530=ORIENTED_EDGE('',*,*,#5367,.T.);
#7531=ORIENTED_EDGE('',*,*,#5368,.T.);
#7532=ORIENTED_EDGE('',*,*,#5364,.F.);
#7533=ORIENTED_EDGE('',*,*,#5369,.T.);
#7534=ORIENTED_EDGE('',*,*,#5370,.T.);
#7535=ORIENTED_EDGE('',*,*,#5371,.T.);
#7536=ORIENTED_EDGE('',*,*,#5367,.F.);
#7537=ORIENTED_EDGE('',*,*,#5372,.T.);
#7538=ORIENTED_EDGE('',*,*,#5373,.T.);
#7539=ORIENTED_EDGE('',*,*,#5374,.T.);
#7540=ORIENTED_EDGE('',*,*,#5370,.F.);
#7541=ORIENTED_EDGE('',*,*,#5375,.T.);
#7542=ORIENTED_EDGE('',*,*,#5376,.F.);
#7543=ORIENTED_EDGE('',*,*,#5377,.T.);
#7544=ORIENTED_EDGE('',*,*,#5378,.F.);
#7545=ORIENTED_EDGE('',*,*,#5379,.T.);
#7546=ORIENTED_EDGE('',*,*,#5380,.T.);
#7547=ORIENTED_EDGE('',*,*,#5381,.T.);
#7548=ORIENTED_EDGE('',*,*,#5382,.F.);
#7549=ORIENTED_EDGE('',*,*,#5383,.F.);
#7550=ORIENTED_EDGE('',*,*,#5384,.T.);
#7551=ORIENTED_EDGE('',*,*,#5385,.T.);
#7552=ORIENTED_EDGE('',*,*,#5380,.F.);
#7553=ORIENTED_EDGE('',*,*,#5386,.F.);
#7554=ORIENTED_EDGE('',*,*,#5387,.T.);
#7555=ORIENTED_EDGE('',*,*,#5388,.T.);
#7556=ORIENTED_EDGE('',*,*,#5384,.F.);
#7557=ORIENTED_EDGE('',*,*,#5389,.F.);
#7558=ORIENTED_EDGE('',*,*,#5390,.T.);
#7559=ORIENTED_EDGE('',*,*,#5391,.T.);
#7560=ORIENTED_EDGE('',*,*,#5387,.F.);
#7561=ORIENTED_EDGE('',*,*,#5392,.F.);
#7562=ORIENTED_EDGE('',*,*,#5393,.T.);
#7563=ORIENTED_EDGE('',*,*,#5394,.T.);
#7564=ORIENTED_EDGE('',*,*,#5390,.F.);
#7565=ORIENTED_EDGE('',*,*,#5395,.F.);
#7566=ORIENTED_EDGE('',*,*,#5396,.T.);
#7567=ORIENTED_EDGE('',*,*,#5397,.T.);
#7568=ORIENTED_EDGE('',*,*,#5393,.F.);
#7569=ORIENTED_EDGE('',*,*,#5398,.F.);
#7570=ORIENTED_EDGE('',*,*,#5399,.T.);
#7571=ORIENTED_EDGE('',*,*,#5400,.T.);
#7572=ORIENTED_EDGE('',*,*,#5396,.F.);
#7573=ORIENTED_EDGE('',*,*,#5401,.F.);
#7574=ORIENTED_EDGE('',*,*,#5402,.T.);
#7575=ORIENTED_EDGE('',*,*,#5403,.T.);
#7576=ORIENTED_EDGE('',*,*,#5399,.F.);
#7577=ORIENTED_EDGE('',*,*,#5404,.F.);
#7578=ORIENTED_EDGE('',*,*,#5405,.T.);
#7579=ORIENTED_EDGE('',*,*,#5406,.T.);
#7580=ORIENTED_EDGE('',*,*,#5402,.F.);
#7581=ORIENTED_EDGE('',*,*,#5407,.F.);
#7582=ORIENTED_EDGE('',*,*,#5408,.T.);
#7583=ORIENTED_EDGE('',*,*,#5409,.T.);
#7584=ORIENTED_EDGE('',*,*,#5405,.F.);
#7585=ORIENTED_EDGE('',*,*,#5410,.F.);
#7586=ORIENTED_EDGE('',*,*,#5411,.T.);
#7587=ORIENTED_EDGE('',*,*,#5412,.T.);
#7588=ORIENTED_EDGE('',*,*,#5408,.F.);
#7589=ORIENTED_EDGE('',*,*,#5413,.F.);
#7590=ORIENTED_EDGE('',*,*,#5414,.T.);
#7591=ORIENTED_EDGE('',*,*,#5415,.T.);
#7592=ORIENTED_EDGE('',*,*,#5411,.F.);
#7593=ORIENTED_EDGE('',*,*,#5416,.F.);
#7594=ORIENTED_EDGE('',*,*,#5417,.T.);
#7595=ORIENTED_EDGE('',*,*,#5418,.T.);
#7596=ORIENTED_EDGE('',*,*,#5414,.F.);
#7597=ORIENTED_EDGE('',*,*,#5419,.F.);
#7598=ORIENTED_EDGE('',*,*,#5420,.T.);
#7599=ORIENTED_EDGE('',*,*,#5421,.T.);
#7600=ORIENTED_EDGE('',*,*,#5417,.F.);
#7601=ORIENTED_EDGE('',*,*,#5422,.F.);
#7602=ORIENTED_EDGE('',*,*,#5423,.T.);
#7603=ORIENTED_EDGE('',*,*,#5424,.T.);
#7604=ORIENTED_EDGE('',*,*,#5420,.F.);
#7605=ORIENTED_EDGE('',*,*,#5425,.F.);
#7606=ORIENTED_EDGE('',*,*,#5426,.T.);
#7607=ORIENTED_EDGE('',*,*,#5427,.T.);
#7608=ORIENTED_EDGE('',*,*,#5423,.F.);
#7609=ORIENTED_EDGE('',*,*,#5428,.F.);
#7610=ORIENTED_EDGE('',*,*,#5429,.T.);
#7611=ORIENTED_EDGE('',*,*,#5430,.T.);
#7612=ORIENTED_EDGE('',*,*,#5426,.F.);
#7613=ORIENTED_EDGE('',*,*,#5431,.F.);
#7614=ORIENTED_EDGE('',*,*,#5432,.F.);
#7615=ORIENTED_EDGE('',*,*,#5433,.F.);
#7616=ORIENTED_EDGE('',*,*,#5434,.F.);
#7617=ORIENTED_EDGE('',*,*,#5435,.T.);
#7618=ORIENTED_EDGE('',*,*,#5323,.F.);
#7619=ORIENTED_EDGE('',*,*,#5436,.T.);
#7620=ORIENTED_EDGE('',*,*,#5382,.T.);
#7621=ORIENTED_EDGE('',*,*,#5437,.T.);
#7622=ORIENTED_EDGE('',*,*,#5326,.F.);
#7623=ORIENTED_EDGE('',*,*,#5432,.T.);
#7624=ORIENTED_EDGE('',*,*,#5438,.T.);
#7625=ORIENTED_EDGE('',*,*,#5429,.F.);
#7626=ORIENTED_EDGE('',*,*,#5439,.F.);
#7627=ORIENTED_EDGE('',*,*,#5437,.F.);
#7628=ORIENTED_EDGE('',*,*,#5381,.F.);
#7629=ORIENTED_EDGE('',*,*,#5385,.F.);
#7630=ORIENTED_EDGE('',*,*,#5388,.F.);
#7631=ORIENTED_EDGE('',*,*,#5391,.F.);
#7632=ORIENTED_EDGE('',*,*,#5394,.F.);
#7633=ORIENTED_EDGE('',*,*,#5397,.F.);
#7634=ORIENTED_EDGE('',*,*,#5400,.F.);
#7635=ORIENTED_EDGE('',*,*,#5403,.F.);
#7636=ORIENTED_EDGE('',*,*,#5406,.F.);
#7637=ORIENTED_EDGE('',*,*,#5409,.F.);
#7638=ORIENTED_EDGE('',*,*,#5412,.F.);
#7639=ORIENTED_EDGE('',*,*,#5415,.F.);
#7640=ORIENTED_EDGE('',*,*,#5418,.F.);
#7641=ORIENTED_EDGE('',*,*,#5421,.F.);
#7642=ORIENTED_EDGE('',*,*,#5424,.F.);
#7643=ORIENTED_EDGE('',*,*,#5427,.F.);
#7644=ORIENTED_EDGE('',*,*,#5430,.F.);
#7645=ORIENTED_EDGE('',*,*,#5438,.F.);
#7646=ORIENTED_EDGE('',*,*,#5435,.F.);
#7647=ORIENTED_EDGE('',*,*,#5440,.F.);
#7648=ORIENTED_EDGE('',*,*,#5377,.F.);
#7649=ORIENTED_EDGE('',*,*,#5441,.F.);
#7650=ORIENTED_EDGE('',*,*,#5375,.F.);
#7651=ORIENTED_EDGE('',*,*,#5372,.F.);
#7652=ORIENTED_EDGE('',*,*,#5369,.F.);
#7653=ORIENTED_EDGE('',*,*,#5366,.F.);
#7654=ORIENTED_EDGE('',*,*,#5363,.F.);
#7655=ORIENTED_EDGE('',*,*,#5360,.F.);
#7656=ORIENTED_EDGE('',*,*,#5357,.F.);
#7657=ORIENTED_EDGE('',*,*,#5354,.F.);
#7658=ORIENTED_EDGE('',*,*,#5351,.F.);
#7659=ORIENTED_EDGE('',*,*,#5348,.F.);
#7660=ORIENTED_EDGE('',*,*,#5345,.F.);
#7661=ORIENTED_EDGE('',*,*,#5342,.F.);
#7662=ORIENTED_EDGE('',*,*,#5339,.F.);
#7663=ORIENTED_EDGE('',*,*,#5336,.F.);
#7664=ORIENTED_EDGE('',*,*,#5333,.F.);
#7665=ORIENTED_EDGE('',*,*,#5330,.F.);
#7666=ORIENTED_EDGE('',*,*,#5327,.F.);
#7667=ORIENTED_EDGE('',*,*,#5436,.F.);
#7668=ORIENTED_EDGE('',*,*,#5322,.F.);
#7669=ORIENTED_EDGE('',*,*,#5329,.F.);
#7670=ORIENTED_EDGE('',*,*,#5332,.F.);
#7671=ORIENTED_EDGE('',*,*,#5335,.F.);
#7672=ORIENTED_EDGE('',*,*,#5338,.F.);
#7673=ORIENTED_EDGE('',*,*,#5341,.F.);
#7674=ORIENTED_EDGE('',*,*,#5344,.F.);
#7675=ORIENTED_EDGE('',*,*,#5347,.F.);
#7676=ORIENTED_EDGE('',*,*,#5350,.F.);
#7677=ORIENTED_EDGE('',*,*,#5353,.F.);
#7678=ORIENTED_EDGE('',*,*,#5356,.F.);
#7679=ORIENTED_EDGE('',*,*,#5359,.F.);
#7680=ORIENTED_EDGE('',*,*,#5362,.F.);
#7681=ORIENTED_EDGE('',*,*,#5365,.F.);
#7682=ORIENTED_EDGE('',*,*,#5368,.F.);
#7683=ORIENTED_EDGE('',*,*,#5371,.F.);
#7684=ORIENTED_EDGE('',*,*,#5374,.F.);
#7685=ORIENTED_EDGE('',*,*,#5442,.F.);
#7686=ORIENTED_EDGE('',*,*,#5379,.F.);
#7687=ORIENTED_EDGE('',*,*,#5443,.F.);
#7688=ORIENTED_EDGE('',*,*,#5433,.T.);
#7689=ORIENTED_EDGE('',*,*,#5439,.T.);
#7690=ORIENTED_EDGE('',*,*,#5431,.T.);
#7691=ORIENTED_EDGE('',*,*,#5428,.T.);
#7692=ORIENTED_EDGE('',*,*,#5425,.T.);
#7693=ORIENTED_EDGE('',*,*,#5422,.T.);
#7694=ORIENTED_EDGE('',*,*,#5419,.T.);
#7695=ORIENTED_EDGE('',*,*,#5416,.T.);
#7696=ORIENTED_EDGE('',*,*,#5413,.T.);
#7697=ORIENTED_EDGE('',*,*,#5410,.T.);
#7698=ORIENTED_EDGE('',*,*,#5407,.T.);
#7699=ORIENTED_EDGE('',*,*,#5404,.T.);
#7700=ORIENTED_EDGE('',*,*,#5401,.T.);
#7701=ORIENTED_EDGE('',*,*,#5398,.T.);
#7702=ORIENTED_EDGE('',*,*,#5395,.T.);
#7703=ORIENTED_EDGE('',*,*,#5392,.T.);
#7704=ORIENTED_EDGE('',*,*,#5389,.T.);
#7705=ORIENTED_EDGE('',*,*,#5386,.T.);
#7706=ORIENTED_EDGE('',*,*,#5383,.T.);
#7707=ORIENTED_EDGE('',*,*,#5376,.T.);
#7708=ORIENTED_EDGE('',*,*,#5442,.T.);
#7709=ORIENTED_EDGE('',*,*,#5373,.F.);
#7710=ORIENTED_EDGE('',*,*,#5441,.T.);
#7711=ORIENTED_EDGE('',*,*,#5325,.F.);
#7712=ORIENTED_EDGE('',*,*,#5241,.F.);
#7713=ORIENTED_EDGE('',*,*,#5444,.T.);
#7714=ORIENTED_EDGE('',*,*,#5282,.T.);
#7715=ORIENTED_EDGE('',*,*,#5445,.T.);
#7716=ORIENTED_EDGE('',*,*,#5317,.T.);
#7717=ORIENTED_EDGE('',*,*,#5446,.T.);
#7718=ORIENTED_EDGE('',*,*,#5314,.F.);
#7719=ORIENTED_EDGE('',*,*,#5447,.F.);
#7720=ORIENTED_EDGE('',*,*,#5445,.F.);
#7721=ORIENTED_EDGE('',*,*,#5281,.F.);
#7722=ORIENTED_EDGE('',*,*,#5285,.F.);
#7723=ORIENTED_EDGE('',*,*,#5288,.F.);
#7724=ORIENTED_EDGE('',*,*,#5291,.F.);
#7725=ORIENTED_EDGE('',*,*,#5294,.F.);
#7726=ORIENTED_EDGE('',*,*,#5297,.F.);
#7727=ORIENTED_EDGE('',*,*,#5300,.F.);
#7728=ORIENTED_EDGE('',*,*,#5303,.F.);
#7729=ORIENTED_EDGE('',*,*,#5306,.F.);
#7730=ORIENTED_EDGE('',*,*,#5309,.F.);
#7731=ORIENTED_EDGE('',*,*,#5312,.F.);
#7732=ORIENTED_EDGE('',*,*,#5315,.F.);
#7733=ORIENTED_EDGE('',*,*,#5446,.F.);
#7734=ORIENTED_EDGE('',*,*,#5320,.F.);
#7735=ORIENTED_EDGE('',*,*,#5448,.F.);
#7736=ORIENTED_EDGE('',*,*,#5277,.F.);
#7737=ORIENTED_EDGE('',*,*,#5449,.F.);
#7738=ORIENTED_EDGE('',*,*,#5275,.F.);
#7739=ORIENTED_EDGE('',*,*,#5272,.F.);
#7740=ORIENTED_EDGE('',*,*,#5269,.F.);
#7741=ORIENTED_EDGE('',*,*,#5266,.F.);
#7742=ORIENTED_EDGE('',*,*,#5263,.F.);
#7743=ORIENTED_EDGE('',*,*,#5260,.F.);
#7744=ORIENTED_EDGE('',*,*,#5257,.F.);
#7745=ORIENTED_EDGE('',*,*,#5254,.F.);
#7746=ORIENTED_EDGE('',*,*,#5251,.F.);
#7747=ORIENTED_EDGE('',*,*,#5248,.F.);
#7748=ORIENTED_EDGE('',*,*,#5245,.F.);
#7749=ORIENTED_EDGE('',*,*,#5242,.F.);
#7750=ORIENTED_EDGE('',*,*,#5444,.F.);
#7751=ORIENTED_EDGE('',*,*,#5240,.F.);
#7752=ORIENTED_EDGE('',*,*,#5247,.F.);
#7753=ORIENTED_EDGE('',*,*,#5250,.F.);
#7754=ORIENTED_EDGE('',*,*,#5253,.F.);
#7755=ORIENTED_EDGE('',*,*,#5256,.F.);
#7756=ORIENTED_EDGE('',*,*,#5259,.F.);
#7757=ORIENTED_EDGE('',*,*,#5262,.F.);
#7758=ORIENTED_EDGE('',*,*,#5265,.F.);
#7759=ORIENTED_EDGE('',*,*,#5268,.F.);
#7760=ORIENTED_EDGE('',*,*,#5271,.F.);
#7761=ORIENTED_EDGE('',*,*,#5274,.F.);
#7762=ORIENTED_EDGE('',*,*,#5450,.F.);
#7763=ORIENTED_EDGE('',*,*,#5279,.F.);
#7764=ORIENTED_EDGE('',*,*,#5451,.F.);
#7765=ORIENTED_EDGE('',*,*,#5318,.T.);
#7766=ORIENTED_EDGE('',*,*,#5447,.T.);
#7767=ORIENTED_EDGE('',*,*,#5316,.T.);
#7768=ORIENTED_EDGE('',*,*,#5313,.T.);
#7769=ORIENTED_EDGE('',*,*,#5310,.T.);
#7770=ORIENTED_EDGE('',*,*,#5307,.T.);
#7771=ORIENTED_EDGE('',*,*,#5304,.T.);
#7772=ORIENTED_EDGE('',*,*,#5301,.T.);
#7773=ORIENTED_EDGE('',*,*,#5298,.T.);
#7774=ORIENTED_EDGE('',*,*,#5295,.T.);
#7775=ORIENTED_EDGE('',*,*,#5292,.T.);
#7776=ORIENTED_EDGE('',*,*,#5289,.T.);
#7777=ORIENTED_EDGE('',*,*,#5286,.T.);
#7778=ORIENTED_EDGE('',*,*,#5283,.T.);
#7779=ORIENTED_EDGE('',*,*,#5276,.T.);
#7780=ORIENTED_EDGE('',*,*,#5450,.T.);
#7781=ORIENTED_EDGE('',*,*,#5273,.F.);
#7782=ORIENTED_EDGE('',*,*,#5449,.T.);
#7783=ORIENTED_EDGE('',*,*,#5244,.F.);
#7784=ORIENTED_EDGE('',*,*,#5452,.T.);
#7785=ORIENTED_EDGE('',*,*,#5453,.T.);
#7786=ORIENTED_EDGE('',*,*,#5454,.F.);
#7787=ORIENTED_EDGE('',*,*,#5455,.F.);
#7788=ORIENTED_EDGE('',*,*,#5456,.T.);
#7789=ORIENTED_EDGE('',*,*,#5455,.T.);
#7790=ORIENTED_EDGE('',*,*,#5457,.F.);
#7791=ORIENTED_EDGE('',*,*,#5458,.F.);
#7792=ORIENTED_EDGE('',*,*,#5459,.T.);
#7793=ORIENTED_EDGE('',*,*,#5458,.T.);
#7794=ORIENTED_EDGE('',*,*,#5460,.F.);
#7795=ORIENTED_EDGE('',*,*,#5461,.F.);
#7796=ORIENTED_EDGE('',*,*,#5462,.T.);
#7797=ORIENTED_EDGE('',*,*,#5461,.T.);
#7798=ORIENTED_EDGE('',*,*,#5463,.F.);
#7799=ORIENTED_EDGE('',*,*,#5453,.F.);
#7800=ORIENTED_EDGE('',*,*,#5463,.T.);
#7801=ORIENTED_EDGE('',*,*,#5460,.T.);
#7802=ORIENTED_EDGE('',*,*,#5457,.T.);
#7803=ORIENTED_EDGE('',*,*,#5454,.T.);
#7804=ORIENTED_EDGE('',*,*,#5443,.T.);
#7805=ORIENTED_EDGE('',*,*,#5378,.T.);
#7806=ORIENTED_EDGE('',*,*,#5440,.T.);
#7807=ORIENTED_EDGE('',*,*,#5434,.T.);
#7808=ORIENTED_EDGE('',*,*,#5462,.F.);
#7809=ORIENTED_EDGE('',*,*,#5452,.F.);
#7810=ORIENTED_EDGE('',*,*,#5456,.F.);
#7811=ORIENTED_EDGE('',*,*,#5459,.F.);
#7812=ORIENTED_EDGE('',*,*,#5451,.T.);
#7813=ORIENTED_EDGE('',*,*,#5278,.T.);
#7814=ORIENTED_EDGE('',*,*,#5448,.T.);
#7815=ORIENTED_EDGE('',*,*,#5319,.T.);
#9033=CYLINDRICAL_SURFACE('',#10315,0.1666);
#9034=CYLINDRICAL_SURFACE('',#10318,0.1666);
#9035=CYLINDRICAL_SURFACE('',#10319,0.1666);
#9036=CYLINDRICAL_SURFACE('',#10320,0.1666);
#9037=CYLINDRICAL_SURFACE('',#10321,0.1666);
#9038=CYLINDRICAL_SURFACE('',#10322,0.1666);
#9039=CYLINDRICAL_SURFACE('',#10323,0.1666);
#9040=CYLINDRICAL_SURFACE('',#10324,0.1666);
#9041=CYLINDRICAL_SURFACE('',#10325,0.1666);
#9042=CYLINDRICAL_SURFACE('',#10326,0.1666);
#9043=CYLINDRICAL_SURFACE('',#10327,0.1666);
#9044=CYLINDRICAL_SURFACE('',#10328,0.1666);
#9045=CYLINDRICAL_SURFACE('',#10330,0.205475);
#9046=CYLINDRICAL_SURFACE('',#10332,0.205475);
#9047=CYLINDRICAL_SURFACE('',#10333,0.205475);
#9048=CYLINDRICAL_SURFACE('',#10334,0.205475);
#9049=CYLINDRICAL_SURFACE('',#10335,0.205475);
#9050=CYLINDRICAL_SURFACE('',#10336,0.205475);
#9051=CYLINDRICAL_SURFACE('',#10337,0.205475);
#9052=CYLINDRICAL_SURFACE('',#10338,0.205475);
#9053=CYLINDRICAL_SURFACE('',#10339,0.205475);
#9054=CYLINDRICAL_SURFACE('',#10340,0.205475);
#9055=CYLINDRICAL_SURFACE('',#10341,0.205475);
#9056=CYLINDRICAL_SURFACE('',#10342,0.205475);
#9057=CYLINDRICAL_SURFACE('',#10343,0.205475);
#9058=CYLINDRICAL_SURFACE('',#10345,0.12645);
#9059=CYLINDRICAL_SURFACE('',#10349,0.12645);
#9060=CYLINDRICAL_SURFACE('',#10350,0.12645);
#9061=CYLINDRICAL_SURFACE('',#10351,0.12645);
#9062=CYLINDRICAL_SURFACE('',#10352,0.12645);
#9063=CYLINDRICAL_SURFACE('',#10353,0.12645);
#9064=CYLINDRICAL_SURFACE('',#10354,0.12645);
#9065=CYLINDRICAL_SURFACE('',#10355,0.12645);
#9066=CYLINDRICAL_SURFACE('',#10356,0.12645);
#9067=CYLINDRICAL_SURFACE('',#10357,0.12645);
#9068=CYLINDRICAL_SURFACE('',#10358,0.12645);
#9069=CYLINDRICAL_SURFACE('',#10359,0.12645);
#9070=CYLINDRICAL_SURFACE('',#10360,0.12645);
#9071=CYLINDRICAL_SURFACE('',#10361,0.12645);
#9072=CYLINDRICAL_SURFACE('',#10362,0.12645);
#9073=CYLINDRICAL_SURFACE('',#10363,0.12645);
#9074=CYLINDRICAL_SURFACE('',#10364,0.12645);
#9075=CYLINDRICAL_SURFACE('',#10365,0.12645);
#9076=CYLINDRICAL_SURFACE('',#10367,0.1543);
#9077=CYLINDRICAL_SURFACE('',#10369,0.1543);
#9078=CYLINDRICAL_SURFACE('',#10370,0.1543);
#9079=CYLINDRICAL_SURFACE('',#10371,0.1543);
#9080=CYLINDRICAL_SURFACE('',#10372,0.1543);
#9081=CYLINDRICAL_SURFACE('',#10373,0.1543);
#9082=CYLINDRICAL_SURFACE('',#10374,0.1543);
#9083=CYLINDRICAL_SURFACE('',#10375,0.1543);
#9084=CYLINDRICAL_SURFACE('',#10376,0.1543);
#9085=CYLINDRICAL_SURFACE('',#10377,0.1543);
#9086=CYLINDRICAL_SURFACE('',#10378,0.1543);
#9087=CYLINDRICAL_SURFACE('',#10379,0.1543);
#9088=CYLINDRICAL_SURFACE('',#10380,0.1543);
#9089=CYLINDRICAL_SURFACE('',#10381,0.1543);
#9090=CYLINDRICAL_SURFACE('',#10382,0.1543);
#9091=CYLINDRICAL_SURFACE('',#10383,0.1543);
#9092=CYLINDRICAL_SURFACE('',#10384,0.1543);
#9093=CYLINDRICAL_SURFACE('',#10385,0.1543);
#9094=CYLINDRICAL_SURFACE('',#10388,0.1543);
#9095=CYLINDRICAL_SURFACE('',#10389,0.12645);
#9096=CYLINDRICAL_SURFACE('',#10392,0.205475);
#9097=CYLINDRICAL_SURFACE('',#10393,0.1666);
#9484=ADVANCED_FACE('',(#694),#9033,.F.);
#9485=ADVANCED_FACE('',(#695),#9034,.F.);
#9486=ADVANCED_FACE('',(#696),#9035,.F.);
#9487=ADVANCED_FACE('',(#697),#9036,.F.);
#9488=ADVANCED_FACE('',(#698),#9037,.F.);
#9489=ADVANCED_FACE('',(#699),#9038,.F.);
#9490=ADVANCED_FACE('',(#700),#9039,.F.);
#9491=ADVANCED_FACE('',(#701),#9040,.F.);
#9492=ADVANCED_FACE('',(#702),#9041,.F.);
#9493=ADVANCED_FACE('',(#703),#9042,.F.);
#9494=ADVANCED_FACE('',(#704),#9043,.F.);
#9495=ADVANCED_FACE('',(#705),#9044,.F.);
#9496=ADVANCED_FACE('',(#706),#9045,.F.);
#9497=ADVANCED_FACE('',(#707),#9046,.F.);
#9498=ADVANCED_FACE('',(#708),#9047,.F.);
#9499=ADVANCED_FACE('',(#709),#9048,.F.);
#9500=ADVANCED_FACE('',(#710),#9049,.F.);
#9501=ADVANCED_FACE('',(#711),#9050,.F.);
#9502=ADVANCED_FACE('',(#712),#9051,.F.);
#9503=ADVANCED_FACE('',(#713),#9052,.F.);
#9504=ADVANCED_FACE('',(#714),#9053,.F.);
#9505=ADVANCED_FACE('',(#715),#9054,.F.);
#9506=ADVANCED_FACE('',(#716),#9055,.F.);
#9507=ADVANCED_FACE('',(#717),#9056,.F.);
#9508=ADVANCED_FACE('',(#718),#9057,.F.);
#9509=ADVANCED_FACE('',(#719),#9058,.F.);
#9510=ADVANCED_FACE('',(#720),#9059,.F.);
#9511=ADVANCED_FACE('',(#721),#9060,.F.);
#9512=ADVANCED_FACE('',(#722),#9061,.F.);
#9513=ADVANCED_FACE('',(#723),#9062,.F.);
#9514=ADVANCED_FACE('',(#724),#9063,.F.);
#9515=ADVANCED_FACE('',(#725),#9064,.F.);
#9516=ADVANCED_FACE('',(#726),#9065,.F.);
#9517=ADVANCED_FACE('',(#727),#9066,.F.);
#9518=ADVANCED_FACE('',(#728),#9067,.F.);
#9519=ADVANCED_FACE('',(#729),#9068,.F.);
#9520=ADVANCED_FACE('',(#730),#9069,.F.);
#9521=ADVANCED_FACE('',(#731),#9070,.F.);
#9522=ADVANCED_FACE('',(#732),#9071,.F.);
#9523=ADVANCED_FACE('',(#733),#9072,.F.);
#9524=ADVANCED_FACE('',(#734),#9073,.F.);
#9525=ADVANCED_FACE('',(#735),#9074,.F.);
#9526=ADVANCED_FACE('',(#736),#9075,.F.);
#9527=ADVANCED_FACE('',(#737),#9076,.F.);
#9528=ADVANCED_FACE('',(#738),#9077,.F.);
#9529=ADVANCED_FACE('',(#739),#9078,.F.);
#9530=ADVANCED_FACE('',(#740),#9079,.F.);
#9531=ADVANCED_FACE('',(#741),#9080,.F.);
#9532=ADVANCED_FACE('',(#742),#9081,.F.);
#9533=ADVANCED_FACE('',(#743),#9082,.F.);
#9534=ADVANCED_FACE('',(#744),#9083,.F.);
#9535=ADVANCED_FACE('',(#745),#9084,.F.);
#9536=ADVANCED_FACE('',(#746),#9085,.F.);
#9537=ADVANCED_FACE('',(#747),#9086,.F.);
#9538=ADVANCED_FACE('',(#748),#9087,.F.);
#9539=ADVANCED_FACE('',(#749),#9088,.F.);
#9540=ADVANCED_FACE('',(#750),#9089,.F.);
#9541=ADVANCED_FACE('',(#751),#9090,.F.);
#9542=ADVANCED_FACE('',(#752),#9091,.F.);
#9543=ADVANCED_FACE('',(#753),#9092,.F.);
#9544=ADVANCED_FACE('',(#754),#9093,.F.);
#9545=ADVANCED_FACE('',(#755),#368,.T.);
#9546=ADVANCED_FACE('',(#756),#9094,.F.);
#9547=ADVANCED_FACE('',(#757),#222,.F.);
#9548=ADVANCED_FACE('',(#758),#223,.F.);
#9549=ADVANCED_FACE('',(#759),#9095,.F.);
#9550=ADVANCED_FACE('',(#760),#369,.F.);
#9551=ADVANCED_FACE('',(#761),#370,.F.);
#9552=ADVANCED_FACE('',(#762),#9096,.F.);
#9553=ADVANCED_FACE('',(#763),#224,.F.);
#9554=ADVANCED_FACE('',(#764),#225,.F.);
#9555=ADVANCED_FACE('',(#765),#9097,.F.);
#9556=ADVANCED_FACE('',(#766),#371,.F.);
#9557=ADVANCED_FACE('',(#767),#372,.T.);
#9558=ADVANCED_FACE('',(#768),#373,.T.);
#9559=ADVANCED_FACE('',(#769),#374,.T.);
#9560=ADVANCED_FACE('',(#770),#375,.T.);
#9561=ADVANCED_FACE('',(#771,#282),#376,.T.);
#9562=ADVANCED_FACE('',(#772,#283),#377,.F.);
#9773=CLOSED_SHELL('',(#9484,#9485,#9486,#9487,#9488,#9489,#9490,#9491,
#9492,#9493,#9494,#9495,#9496,#9497,#9498,#9499,#9500,#9501,#9502,#9503,
#9504,#9505,#9506,#9507,#9508,#9509,#9510,#9511,#9512,#9513,#9514,#9515,
#9516,#9517,#9518,#9519,#9520,#9521,#9522,#9523,#9524,#9525,#9526,#9527,
#9528,#9529,#9530,#9531,#9532,#9533,#9534,#9535,#9536,#9537,#9538,#9539,
#9540,#9541,#9542,#9543,#9544,#9545,#9546,#9547,#9548,#9549,#9550,#9551,
#9552,#9553,#9554,#9555,#9556,#9557,#9558,#9559,#9560,#9561,#9562));
#10314=AXIS2_PLACEMENT_3D('',#23206,#11656,#11657);
#10315=AXIS2_PLACEMENT_3D('',#23207,#11658,#11659);
#10316=AXIS2_PLACEMENT_3D('',#23235,#11661,#11662);
#10317=AXIS2_PLACEMENT_3D('',#23246,#11664,#11665);
#10318=AXIS2_PLACEMENT_3D('',#23269,#11666,#11667);
#10319=AXIS2_PLACEMENT_3D('',#23320,#11669,#11670);
#10320=AXIS2_PLACEMENT_3D('',#23368,#11672,#11673);
#10321=AXIS2_PLACEMENT_3D('',#23416,#11675,#11676);
#10322=AXIS2_PLACEMENT_3D('',#23467,#11678,#11679);
#10323=AXIS2_PLACEMENT_3D('',#23515,#11681,#11682);
#10324=AXIS2_PLACEMENT_3D('',#23563,#11684,#11685);
#10325=AXIS2_PLACEMENT_3D('',#23614,#11687,#11688);
#10326=AXIS2_PLACEMENT_3D('',#23665,#11690,#11691);
#10327=AXIS2_PLACEMENT_3D('',#23713,#11693,#11694);
#10328=AXIS2_PLACEMENT_3D('',#23764,#11696,#11697);
#10329=AXIS2_PLACEMENT_3D('',#23783,#11699,#11700);
#10330=AXIS2_PLACEMENT_3D('',#23803,#11701,#11702);
#10331=AXIS2_PLACEMENT_3D('',#23816,#11704,#11705);
#10332=AXIS2_PLACEMENT_3D('',#23825,#11706,#11707);
#10333=AXIS2_PLACEMENT_3D('',#23849,#11709,#11710);
#10334=AXIS2_PLACEMENT_3D('',#23874,#11712,#11713);
#10335=AXIS2_PLACEMENT_3D('',#23899,#11715,#11716);
#10336=AXIS2_PLACEMENT_3D('',#23923,#11718,#11719);
#10337=AXIS2_PLACEMENT_3D('',#23948,#11721,#11722);
#10338=AXIS2_PLACEMENT_3D('',#23972,#11724,#11725);
#10339=AXIS2_PLACEMENT_3D('',#23997,#11727,#11728);
#10340=AXIS2_PLACEMENT_3D('',#24021,#11730,#11731);
#10341=AXIS2_PLACEMENT_3D('',#24046,#11733,#11734);
#10342=AXIS2_PLACEMENT_3D('',#24071,#11736,#11737);
#10343=AXIS2_PLACEMENT_3D('',#24095,#11739,#11740);
#10344=AXIS2_PLACEMENT_3D('',#24106,#11742,#11743);
#10345=AXIS2_PLACEMENT_3D('',#24112,#11744,#11745);
#10346=AXIS2_PLACEMENT_3D('',#24122,#11747,#11748);
#10347=AXIS2_PLACEMENT_3D('',#24125,#11750,#11751);
#10348=AXIS2_PLACEMENT_3D('',#24127,#11752,#11753);
#10349=AXIS2_PLACEMENT_3D('',#24138,#11754,#11755);
#10350=AXIS2_PLACEMENT_3D('',#24189,#11757,#11758);
#10351=AXIS2_PLACEMENT_3D('',#24240,#11760,#11761);
#10352=AXIS2_PLACEMENT_3D('',#24288,#11763,#11764);
#10353=AXIS2_PLACEMENT_3D('',#24339,#11766,#11767);
#10354=AXIS2_PLACEMENT_3D('',#24390,#11769,#11770);
#10355=AXIS2_PLACEMENT_3D('',#24438,#11772,#11773);
#10356=AXIS2_PLACEMENT_3D('',#24489,#11775,#11776);
#10357=AXIS2_PLACEMENT_3D('',#24540,#11778,#11779);
#10358=AXIS2_PLACEMENT_3D('',#24588,#11781,#11782);
#10359=AXIS2_PLACEMENT_3D('',#24639,#11784,#11785);
#10360=AXIS2_PLACEMENT_3D('',#24690,#11787,#11788);
#10361=AXIS2_PLACEMENT_3D('',#24738,#11790,#11791);
#10362=AXIS2_PLACEMENT_3D('',#24789,#11793,#11794);
#10363=AXIS2_PLACEMENT_3D('',#24840,#11796,#11797);
#10364=AXIS2_PLACEMENT_3D('',#24888,#11799,#11800);
#10365=AXIS2_PLACEMENT_3D('',#24939,#11802,#11803);
#10366=AXIS2_PLACEMENT_3D('',#24958,#11805,#11806);
#10367=AXIS2_PLACEMENT_3D('',#24978,#11807,#11808);
#10368=AXIS2_PLACEMENT_3D('',#24992,#11810,#11811);
#10369=AXIS2_PLACEMENT_3D('',#25002,#11812,#11813);
#10370=AXIS2_PLACEMENT_3D('',#25026,#11815,#11816);
#10371=AXIS2_PLACEMENT_3D('',#25051,#11818,#11819);
#10372=AXIS2_PLACEMENT_3D('',#25076,#11821,#11822);
#10373=AXIS2_PLACEMENT_3D('',#25100,#11824,#11825);
#10374=AXIS2_PLACEMENT_3D('',#25125,#11827,#11828);
#10375=AXIS2_PLACEMENT_3D('',#25150,#11830,#11831);
#10376=AXIS2_PLACEMENT_3D('',#25174,#11833,#11834);
#10377=AXIS2_PLACEMENT_3D('',#25199,#11836,#11837);
#10378=AXIS2_PLACEMENT_3D('',#25224,#11839,#11840);
#10379=AXIS2_PLACEMENT_3D('',#25248,#11842,#11843);
#10380=AXIS2_PLACEMENT_3D('',#25273,#11845,#11846);
#10381=AXIS2_PLACEMENT_3D('',#25298,#11848,#11849);
#10382=AXIS2_PLACEMENT_3D('',#25322,#11851,#11852);
#10383=AXIS2_PLACEMENT_3D('',#25347,#11854,#11855);
#10384=AXIS2_PLACEMENT_3D('',#25372,#11857,#11858);
#10385=AXIS2_PLACEMENT_3D('',#25396,#11860,#11861);
#10386=AXIS2_PLACEMENT_3D('',#25407,#11863,#11864);
#10387=AXIS2_PLACEMENT_3D('',#25413,#11865,#11866);
#10388=AXIS2_PLACEMENT_3D('',#25521,#11867,#11868);
#10389=AXIS2_PLACEMENT_3D('',#26640,#11869,#11870);
#10390=AXIS2_PLACEMENT_3D('',#26641,#11871,#11872);
#10391=AXIS2_PLACEMENT_3D('',#26642,#11873,#11874);
#10392=AXIS2_PLACEMENT_3D('',#26753,#11875,#11876);
#10393=AXIS2_PLACEMENT_3D('',#27614,#11877,#11878);
#10394=AXIS2_PLACEMENT_3D('',#27615,#11879,#11880);
#10395=AXIS2_PLACEMENT_3D('',#27616,#11881,#11882);
#10396=AXIS2_PLACEMENT_3D('',#27625,#11887,#11888);
#10397=AXIS2_PLACEMENT_3D('',#27631,#11892,#11893);
#10398=AXIS2_PLACEMENT_3D('',#27637,#11897,#11898);
#10399=AXIS2_PLACEMENT_3D('',#27640,#11901,#11902);
#10400=AXIS2_PLACEMENT_3D('',#27641,#11903,#11904);
#11656=DIRECTION('axis',(0.,0.,1.));
#11657=DIRECTION('refdir',(1.,0.,0.));
#11658=DIRECTION('center_axis',(0.,0.,1.));
#11659=DIRECTION('ref_axis',(-1.,0.,0.));
#11660=DIRECTION('',(0.,0.,1.));
#11661=DIRECTION('center_axis',(0.,0.,-1.));
#11662=DIRECTION('ref_axis',(-1.,0.,0.));
#11663=DIRECTION('',(0.,0.,1.));
#11664=DIRECTION('center_axis',(0.,0.,-1.));
#11665=DIRECTION('ref_axis',(-1.,0.,0.));
#11666=DIRECTION('center_axis',(0.,0.,1.));
#11667=DIRECTION('ref_axis',(-1.,0.,0.));
#11668=DIRECTION('',(0.,0.,1.));
#11669=DIRECTION('center_axis',(0.,0.,1.));
#11670=DIRECTION('ref_axis',(-1.,0.,0.));
#11671=DIRECTION('',(0.,0.,1.));
#11672=DIRECTION('center_axis',(0.,0.,1.));
#11673=DIRECTION('ref_axis',(-1.,0.,0.));
#11674=DIRECTION('',(0.,0.,1.));
#11675=DIRECTION('center_axis',(0.,0.,1.));
#11676=DIRECTION('ref_axis',(-1.,0.,0.));
#11677=DIRECTION('',(0.,0.,1.));
#11678=DIRECTION('center_axis',(0.,0.,1.));
#11679=DIRECTION('ref_axis',(-1.,0.,0.));
#11680=DIRECTION('',(0.,0.,1.));
#11681=DIRECTION('center_axis',(0.,0.,1.));
#11682=DIRECTION('ref_axis',(-1.,0.,0.));
#11683=DIRECTION('',(0.,0.,1.));
#11684=DIRECTION('center_axis',(0.,0.,1.));
#11685=DIRECTION('ref_axis',(-1.,0.,0.));
#11686=DIRECTION('',(0.,0.,1.));
#11687=DIRECTION('center_axis',(0.,0.,1.));
#11688=DIRECTION('ref_axis',(-1.,0.,0.));
#11689=DIRECTION('',(0.,0.,1.));
#11690=DIRECTION('center_axis',(0.,0.,1.));
#11691=DIRECTION('ref_axis',(-1.,0.,0.));
#11692=DIRECTION('',(0.,0.,1.));
#11693=DIRECTION('center_axis',(0.,0.,1.));
#11694=DIRECTION('ref_axis',(-1.,0.,0.));
#11695=DIRECTION('',(0.,0.,1.));
#11696=DIRECTION('center_axis',(0.,0.,1.));
#11697=DIRECTION('ref_axis',(-0.938434237953747,-0.345457929473576,0.));
#11698=DIRECTION('',(0.,0.,1.));
#11699=DIRECTION('center_axis',(0.,0.,-1.));
#11700=DIRECTION('ref_axis',(-1.,0.,0.));
#11701=DIRECTION('center_axis',(0.,0.,1.));
#11702=DIRECTION('ref_axis',(-0.450135889590755,0.892960066801612,0.));
#11703=DIRECTION('',(-1.22464679914735E-16,-7.02543712147503E-30,1.));
#11704=DIRECTION('center_axis',(0.,0.,-1.));
#11705=DIRECTION('ref_axis',(-1.,-5.72445829159016E-14,0.));
#11706=DIRECTION('center_axis',(0.,0.,1.));
#11707=DIRECTION('ref_axis',(-1.,-5.72445829159016E-14,0.));
#11708=DIRECTION('',(-1.22464679914735E-16,-7.02543712147503E-30,1.));
#11709=DIRECTION('center_axis',(0.,0.,1.));
#11710=DIRECTION('ref_axis',(-1.,-5.72445829159016E-14,0.));
#11711=DIRECTION('',(-1.22464679914735E-16,-7.02543712147503E-30,1.));
#11712=DIRECTION('center_axis',(0.,0.,1.));
#11713=DIRECTION('ref_axis',(-1.,-5.72445829159016E-14,0.));
#11714=DIRECTION('',(-1.22464679914735E-16,-7.02543712147503E-30,1.));
#11715=DIRECTION('center_axis',(0.,0.,1.));
#11716=DIRECTION('ref_axis',(-1.,-5.72445829159016E-14,0.));
#11717=DIRECTION('',(-1.22464679914735E-16,-7.02543712147503E-30,1.));
#11718=DIRECTION('center_axis',(0.,0.,1.));
#11719=DIRECTION('ref_axis',(-1.,-5.72445829159016E-14,0.));
#11720=DIRECTION('',(-1.22464679914735E-16,-7.02543712147503E-30,1.));
#11721=DIRECTION('center_axis',(0.,0.,1.));
#11722=DIRECTION('ref_axis',(-1.,-5.72445829159016E-14,0.));
#11723=DIRECTION('',(-1.22464679914735E-16,-7.02543712147503E-30,1.));
#11724=DIRECTION('center_axis',(0.,0.,1.));
#11725=DIRECTION('ref_axis',(-1.,-5.72445829159016E-14,0.));
#11726=DIRECTION('',(-1.22464679914735E-16,-7.02543712147503E-30,1.));
#11727=DIRECTION('center_axis',(0.,0.,1.));
#11728=DIRECTION('ref_axis',(-1.,-5.72445829159016E-14,0.));
#11729=DIRECTION('',(-1.22464679914735E-16,-7.02543712147503E-30,1.));
#11730=DIRECTION('center_axis',(0.,0.,1.));
#11731=DIRECTION('ref_axis',(-1.,-5.72445829159016E-14,0.));
#11732=DIRECTION('',(-1.22464679914735E-16,-7.02543712147503E-30,1.));
#11733=DIRECTION('center_axis',(0.,0.,1.));
#11734=DIRECTION('ref_axis',(-1.,-5.72445829159016E-14,0.));
#11735=DIRECTION('',(-1.22464679914735E-16,-7.02543712147503E-30,1.));
#11736=DIRECTION('center_axis',(0.,0.,1.));
#11737=DIRECTION('ref_axis',(-1.,-5.72445829159016E-14,0.));
#11738=DIRECTION('',(-1.22464679914735E-16,-7.02543712147503E-30,1.));
#11739=DIRECTION('center_axis',(0.,0.,1.));
#11740=DIRECTION('ref_axis',(0.609351642559645,-0.79290010449606,0.));
#11741=DIRECTION('',(-1.22464679914735E-16,-7.02543712147503E-30,1.));
#11742=DIRECTION('center_axis',(0.,0.,1.));
#11743=DIRECTION('ref_axis',(-1.,-5.72445829159016E-14,0.));
#11744=DIRECTION('center_axis',(0.,0.,-1.));
#11745=DIRECTION('ref_axis',(1.,0.,0.));
#11746=DIRECTION('',(0.,0.,-1.));
#11747=DIRECTION('center_axis',(0.,0.,1.));
#11748=DIRECTION('ref_axis',(1.,0.,0.));
#11749=DIRECTION('',(0.,0.,-1.));
#11750=DIRECTION('center_axis',(0.,0.,1.));
#11751=DIRECTION('ref_axis',(1.,0.,0.));
#11752=DIRECTION('center_axis',(0.,0.,1.));
#11753=DIRECTION('ref_axis',(1.,0.,0.));
#11754=DIRECTION('center_axis',(0.,0.,-1.));
#11755=DIRECTION('ref_axis',(1.,0.,0.));
#11756=DIRECTION('',(0.,0.,-1.));
#11757=DIRECTION('center_axis',(0.,0.,-1.));
#11758=DIRECTION('ref_axis',(1.,0.,0.));
#11759=DIRECTION('',(0.,0.,-1.));
#11760=DIRECTION('center_axis',(0.,0.,-1.));
#11761=DIRECTION('ref_axis',(1.,0.,0.));
#11762=DIRECTION('',(0.,0.,-1.));
#11763=DIRECTION('center_axis',(0.,0.,-1.));
#11764=DIRECTION('ref_axis',(1.,0.,0.));
#11765=DIRECTION('',(0.,0.,-1.));
#11766=DIRECTION('center_axis',(0.,0.,-1.));
#11767=DIRECTION('ref_axis',(1.,0.,0.));
#11768=DIRECTION('',(0.,0.,-1.));
#11769=DIRECTION('center_axis',(0.,0.,-1.));
#11770=DIRECTION('ref_axis',(1.,0.,0.));
#11771=DIRECTION('',(0.,0.,-1.));
#11772=DIRECTION('center_axis',(0.,0.,-1.));
#11773=DIRECTION('ref_axis',(1.,0.,0.));
#11774=DIRECTION('',(0.,0.,-1.));
#11775=DIRECTION('center_axis',(0.,0.,-1.));
#11776=DIRECTION('ref_axis',(1.,0.,0.));
#11777=DIRECTION('',(0.,0.,-1.));
#11778=DIRECTION('center_axis',(0.,0.,-1.));
#11779=DIRECTION('ref_axis',(1.,0.,0.));
#11780=DIRECTION('',(0.,0.,-1.));
#11781=DIRECTION('center_axis',(0.,0.,-1.));
#11782=DIRECTION('ref_axis',(1.,0.,0.));
#11783=DIRECTION('',(0.,0.,-1.));
#11784=DIRECTION('center_axis',(0.,0.,-1.));
#11785=DIRECTION('ref_axis',(1.,0.,0.));
#11786=DIRECTION('',(0.,0.,-1.));
#11787=DIRECTION('center_axis',(0.,0.,-1.));
#11788=DIRECTION('ref_axis',(1.,0.,0.));
#11789=DIRECTION('',(0.,0.,-1.));
#11790=DIRECTION('center_axis',(0.,0.,-1.));
#11791=DIRECTION('ref_axis',(1.,0.,0.));
#11792=DIRECTION('',(0.,0.,-1.));
#11793=DIRECTION('center_axis',(0.,0.,-1.));
#11794=DIRECTION('ref_axis',(1.,0.,0.));
#11795=DIRECTION('',(0.,0.,-1.));
#11796=DIRECTION('center_axis',(0.,0.,-1.));
#11797=DIRECTION('ref_axis',(1.,0.,0.));
#11798=DIRECTION('',(0.,0.,-1.));
#11799=DIRECTION('center_axis',(0.,0.,-1.));
#11800=DIRECTION('ref_axis',(1.,0.,0.));
#11801=DIRECTION('',(0.,0.,-1.));
#11802=DIRECTION('center_axis',(0.,0.,-1.));
#11803=DIRECTION('ref_axis',(0.937376106323228,-0.348318870138132,0.));
#11804=DIRECTION('',(0.,0.,-1.));
#11805=DIRECTION('center_axis',(0.,0.,-1.));
#11806=DIRECTION('ref_axis',(1.,0.,0.));
#11807=DIRECTION('center_axis',(0.,0.,-1.));
#11808=DIRECTION('ref_axis',(1.,-9.27379496885572E-14,0.));
#11809=DIRECTION('',(1.22464679914735E-16,-1.13721209223846E-29,-1.));
#11810=DIRECTION('center_axis',(0.,0.,1.));
#11811=DIRECTION('ref_axis',(1.,-9.27379496885572E-14,0.));
#11812=DIRECTION('center_axis',(0.,0.,-1.));
#11813=DIRECTION('ref_axis',(1.,-9.27379496885572E-14,0.));
#11814=DIRECTION('',(1.22464679914735E-16,-1.13721209223846E-29,-1.));
#11815=DIRECTION('center_axis',(0.,0.,-1.));
#11816=DIRECTION('ref_axis',(1.,-9.27379496885572E-14,0.));
#11817=DIRECTION('',(1.22464679914735E-16,-1.13721209223846E-29,-1.));
#11818=DIRECTION('center_axis',(0.,0.,-1.));
#11819=DIRECTION('ref_axis',(1.,-9.27379496885572E-14,0.));
#11820=DIRECTION('',(1.22464679914735E-16,-1.13721209223846E-29,-1.));
#11821=DIRECTION('center_axis',(0.,0.,-1.));
#11822=DIRECTION('ref_axis',(1.,-9.27379496885572E-14,0.));
#11823=DIRECTION('',(1.22464679914735E-16,-1.13721209223846E-29,-1.));
#11824=DIRECTION('center_axis',(0.,0.,-1.));
#11825=DIRECTION('ref_axis',(1.,-9.27379496885572E-14,0.));
#11826=DIRECTION('',(1.22464679914735E-16,-1.13721209223846E-29,-1.));
#11827=DIRECTION('center_axis',(0.,0.,-1.));
#11828=DIRECTION('ref_axis',(1.,-9.27379496885572E-14,0.));
#11829=DIRECTION('',(1.22464679914735E-16,-1.13721209223846E-29,-1.));
#11830=DIRECTION('center_axis',(0.,0.,-1.));
#11831=DIRECTION('ref_axis',(1.,-9.27379496885572E-14,0.));
#11832=DIRECTION('',(1.22464679914735E-16,-1.13721209223846E-29,-1.));
#11833=DIRECTION('center_axis',(0.,0.,-1.));
#11834=DIRECTION('ref_axis',(1.,-9.27379496885572E-14,0.));
#11835=DIRECTION('',(1.22464679914735E-16,-1.13721209223846E-29,-1.));
#11836=DIRECTION('center_axis',(0.,0.,-1.));
#11837=DIRECTION('ref_axis',(1.,-9.27379496885572E-14,0.));
#11838=DIRECTION('',(1.22464679914735E-16,-1.13721209223846E-29,-1.));
#11839=DIRECTION('center_axis',(0.,0.,-1.));
#11840=DIRECTION('ref_axis',(1.,-9.27379496885572E-14,0.));
#11841=DIRECTION('',(1.22464679914735E-16,-1.13721209223846E-29,-1.));
#11842=DIRECTION('center_axis',(0.,0.,-1.));
#11843=DIRECTION('ref_axis',(1.,-9.27379496885572E-14,0.));
#11844=DIRECTION('',(1.22464679914735E-16,-1.13721209223846E-29,-1.));
#11845=DIRECTION('center_axis',(0.,0.,-1.));
#11846=DIRECTION('ref_axis',(1.,-9.27379496885572E-14,0.));
#11847=DIRECTION('',(1.22464679914735E-16,-1.13721209223846E-29,-1.));
#11848=DIRECTION('center_axis',(0.,0.,-1.));
#11849=DIRECTION('ref_axis',(1.,-9.27379496885572E-14,0.));
#11850=DIRECTION('',(1.22464679914735E-16,-1.13721209223846E-29,-1.));
#11851=DIRECTION('center_axis',(0.,0.,-1.));
#11852=DIRECTION('ref_axis',(1.,-9.27379496885572E-14,0.));
#11853=DIRECTION('',(1.22464679914735E-16,-1.13721209223846E-29,-1.));
#11854=DIRECTION('center_axis',(0.,0.,-1.));
#11855=DIRECTION('ref_axis',(1.,-9.27379496885572E-14,0.));
#11856=DIRECTION('',(1.22464679914735E-16,-1.13721209223846E-29,-1.));
#11857=DIRECTION('center_axis',(0.,0.,-1.));
#11858=DIRECTION('ref_axis',(1.,-9.27379496885572E-14,0.));
#11859=DIRECTION('',(1.22464679914735E-16,-1.13721209223846E-29,-1.));
#11860=DIRECTION('center_axis',(0.,0.,-1.));
#11861=DIRECTION('ref_axis',(-0.609161390867883,-0.793046278520936,0.));
#11862=DIRECTION('',(1.22464679914735E-16,-1.13721209223846E-29,-1.));
#11863=DIRECTION('center_axis',(0.,0.,-1.));
#11864=DIRECTION('ref_axis',(1.,-9.27379496885572E-14,0.));
#11865=DIRECTION('center_axis',(0.,0.,1.));
#11866=DIRECTION('ref_axis',(1.,0.,0.));
#11867=DIRECTION('center_axis',(0.,0.,-1.));
#11868=DIRECTION('ref_axis',(1.,-9.27379496885572E-14,0.));
#11869=DIRECTION('center_axis',(0.,0.,-1.));
#11870=DIRECTION('ref_axis',(1.,0.,0.));
#11871=DIRECTION('center_axis',(0.,0.,-1.));
#11872=DIRECTION('ref_axis',(1.,0.,0.));
#11873=DIRECTION('center_axis',(0.,0.,1.));
#11874=DIRECTION('ref_axis',(1.,0.,0.));
#11875=DIRECTION('center_axis',(0.,0.,1.));
#11876=DIRECTION('ref_axis',(-1.,-5.72445829159016E-14,0.));
#11877=DIRECTION('center_axis',(0.,0.,1.));
#11878=DIRECTION('ref_axis',(-1.,0.,0.));
#11879=DIRECTION('center_axis',(0.,0.,1.));
#11880=DIRECTION('ref_axis',(-1.,0.,0.));
#11881=DIRECTION('center_axis',(0.,1.,0.));
#11882=DIRECTION('ref_axis',(-1.,0.,0.));
#11883=DIRECTION('',(-1.,0.,0.));
#11884=DIRECTION('',(0.,0.,1.));
#11885=DIRECTION('',(-1.,0.,0.));
#11886=DIRECTION('',(0.,0.,1.));
#11887=DIRECTION('center_axis',(1.,0.,0.));
#11888=DIRECTION('ref_axis',(0.,1.,0.));
#11889=DIRECTION('',(0.,1.,0.));
#11890=DIRECTION('',(0.,1.,0.));
#11891=DIRECTION('',(0.,0.,1.));
#11892=DIRECTION('center_axis',(0.,-1.,0.));
#11893=DIRECTION('ref_axis',(1.,0.,0.));
#11894=DIRECTION('',(1.,0.,0.));
#11895=DIRECTION('',(1.,0.,0.));
#11896=DIRECTION('',(0.,0.,1.));
#11897=DIRECTION('center_axis',(-1.,0.,0.));
#11898=DIRECTION('ref_axis',(0.,-1.,0.));
#11899=DIRECTION('',(0.,-1.,0.));
#11900=DIRECTION('',(0.,-1.,0.));
#11901=DIRECTION('center_axis',(0.,0.,1.));
#11902=DIRECTION('ref_axis',(1.,0.,0.));
#11903=DIRECTION('center_axis',(0.,0.,1.));
#11904=DIRECTION('ref_axis',(1.,0.,0.));
#23206=CARTESIAN_POINT('',(0.,0.,0.));
#23207=CARTESIAN_POINT('Origin',(0.,0.,1.3));
#23208=CARTESIAN_POINT('',(0.166752921449725,-0.000121400228749406,1.61285196366098));
#23209=CARTESIAN_POINT('',(0.166796959880497,9.66735530056473E-5,1.63214803633902));
#23210=CARTESIAN_POINT('',(0.1666,2.04026156737949E-17,1.3));
#23211=CARTESIAN_POINT('',(0.163512932725146,-0.0319230454628286,1.7));
#23212=CARTESIAN_POINT('Ctrl Pts',(0.166796959880497,9.66735530056473E-5,
1.63214803633902));
#23213=CARTESIAN_POINT('Ctrl Pts',(0.166837734552074,0.00590520031683778,
1.63253777944574));
#23214=CARTESIAN_POINT('Ctrl Pts',(0.166560755157907,0.0117098399368759,
1.63292752255246));
#23215=CARTESIAN_POINT('Ctrl Pts',(0.165953190799148,0.0174796970799782,
1.63331726565918));
#23216=CARTESIAN_POINT('Ctrl Pts',(0.160178154195734,0.0723234938194388,
1.63702186201144));
#23217=CARTESIAN_POINT('Ctrl Pts',(0.124534989745148,0.12402471730472,1.64072645836371));
#23218=CARTESIAN_POINT('Ctrl Pts',(0.0753220427557469,0.148912116862319,
1.64443105471598));
#23219=CARTESIAN_POINT('Ctrl Pts',(0.0261090957663466,0.173799516419917,
1.64813565106825));
#23220=CARTESIAN_POINT('Ctrl Pts',(-0.0366736337618685,0.171873092049834,
1.65184024742052));
#23221=CARTESIAN_POINT('Ctrl Pts',(-0.0842665124811252,0.144033445936741,
1.65554484377278));
#23222=CARTESIAN_POINT('Ctrl Pts',(-0.131859391200383,0.116193799823647,
1.65924944012505));
#23223=CARTESIAN_POINT('Ctrl Pts',(-0.164262419110682,0.0624409319675427,
1.66295403647732));
#23224=CARTESIAN_POINT('Ctrl Pts',(-0.16669782361829,0.00733866012848643,
1.66665863282959));
#23225=CARTESIAN_POINT('Ctrl Pts',(-0.169133228125899,-0.0477636117105698,
1.67036322918185));
#23226=CARTESIAN_POINT('Ctrl Pts',(-0.141601009230818,-0.104215287532578,
1.67406782553412));
#23227=CARTESIAN_POINT('Ctrl Pts',(-0.0965988342506402,-0.136109501609562,
1.67777242188639));
#23228=CARTESIAN_POINT('Ctrl Pts',(-0.0515966592704642,-0.168003715686544,
1.68147701823866));
#23229=CARTESIAN_POINT('Ctrl Pts',(0.0108754717948065,-0.175340468018505,
1.68518161459093));
#23230=CARTESIAN_POINT('Ctrl Pts',(0.0619990767693629,-0.154913285529167,
1.6888862109432));
#23231=CARTESIAN_POINT('Ctrl Pts',(0.11312268174392,-0.134486103039829,
1.69259080729546));
#23232=CARTESIAN_POINT('Ctrl Pts',(0.152897760627763,-0.0862949857291919,
1.69629540364773));
#23233=CARTESIAN_POINT('Ctrl Pts',(0.163512932725146,-0.0319230454628286,
1.7));
#23234=CARTESIAN_POINT('',(0.0052623718904234,0.166820541544646,1.7));
#23235=CARTESIAN_POINT('Origin',(0.,0.,1.7));
#23236=CARTESIAN_POINT('',(0.166340825374871,-6.57396331519428E-5,1.68285196366098));
#23237=CARTESIAN_POINT('Ctrl Pts',(0.00526237188778958,0.16682061735739,
1.7));
#23238=CARTESIAN_POINT('Ctrl Pts',(0.059315846276127,0.165049198896683,
1.69636770818144));
#23239=CARTESIAN_POINT('Ctrl Pts',(0.112514618214038,0.134574177622605,
1.69273541636289));
#23240=CARTESIAN_POINT('Ctrl Pts',(0.141280425894631,0.0887797885328044,
1.68910312454433));
#23241=CARTESIAN_POINT('Ctrl Pts',(0.157782375695069,0.0625091300380853,
1.68701940424988));
#23242=CARTESIAN_POINT('Ctrl Pts',(0.166243631438541,0.0311969895334432,
1.68493568395543));
#23243=CARTESIAN_POINT('Ctrl Pts',(0.166340825374871,-6.57396331519428E-5,
1.68285196366098));
#23244=CARTESIAN_POINT('',(0.1666,-2.04026156737949E-17,1.8));
#23245=CARTESIAN_POINT('',(0.1666,2.04026156737949E-17,1.3));
#23246=CARTESIAN_POINT('Origin',(0.,0.,1.8));
#23247=CARTESIAN_POINT('Ctrl Pts',(0.166340825374871,-6.57396331519428E-5,
1.68285196366098));
#23248=CARTESIAN_POINT('Ctrl Pts',(0.166416430207622,-0.024384267097259,
1.68123108760316));
#23249=CARTESIAN_POINT('Ctrl Pts',(0.161431015607884,-0.0486728962000426,
1.67961021154535));
#23250=CARTESIAN_POINT('Ctrl Pts',(0.151232376946182,-0.070535415398117,
1.67798933548753));
#23251=CARTESIAN_POINT('Ctrl Pts',(0.12792285898394,-0.120503337672002,
1.67428473913526));
#23252=CARTESIAN_POINT('Ctrl Pts',(0.0773807749454364,-0.157797874435697,
1.67058014278299));
#23253=CARTESIAN_POINT('Ctrl Pts',(0.0227482513872868,-0.165320125260105,
1.66687554643073));
#23254=CARTESIAN_POINT('Ctrl Pts',(-0.0318842721708627,-0.172842376084512,
1.66317095007846));
#23255=CARTESIAN_POINT('Ctrl Pts',(-0.0906072352486578,-0.150592340969633,
1.65946635372619));
#23256=CARTESIAN_POINT('Ctrl Pts',(-0.126551605667113,-0.108768963100728,
1.65576175737392));
#23257=CARTESIAN_POINT('Ctrl Pts',(-0.162495976085569,-0.0669455852318239,
1.65205716102165));
#23258=CARTESIAN_POINT('Ctrl Pts',(-0.175661753844685,-0.00554886460889432,
1.64835256466938));
#23259=CARTESIAN_POINT('Ctrl Pts',(-0.160020484350268,0.0473310422055452,
1.64464796831712));
#23260=CARTESIAN_POINT('Ctrl Pts',(-0.144379214855851,0.100210949019985,
1.64094337196485));
#23261=CARTESIAN_POINT('Ctrl Pts',(-0.0999308981078997,0.144574042025934,
1.63723877561258));
#23262=CARTESIAN_POINT('Ctrl Pts',(-0.0470191573240233,0.160112912591645,
1.63353417926031));
#23263=CARTESIAN_POINT('Ctrl Pts',(0.00589258345985309,0.175651783157355,
1.62982958290805));
#23264=CARTESIAN_POINT('Ctrl Pts',(0.067267748279655,0.162366431282826,
1.62612498655578));
#23265=CARTESIAN_POINT('Ctrl Pts',(0.109018480103692,0.126339265236092,
1.62242039020351));
#23266=CARTESIAN_POINT('Ctrl Pts',(0.144963809686008,0.0953216446845623,
1.61923091468933));
#23267=CARTESIAN_POINT('Ctrl Pts',(0.166362794628908,0.0474469630018487,
1.61604143917516));
#23268=CARTESIAN_POINT('Ctrl Pts',(0.166752921449725,-0.000121400228749406,
1.61285196366098));
#23269=CARTESIAN_POINT('Origin',(0.,0.,1.3));
#23270=CARTESIAN_POINT('',(0.166721717270512,0.00013247748987999,1.54285196366098));
#23271=CARTESIAN_POINT('',(0.166368100504911,8.32215516180224E-5,1.56214803633902));
#23272=CARTESIAN_POINT('',(0.1666,2.04026156737949E-17,1.3));
#23273=CARTESIAN_POINT('Ctrl Pts',(0.166368100504911,8.32215516180223E-5,
1.56214803633902));
#23274=CARTESIAN_POINT('Ctrl Pts',(0.166469575983711,0.0225191704554514,
1.56364353466546));
#23275=CARTESIAN_POINT('Ctrl Pts',(0.162248711501603,0.0449185271683059,
1.56513903299191));
#23276=CARTESIAN_POINT('Ctrl Pts',(0.153524147106197,0.0653993692500711,
1.56663453131835));
#23277=CARTESIAN_POINT('Ctrl Pts',(0.131911960142923,0.116133797718439,
1.57033912767062));
#23278=CARTESIAN_POINT('Ctrl Pts',(0.0826635066749161,0.155095554237362,
1.57404372402289));
#23279=CARTESIAN_POINT('Ctrl Pts',(0.028317337914343,0.164453369456362,
1.57774832037515));
#23280=CARTESIAN_POINT('Ctrl Pts',(-0.026028830846231,0.173811184675361,
1.58145291672742));
#23281=CARTESIAN_POINT('Ctrl Pts',(-0.0854727148993724,0.153565058594437,
1.58515751307969));
#23282=CARTESIAN_POINT('Ctrl Pts',(-0.122808942133701,0.11298112966685,
1.58886210943196));
#23283=CARTESIAN_POINT('Ctrl Pts',(-0.160145169368031,0.0723972007392629,
1.59256670578423));
#23284=CARTESIAN_POINT('Ctrl Pts',(-0.175373739783547,0.0114754689650147,
1.59627130213649));
#23285=CARTESIAN_POINT('Ctrl Pts',(-0.161526248741115,-0.041903625100424,
1.59997589848876));
#23286=CARTESIAN_POINT('Ctrl Pts',(-0.147678757698683,-0.0952827191658612,
1.60368049484103));
#23287=CARTESIAN_POINT('Ctrl Pts',(-0.1047552051983,-0.14111917552249,1.6073850911933));
#23288=CARTESIAN_POINT('Ctrl Pts',(-0.0523978126792817,-0.158434271662077,
1.61108968754557));
#23289=CARTESIAN_POINT('Ctrl Pts',(-4.04201602626775E-5,-0.175749367801665,
1.61479428389783));
#23290=CARTESIAN_POINT('Ctrl Pts',(0.0617508123773913,-0.164543103724215,
1.6184988802501));
#23291=CARTESIAN_POINT('Ctrl Pts',(0.104692974268098,-0.12994678668867,
1.62220347660237));
#23292=CARTESIAN_POINT('Ctrl Pts',(0.143117393875163,-0.0989901849689851,
1.62551832984792));
#23293=CARTESIAN_POINT('Ctrl Pts',(0.166450162079376,-0.0493061599110598,
1.62883318309347));
#23294=CARTESIAN_POINT('Ctrl Pts',(0.166796959880497,9.66735530056473E-5,
1.63214803633902));
#23295=CARTESIAN_POINT('Ctrl Pts',(0.166752921449725,-0.000121400228749406,
1.61285196366098));
#23296=CARTESIAN_POINT('Ctrl Pts',(0.166815929443988,-0.00780399726549495,
1.61233684282289));
#23297=CARTESIAN_POINT('Ctrl Pts',(0.166330935441723,-0.0154786041905287,
1.6118217219848));
#23298=CARTESIAN_POINT('Ctrl Pts',(0.165270714247807,-0.0230729153352646,
1.61130660114671));
#23299=CARTESIAN_POINT('Ctrl Pts',(0.157645917739612,-0.0776889496409508,
1.60760200479444));
#23300=CARTESIAN_POINT('Ctrl Pts',(0.120270025894947,-0.128152038033383,
1.60389740844217));
#23301=CARTESIAN_POINT('Ctrl Pts',(0.0702485553938763,-0.151366836780329,
1.6001928120899));
#23302=CARTESIAN_POINT('Ctrl Pts',(0.0202270848928061,-0.174581635527273,
1.59648821573763));
#23303=CARTESIAN_POINT('Ctrl Pts',(-0.0424399642646696,-0.170548144628732,
1.59278361938537));
#23304=CARTESIAN_POINT('Ctrl Pts',(-0.0890727806898626,-0.141112640607554,
1.5890790230331));
#23305=CARTESIAN_POINT('Ctrl Pts',(-0.135705597115056,-0.111677136586376,
1.58537442668083));
#23306=CARTESIAN_POINT('Ctrl Pts',(-0.166304180807966,-0.0568396194425618,
1.58166983032856));
#23307=CARTESIAN_POINT('Ctrl Pts',(-0.16686485427816,-0.00169661928996206,
1.57796523397629));
#23308=CARTESIAN_POINT('Ctrl Pts',(-0.167425527748354,0.0534463808626376,
1.57426063762402));
#23309=CARTESIAN_POINT('Ctrl Pts',(-0.137948290995833,0.108894864024023,
1.57055604127176));
#23310=CARTESIAN_POINT('Ctrl Pts',(-0.0919236010333964,0.139272428377062,
1.56685144491949));
#23311=CARTESIAN_POINT('Ctrl Pts',(-0.0458989110709602,0.169649992730101,
1.56314684856722));
#23312=CARTESIAN_POINT('Ctrl Pts',(0.0166732321013904,0.174956638274794,
1.55944225221495));
#23313=CARTESIAN_POINT('Ctrl Pts',(0.0671563493099001,0.152763795116617,
1.55573765586268));
#23314=CARTESIAN_POINT('Ctrl Pts',(0.117639466518409,0.13057095195844,1.55203305951042));
#23315=CARTESIAN_POINT('Ctrl Pts',(0.156033557763077,0.0808786200973942,
1.54832846315815));
#23316=CARTESIAN_POINT('Ctrl Pts',(0.164767340619488,0.0264287526812992,
1.54462386680588));
#23317=CARTESIAN_POINT('Ctrl Pts',(0.166159792575437,0.0177476547388351,
1.54403323242425));
#23318=CARTESIAN_POINT('Ctrl Pts',(0.166798314017023,0.0089456257803759,
1.54344259804261));
#23319=CARTESIAN_POINT('Ctrl Pts',(0.166721717270512,0.00013247748987999,
1.54285196366098));
#23320=CARTESIAN_POINT('Origin',(0.,0.,1.3));
#23321=CARTESIAN_POINT('',(0.166334949033457,3.80241454671915E-5,1.47285196366098));
#23322=CARTESIAN_POINT('',(0.166495616539739,-0.000143126867227327,1.49214803633902));
#23323=CARTESIAN_POINT('',(0.1666,2.04026156737949E-17,1.3));
#23324=CARTESIAN_POINT('Ctrl Pts',(0.166495616539739,-0.000143126867227327,
1.49214803633902));
#23325=CARTESIAN_POINT('Ctrl Pts',(0.166176505544999,0.0388065957770001,
1.49474928988519));
#23326=CARTESIAN_POINT('Ctrl Pts',(0.15254095518154,0.0779576027494656,
1.49735054343136));
#23327=CARTESIAN_POINT('Ctrl Pts',(0.127581990737563,0.107562045989894,
1.49995179697752));
#23328=CARTESIAN_POINT('Ctrl Pts',(0.0920364789316288,0.149723454131357,
1.50365639332979));
#23329=CARTESIAN_POINT('Ctrl Pts',(0.0335245204022979,0.172522270232617,
1.50736098968206));
#23330=CARTESIAN_POINT('Ctrl Pts',(-0.0211755609783529,0.165524482759979,
1.51106558603433));
#23331=CARTESIAN_POINT('Ctrl Pts',(-0.0758756423590036,0.158526695287341,
1.5147701823866));
#23332=CARTESIAN_POINT('Ctrl Pts',(-0.126763846590974,0.121732304240806,
1.51847477873887));
#23333=CARTESIAN_POINT('Ctrl Pts',(-0.150550887470885,0.0719804791091254,
1.52217937509113));
#23334=CARTESIAN_POINT('Ctrl Pts',(-0.174337928350795,0.0222286539774451,
1.5258839714434));
#23335=CARTESIAN_POINT('Ctrl Pts',(-0.171023805878645,-0.0404806052393804,
1.52958856779567));
#23336=CARTESIAN_POINT('Ctrl Pts',(-0.142125268024159,-0.0874480653886775,
1.53329316414794));
#23337=CARTESIAN_POINT('Ctrl Pts',(-0.113226730169674,-0.134415525537975,
1.5369977605002));
#23338=CARTESIAN_POINT('Ctrl Pts',(-0.058743776932853,-0.165641186619743,
1.54070235685247));
#23339=CARTESIAN_POINT('Ctrl Pts',(-0.00361080053401195,-0.166834419219364,
1.54440695320474));
#23340=CARTESIAN_POINT('Ctrl Pts',(0.0515221758648292,-0.168027651818985,
1.54811154955701));
#23341=CARTESIAN_POINT('Ctrl Pts',(0.10730517542569,-0.139188455936458,
1.55181614590928));
#23342=CARTESIAN_POINT('Ctrl Pts',(0.138208714976851,-0.0935153077862871,
1.55552074226154));
#23343=CARTESIAN_POINT('Ctrl Pts',(0.15663688952593,-0.0662798273674848,
1.55772984028737));
#23344=CARTESIAN_POINT('Ctrl Pts',(0.166218204462953,-0.0330583805181475,
1.5599389383132));
#23345=CARTESIAN_POINT('Ctrl Pts',(0.166368100504911,8.32215516180223E-5,
1.56214803633902));
#23346=CARTESIAN_POINT('Ctrl Pts',(0.166721717270512,0.00013247748987999,
1.54285196366098));
#23347=CARTESIAN_POINT('Ctrl Pts',(0.16631788138976,-0.0463324921623522,
1.53973800169035));
#23348=CARTESIAN_POINT('Ctrl Pts',(0.146036306492028,-0.0931065396480778,
1.53662403971971));
#23349=CARTESIAN_POINT('Ctrl Pts',(0.111564911721182,-0.124096839839778,
1.53351007774908));
#23350=CARTESIAN_POINT('Ctrl Pts',(0.0705552254983152,-0.160965161973612,
1.52980548139681));
#23351=CARTESIAN_POINT('Ctrl Pts',(0.00946237858443097,-0.175494403270137,
1.52610088504454));
#23352=CARTESIAN_POINT('Ctrl Pts',(-0.043754143626611,-0.161035180693733,
1.52239628869227));
#23353=CARTESIAN_POINT('Ctrl Pts',(-0.0969706658376549,-0.146575958117328,
1.51869169234));
#23354=CARTESIAN_POINT('Ctrl Pts',(-0.142310863345855,-0.103128271667992,
1.51498709598774));
#23355=CARTESIAN_POINT('Ctrl Pts',(-0.159024536403123,-0.0505761979513979,
1.51128249963547));
#23356=CARTESIAN_POINT('Ctrl Pts',(-0.175738209460389,0.00197587576519482,
1.5075779032832));
#23357=CARTESIAN_POINT('Ctrl Pts',(-0.163825358066725,0.0636323367490458,
1.50387330693093));
#23358=CARTESIAN_POINT('Ctrl Pts',(-0.128737966872089,0.106175754206211,
1.50016871057866));
#23359=CARTESIAN_POINT('Ctrl Pts',(-0.0936505756774527,0.148719171663375,
1.4964641142264));
#23360=CARTESIAN_POINT('Ctrl Pts',(-0.035388644681846,0.172149545593854,
1.49275951787413));
#23361=CARTESIAN_POINT('Ctrl Pts',(0.0193839233712769,0.165743833453852,
1.48905492152186));
#23362=CARTESIAN_POINT('Ctrl Pts',(0.0741564914244009,0.159338121313851,
1.48535032516959));
#23363=CARTESIAN_POINT('Ctrl Pts',(0.125439696535041,0.123096323103367,
1.48164572881732));
#23364=CARTESIAN_POINT('Ctrl Pts',(0.149763488908927,0.07360470278495,1.47794113246505));
#23365=CARTESIAN_POINT('Ctrl Pts',(0.160901714109468,0.0509417559807338,
1.4762447428637));
#23366=CARTESIAN_POINT('Ctrl Pts',(0.166386928169176,0.0255005071147636,
1.47454835326234));
#23367=CARTESIAN_POINT('Ctrl Pts',(0.166334949033457,3.80241454671915E-5,
1.47285196366098));
#23368=CARTESIAN_POINT('Origin',(0.,0.,1.3));
#23369=CARTESIAN_POINT('',(0.166582270817784,-0.000152340582006284,1.40285196366098));
#23370=CARTESIAN_POINT('',(0.166873478424592,6.71112968702338E-7,1.42214803633902));
#23371=CARTESIAN_POINT('',(0.1666,2.04026156737949E-17,1.3));
#23372=CARTESIAN_POINT('Ctrl Pts',(0.166873476951752,6.71109354370205E-7,
1.42214803633902));
#23373=CARTESIAN_POINT('Ctrl Pts',(0.166876772816304,0.0551824619258391,
1.42585504510491));
#23374=CARTESIAN_POINT('Ctrl Pts',(0.136792549878611,0.110361163623334,
1.42956205387081));
#23375=CARTESIAN_POINT('Ctrl Pts',(0.0904117910907898,0.140258570073462,
1.4332690626367));
#23376=CARTESIAN_POINT('Ctrl Pts',(0.0440612155535343,0.170136520159922,
1.43697365898897));
#23377=CARTESIAN_POINT('Ctrl Pts',(-0.0185646804667758,0.174766068965047,
1.44067825534124));
#23378=CARTESIAN_POINT('Ctrl Pts',(-0.0688048006597445,0.152028477144375,
1.4443828516935));
#23379=CARTESIAN_POINT('Ctrl Pts',(-0.119044920852713,0.129290885323702,
1.44808744804577));
#23380=CARTESIAN_POINT('Ctrl Pts',(-0.15689926521834,0.0791861528772324,
1.45179204439804));
#23381=CARTESIAN_POINT('Ctrl Pts',(-0.165043578186289,0.0246449948801753,
1.45549664075031));
#23382=CARTESIAN_POINT('Ctrl Pts',(-0.173187891154238,-0.0298961631168814,
1.45920123710258));
#23383=CARTESIAN_POINT('Ctrl Pts',(-0.15162217272451,-0.088873746664526,
1.46290583345484));
#23384=CARTESIAN_POINT('Ctrl Pts',(-0.110216096648825,-0.125296330528958,
1.46661042980711));
#23385=CARTESIAN_POINT('Ctrl Pts',(-0.0688100205731403,-0.16171891439339,
1.47031502615938));
#23386=CARTESIAN_POINT('Ctrl Pts',(-0.00756358685149875,-0.17558649857461,
1.47401962251165));
#23387=CARTESIAN_POINT('Ctrl Pts',(0.0454934276490607,-0.160552503958399,
1.47772421886392));
#23388=CARTESIAN_POINT('Ctrl Pts',(0.0985504421496201,-0.145518509342189,
1.48142881521618));
#23389=CARTESIAN_POINT('Ctrl Pts',(0.143418037429097,-0.101582935928549,
1.48513341156845));
#23390=CARTESIAN_POINT('Ctrl Pts',(0.159562302527567,-0.0488531491308943,
1.48883800792072));
#23391=CARTESIAN_POINT('Ctrl Pts',(0.164370561528649,-0.0331485958143723,
1.48994135072682));
#23392=CARTESIAN_POINT('Ctrl Pts',(0.166630970058396,-0.0166639678834416,
1.49104469353292));
#23393=CARTESIAN_POINT('Ctrl Pts',(0.166495616539739,-0.000143126867227327,
1.49214803633902));
#23394=CARTESIAN_POINT('Ctrl Pts',(0.166334949033457,3.80241454671915E-5,
1.47285196366098));
#23395=CARTESIAN_POINT('Ctrl Pts',(0.166273415497072,-0.0301047745093415,
1.47084375691007));
#23396=CARTESIAN_POINT('Ctrl Pts',(0.158451996361882,-0.0602773308783548,
1.46883555015916));
#23397=CARTESIAN_POINT('Ctrl Pts',(0.143062834518306,-0.085905647341766,
1.46682734340825));
#23398=CARTESIAN_POINT('Ctrl Pts',(0.114674008116665,-0.133182934723717,
1.46312274705598));
#23399=CARTESIAN_POINT('Ctrl Pts',(0.060531975676251,-0.16499606706127,
1.45941815070371));
#23400=CARTESIAN_POINT('Ctrl Pts',(0.00541514530056254,-0.166785584082033,
1.45571355435145));
#23401=CARTESIAN_POINT('Ctrl Pts',(-0.0497016850751255,-0.168575101102797,
1.45200895799918));
#23402=CARTESIAN_POINT('Ctrl Pts',(-0.105793313386088,-0.14034100280677,
1.44830436164691));
#23403=CARTESIAN_POINT('Ctrl Pts',(-0.137189087849022,-0.0950047843070436,
1.44459976529464));
#23404=CARTESIAN_POINT('Ctrl Pts',(-0.168584862311956,-0.0496685658073169,
1.44089516894238));
#23405=CARTESIAN_POINT('Ctrl Pts',(-0.175284782926862,0.0127697728961095,
1.43719057259011));
#23406=CARTESIAN_POINT('Ctrl Pts',(-0.154222593046579,0.0637349720094271,
1.43348597623784));
#23407=CARTESIAN_POINT('Ctrl Pts',(-0.133160403166296,0.114700171122744,
1.42978137988557));
#23408=CARTESIAN_POINT('Ctrl Pts',(-0.0843361027908238,0.154192230645953,
1.4260767835333));
#23409=CARTESIAN_POINT('Ctrl Pts',(-0.0300944098326194,0.16413738562223,
1.42237218718103));
#23410=CARTESIAN_POINT('Ctrl Pts',(0.0241472831255854,0.174082540598506,
1.41866759082877));
#23411=CARTESIAN_POINT('Ctrl Pts',(0.0838063686665219,0.154480791027852,
1.4149629944765));
#23412=CARTESIAN_POINT('Ctrl Pts',(0.121579527998707,0.114302988740736,
1.41125839812423));
#23413=CARTESIAN_POINT('Ctrl Pts',(0.150151024791829,0.0839126277146479,
1.40845625330315));
#23414=CARTESIAN_POINT('Ctrl Pts',(0.166200792747313,0.0417499637845381,
1.40565410848206));
#23415=CARTESIAN_POINT('Ctrl Pts',(0.166582270817784,-0.000152340582006284,
1.40285196366098));
#23416=CARTESIAN_POINT('Origin',(0.,0.,1.3));
#23417=CARTESIAN_POINT('',(0.16685129292948,5.5034311338048E-5,1.33285196366098));
#23418=CARTESIAN_POINT('',(0.166493658714001,0.000142704933107348,1.35214803633902));
#23419=CARTESIAN_POINT('',(0.1666,2.04026156737949E-17,1.3));
#23420=CARTESIAN_POINT('Ctrl Pts',(0.166493658714001,0.000142704933107348,
1.35214803633902));
#23421=CARTESIAN_POINT('Ctrl Pts',(0.166629086818581,0.0167362841743647,
1.35325620397237));
#23422=CARTESIAN_POINT('Ctrl Pts',(0.164348470273229,0.0332934752509887,
1.35436437160572));
#23423=CARTESIAN_POINT('Ctrl Pts',(0.159498696116421,0.0490604157264683,
1.35547253923907));
#23424=CARTESIAN_POINT('Ctrl Pts',(0.143285936322738,0.101769183257714,
1.35917713559134));
#23425=CARTESIAN_POINT('Ctrl Pts',(0.0983612975566499,0.145646425810988,
1.36288173194361));
#23426=CARTESIAN_POINT('Ctrl Pts',(0.0452847954907157,0.16061147453177,
1.36658632829587));
#23427=CARTESIAN_POINT('Ctrl Pts',(-0.00779170657521921,0.175576523252552,
1.37029092464814));
#23428=CARTESIAN_POINT('Ctrl Pts',(-0.0690200719410003,0.161629378140841,
1.37399552100041));
#23429=CARTESIAN_POINT('Ctrl Pts',(-0.11037879201089,0.125153029241032,
1.37770011735268));
#23430=CARTESIAN_POINT('Ctrl Pts',(-0.151737512080778,0.0886766803412233,
1.38140471370495));
#23431=CARTESIAN_POINT('Ctrl Pts',(-0.173226586854776,0.0296711276533176,
1.38510931005721));
#23432=CARTESIAN_POINT('Ctrl Pts',(-0.165011419406707,-0.0248594030476235,
1.38881390640948));
#23433=CARTESIAN_POINT('Ctrl Pts',(-0.156796251958638,-0.0793899337485655,
1.39251850276175));
#23434=CARTESIAN_POINT('Ctrl Pts',(-0.1188768422885,-0.129445442462543,
1.39622309911402));
#23435=CARTESIAN_POINT('Ctrl Pts',(-0.0686072232581569,-0.152117741798697,
1.39992769546629));
#23436=CARTESIAN_POINT('Ctrl Pts',(-0.0183376042278136,-0.174790041134852,
1.40363229181856));
#23437=CARTESIAN_POINT('Ctrl Pts',(0.0442822241627354,-0.170079131093183,
1.40733688817082));
#23438=CARTESIAN_POINT('Ctrl Pts',(0.0905939423885369,-0.140140986355195,
1.41104148452309));
#23439=CARTESIAN_POINT('Ctrl Pts',(0.136875502667449,-0.110222337179314,
1.41474366846173));
#23440=CARTESIAN_POINT('Ctrl Pts',(0.166870185376906,-0.0551092982940088,
1.41844585240038));
#23441=CARTESIAN_POINT('Ctrl Pts',(0.166873476951752,6.71109354370205E-7,
1.42214803633902));
#23442=CARTESIAN_POINT('Ctrl Pts',(0.166582270817784,-0.000152340582006284,
1.40285196366098));
#23443=CARTESIAN_POINT('Ctrl Pts',(0.166705128660898,-0.0136472886129686,
1.4019495121298));
#23444=CARTESIAN_POINT('Ctrl Pts',(0.165202856095667,-0.0271152318944043,
1.40104706059861));
#23445=CARTESIAN_POINT('Ctrl Pts',(0.161970345045233,-0.0401542300245841,
1.40014460906743));
#23446=CARTESIAN_POINT('Ctrl Pts',(0.148700769636142,-0.0936797914992128,
1.39644001271516));
#23447=CARTESIAN_POINT('Ctrl Pts',(0.106274385694529,-0.139977059444894,
1.39273541636289));
#23448=CARTESIAN_POINT('Ctrl Pts',(0.054107868404235,-0.157857826665655,
1.38903082001062));
#23449=CARTESIAN_POINT('Ctrl Pts',(0.00194135111394122,-0.175738593886417,
1.38532622365835));
#23450=CARTESIAN_POINT('Ctrl Pts',(-0.0599652995250327,-0.165202860382259,
1.38162162730609));
#23451=CARTESIAN_POINT('Ctrl Pts',(-0.103280153812656,-0.131072364331603,
1.37791703095382));
#23452=CARTESIAN_POINT('Ctrl Pts',(-0.146595008100279,-0.0969418682809483,
1.37421243460155));
#23453=CARTESIAN_POINT('Ctrl Pts',(-0.171318066036552,-0.0392166096837955,
1.37050783824928));
#23454=CARTESIAN_POINT('Ctrl Pts',(-0.166134679967937,0.0156851195376423,
1.36680324189701));
#23455=CARTESIAN_POINT('Ctrl Pts',(-0.160951293899322,0.0705868487590808,
1.36309864554474));
#23456=CARTESIAN_POINT('Ctrl Pts',(-0.12586146382582,0.122665048604804,
1.35939404919248));
#23457=CARTESIAN_POINT('Ctrl Pts',(-0.0769242494532953,0.14808583561233,
1.35568945284021));
#23458=CARTESIAN_POINT('Ctrl Pts',(-0.0279870350807717,0.173506622619856,
1.35198485648794));
#23459=CARTESIAN_POINT('Ctrl Pts',(0.0347975635907744,0.172269996789183,
1.34828026013567));
#23460=CARTESIAN_POINT('Ctrl Pts',(0.0826958189663461,0.144941906943662,
1.3445756637834));
#23461=CARTESIAN_POINT('Ctrl Pts',(0.130594074341918,0.117613817098141,
1.34087106743114));
#23462=CARTESIAN_POINT('Ctrl Pts',(0.163605986421516,0.0641942632377707,
1.33716647107887));
#23463=CARTESIAN_POINT('Ctrl Pts',(0.166623466451679,0.00913100709632859,
1.3334618747266));
#23464=CARTESIAN_POINT('Ctrl Pts',(0.166789062042101,0.00610920336601207,
1.33325857103806));
#23465=CARTESIAN_POINT('Ctrl Pts',(0.16686432402183,0.00308244933152886,
1.33305526734952));
#23466=CARTESIAN_POINT('Ctrl Pts',(0.16685129292948,5.5034311338048E-5,
1.33285196366098));
#23467=CARTESIAN_POINT('Origin',(0.,0.,1.3));
#23468=CARTESIAN_POINT('',(0.166419792426106,0.000117644517947116,1.26285196366098));
#23469=CARTESIAN_POINT('',(0.166369239667266,-8.42498788368234E-5,1.28214803633902));
#23470=CARTESIAN_POINT('',(0.1666,2.04026156737949E-17,1.3));
#23471=CARTESIAN_POINT('Ctrl Pts',(0.166369239667266,-8.42498788368234E-5,
1.28214803633902));
#23472=CARTESIAN_POINT('Ctrl Pts',(0.166217137033255,0.0331292003521081,
1.2843619591921));
#23473=CARTESIAN_POINT('Ctrl Pts',(0.156590960021794,0.0664238537129591,
1.28657588204517));
#23474=CARTESIAN_POINT('Ctrl Pts',(0.138087078302622,0.093694809140457,
1.28878980489824));
#23475=CARTESIAN_POINT('Ctrl Pts',(0.107124205036991,0.139327782240334,
1.29249440125051));
#23476=CARTESIAN_POINT('Ctrl Pts',(0.051303827751912,0.168094448054701,
1.29619899760278));
#23477=CARTESIAN_POINT('Ctrl Pts',(-0.00382754136500674,0.166829578855541,
1.29990359395505));
#23478=CARTESIAN_POINT('Ctrl Pts',(-0.0589589104819255,0.16556470965638,
1.30360819030732));
#23479=CARTESIAN_POINT('Ctrl Pts',(-0.113401271430684,0.134268305443692,
1.30731278665959));
#23480=CARTESIAN_POINT('Ctrl Pts',(-0.142238769013948,0.0872633430680612,
1.31101738301185));
#23481=CARTESIAN_POINT('Ctrl Pts',(-0.171076266597211,0.0402583806924305,
1.31472197936412));
#23482=CARTESIAN_POINT('Ctrl Pts',(-0.17430890081498,-0.0224551398461431,
1.31842657571639));
#23483=CARTESIAN_POINT('Ctrl Pts',(-0.150457238287118,-0.0721760202632685,
1.32213117206866));
#23484=CARTESIAN_POINT('Ctrl Pts',(-0.126605575759256,-0.121896900680394,
1.32583576842093));
#23485=CARTESIAN_POINT('Ctrl Pts',(-0.0756696164857624,-0.158625140976071,
1.32954036477319));
#23486=CARTESIAN_POINT('Ctrl Pts',(-0.0209604910548609,-0.165551853715821,
1.33324496112546));
#23487=CARTESIAN_POINT('Ctrl Pts',(0.0337486343760406,-0.17247856645557,
1.33694955747773));
#23488=CARTESIAN_POINT('Ctrl Pts',(0.0922309259643503,-0.149603751639392,
1.34065415383));
#23489=CARTESIAN_POINT('Ctrl Pts',(0.127721631347866,-0.107396197976694,
1.34435875018227));
#23490=CARTESIAN_POINT('Ctrl Pts',(0.152595889688052,-0.0778143234445287,
1.34695517890118));
#23491=CARTESIAN_POINT('Ctrl Pts',(0.166176351648266,-0.038735930748939,
1.3495516076201));
#23492=CARTESIAN_POINT('Ctrl Pts',(0.166493658714001,0.000142704933107348,
1.35214803633902));
#23493=CARTESIAN_POINT('Ctrl Pts',(0.16685129292948,5.5034311338048E-5,
1.33285196366098));
#23494=CARTESIAN_POINT('Ctrl Pts',(0.16662687167882,-0.0520830556384961,
1.32935067099725));
#23495=CARTESIAN_POINT('Ctrl Pts',(0.140215016815216,-0.104417191766459,
1.32584937833352));
#23496=CARTESIAN_POINT('Ctrl Pts',(0.0980387654551791,-0.135037607098881,
1.3223480856698));
#23497=CARTESIAN_POINT('Ctrl Pts',(0.0534135364477915,-0.167436006730135,
1.31864348931753));
#23498=CARTESIAN_POINT('Ctrl Pts',(-0.00885996954770948,-0.175525847570128,
1.31493889296526));
#23499=CARTESIAN_POINT('Ctrl Pts',(-0.0602819293976768,-0.155604768085892,
1.31123429661299));
#23500=CARTESIAN_POINT('Ctrl Pts',(-0.111703889247644,-0.135683688601655,
1.30752970026073));
#23501=CARTESIAN_POINT('Ctrl Pts',(-0.152274302952078,-0.0877516887931891,
1.30382510390846));
#23502=CARTESIAN_POINT('Ctrl Pts',(-0.163425890629257,-0.0337451201657775,
1.30012050755619));
#23503=CARTESIAN_POINT('Ctrl Pts',(-0.174577478306436,0.0202614484616345,
1.29641591120392));
#23504=CARTESIAN_POINT('Ctrl Pts',(-0.15631023995636,0.0803425859079921,
1.29271131485165));
#23505=CARTESIAN_POINT('Ctrl Pts',(-0.116984280792225,0.119001818937757,
1.28900671849938));
#23506=CARTESIAN_POINT('Ctrl Pts',(-0.077658321628091,0.157661051967521,
1.28530212214712));
#23507=CARTESIAN_POINT('Ctrl Pts',(-0.0172736416498982,0.174898380580693,
1.28159752579485));
#23508=CARTESIAN_POINT('Ctrl Pts',(0.0365343679459083,0.162825043595149,
1.27789292944258));
#23509=CARTESIAN_POINT('Ctrl Pts',(0.090342377541716,0.150751706609605,
1.27418833309031));
#23510=CARTESIAN_POINT('Ctrl Pts',(0.137573716755137,0.109367704025345,
1.27048373673804));
#23511=CARTESIAN_POINT('Ctrl Pts',(0.15661269537524,0.0576126592883118,
1.26677914038578));
#23512=CARTESIAN_POINT('Ctrl Pts',(0.163340322948393,0.0393244583837232,
1.26547008147751));
#23513=CARTESIAN_POINT('Ctrl Pts',(0.166547744893355,0.0197412896159237,
1.26416102256925));
#23514=CARTESIAN_POINT('Ctrl Pts',(0.166419792426106,0.000117644517947116,
1.26285196366098));
#23515=CARTESIAN_POINT('Origin',(0.,0.,1.3));
#23516=CARTESIAN_POINT('',(0.166426142970557,-0.000120642765556289,1.19285196366098));
#23517=CARTESIAN_POINT('',(0.16680112293357,-9.74720745467285E-5,1.21214803633902));
#23518=CARTESIAN_POINT('',(0.1666,2.04026156737949E-17,1.3));
#23519=CARTESIAN_POINT('Ctrl Pts',(0.16680112293357,-9.74720745467285E-5,
1.21214803633902));
#23520=CARTESIAN_POINT('Ctrl Pts',(0.166457232615762,0.0493755335317627,
1.21546771441182));
#23521=CARTESIAN_POINT('Ctrl Pts',(0.143044424972525,0.0991312161213854,
1.21878739248462));
#23522=CARTESIAN_POINT('Ctrl Pts',(0.104522946124804,0.130083481608585,
1.22210707055742));
#23523=CARTESIAN_POINT('Ctrl Pts',(0.0615348831579396,0.164624677261814,
1.22581166690969));
#23524=CARTESIAN_POINT('Ctrl Pts',(-0.000268695245690821,0.175749122363903,
1.22951626326196));
#23525=CARTESIAN_POINT('Ctrl Pts',(-0.0526030309795398,0.15836565153399,
1.23322085961422));
#23526=CARTESIAN_POINT('Ctrl Pts',(-0.104937366713389,0.140982180704076,
1.23692545596649));
#23527=CARTESIAN_POINT('Ctrl Pts',(-0.147802459777456,0.0950907939421611,
1.24063005231876));
#23528=CARTESIAN_POINT('Ctrl Pts',(-0.161580857269364,0.0416939446216941,
1.24433464867103));
#23529=CARTESIAN_POINT('Ctrl Pts',(-0.175359254761272,-0.0117029046987729,
1.2480392450233));
#23530=CARTESIAN_POINT('Ctrl Pts',(-0.16005095668102,-0.0726052165777916,
1.25174384137556));
#23531=CARTESIAN_POINT('Ctrl Pts',(-0.122661892448987,-0.113140702644331,
1.25544843772783));
#23532=CARTESIAN_POINT('Ctrl Pts',(-0.0852728282169544,-0.15367618871087,
1.2591530340801));
#23533=CARTESIAN_POINT('Ctrl Pts',(-0.0258029978331414,-0.17384484896493,
1.26285763043237));
#23534=CARTESIAN_POINT('Ctrl Pts',(0.0285308936104228,-0.164416381677161,
1.26656222678464));
#23535=CARTESIAN_POINT('Ctrl Pts',(0.0828647850539866,-0.154987914389393,
1.2702668231369));
#23536=CARTESIAN_POINT('Ctrl Pts',(0.132062737557302,-0.115962319559795,
1.27397141948917));
#23537=CARTESIAN_POINT('Ctrl Pts',(0.153609029185868,-0.0651998819523026,
1.27767601584144));
#23538=CARTESIAN_POINT('Ctrl Pts',(0.162278930811433,-0.044773845401895,
1.27916668934063));
#23539=CARTESIAN_POINT('Ctrl Pts',(0.166471653066795,-0.022447454634266,
1.28065736283983));
#23540=CARTESIAN_POINT('Ctrl Pts',(0.166369239667266,-8.42498788368234E-5,
1.28214803633902));
#23541=CARTESIAN_POINT('Ctrl Pts',(0.166419792426106,0.000117644517947116,
1.26285196366098));
#23542=CARTESIAN_POINT('Ctrl Pts',(0.166185643355799,-0.0357930210168177,
1.26045642621698));
#23543=CARTESIAN_POINT('Ctrl Pts',(0.154782035268061,-0.0718392331665093,
1.25806088877297));
#23544=CARTESIAN_POINT('Ctrl Pts',(0.133341646618848,-0.100333245437109,
1.25566535132897));
#23545=CARTESIAN_POINT('Ctrl Pts',(0.100185001215565,-0.144398018535696,
1.2519607549767));
#23546=CARTESIAN_POINT('Ctrl Pts',(0.0430250923822119,-0.170401477843065,
1.24825615862443));
#23547=CARTESIAN_POINT('Ctrl Pts',(-0.0119785234848996,-0.166442992757554,
1.24455156227217));
#23548=CARTESIAN_POINT('Ctrl Pts',(-0.0669821393520106,-0.162484507672042,
1.2408469659199));
#23549=CARTESIAN_POINT('Ctrl Pts',(-0.11982946225288,-0.12856407819365,
1.23714236956763));
#23550=CARTESIAN_POINT('Ctrl Pts',(-0.146334615197223,-0.0802055812150856,
1.23343777321536));
#23551=CARTESIAN_POINT('Ctrl Pts',(-0.172839768141565,-0.0318470842365214,
1.22973317686309));
#23552=CARTESIAN_POINT('Ctrl Pts',(-0.17300275112938,0.0309494802422141,
1.22602858051083));
#23553=CARTESIAN_POINT('Ctrl Pts',(-0.14674897407212,0.0794449084066994,
1.22232398415856));
#23554=CARTESIAN_POINT('Ctrl Pts',(-0.12049519701486,0.127940336571185,
1.21861938780629));
#23555=CARTESIAN_POINT('Ctrl Pts',(-0.0678246599125219,0.162134628421419,
1.21491479145402));
#23556=CARTESIAN_POINT('Ctrl Pts',(-0.01284233273225,0.166378572397304,
1.21121019510176));
#23557=CARTESIAN_POINT('Ctrl Pts',(0.0421399944480223,0.170622516373188,
1.20750559874949));
#23558=CARTESIAN_POINT('Ctrl Pts',(0.0994341117062293,0.144916112474723,
1.20380100239722));
#23559=CARTESIAN_POINT('Ctrl Pts',(0.132819041399409,0.101024042211295,
1.20009640604495));
#23560=CARTESIAN_POINT('Ctrl Pts',(0.154580764464244,0.0724133161563545,
1.19768159191696));
#23561=CARTESIAN_POINT('Ctrl Pts',(0.166183499569454,0.0360755201147432,
1.19526677778897));
#23562=CARTESIAN_POINT('Ctrl Pts',(0.166426142970557,-0.000120642765556289,
1.19285196366098));
#23563=CARTESIAN_POINT('Origin',(0.,0.,1.3));
#23564=CARTESIAN_POINT('',(0.166855124306607,-5.00565220619177E-5,1.12285196366098));
#23565=CARTESIAN_POINT('',(0.166664543572935,0.000145872469707454,1.14214803633902));
#23566=CARTESIAN_POINT('',(0.1666,2.04026156737949E-17,1.3));
#23567=CARTESIAN_POINT('Ctrl Pts',(0.166664543572935,0.000145872469707454,
1.14214803633902));
#23568=CARTESIAN_POINT('Ctrl Pts',(0.166763206461382,0.0109113832732099,
1.14286887327928));
#23569=CARTESIAN_POINT('Ctrl Pts',(0.165809417829237,0.0216594859626649,
1.14358971021953));
#23570=CARTESIAN_POINT('Ctrl Pts',(0.163739663996808,0.0321882103916611,
1.14431054715979));
#23571=CARTESIAN_POINT('Ctrl Pts',(0.153102580809897,0.0862984701957669,
1.14801514351206));
#23572=CARTESIAN_POINT('Ctrl Pts',(0.112990188231545,0.134614425572516,
1.15171973986433));
#23573=CARTESIAN_POINT('Ctrl Pts',(0.0617601501778567,0.155024005573456,
1.1554243362166));
#23574=CARTESIAN_POINT('Ctrl Pts',(0.010530112124168,0.175433585574396,
1.15912893256886));
#23575=CARTESIAN_POINT('Ctrl Pts',(-0.0518175714048562,0.167936790199525,
1.16283352892113));
#23576=CARTESIAN_POINT('Ctrl Pts',(-0.0967491295066884,0.135964570361971,
1.1665381252734));
#23577=CARTESIAN_POINT('Ctrl Pts',(-0.14168068760852,0.103992350524416,
1.17024272162567));
#23578=CARTESIAN_POINT('Ctrl Pts',(-0.16919612028316,0.0475447062241783,
1.17394731797794));
#23579=CARTESIAN_POINT('Ctrl Pts',(-0.166702833743975,-0.00754477804487655,
1.1776519143302));
#23580=CARTESIAN_POINT('Ctrl Pts',(-0.16420954720479,-0.0626342623139314,
1.18135651068247));
#23581=CARTESIAN_POINT('Ctrl Pts',(-0.131707541451779,-0.116365586551803,
1.18506110703474));
#23582=CARTESIAN_POINT('Ctrl Pts',(-0.0840715437167003,-0.144148305543673,
1.18876570338701));
#23583=CARTESIAN_POINT('Ctrl Pts',(-0.0364355459816213,-0.171931024535542,
1.19247029973928));
#23584=CARTESIAN_POINT('Ctrl Pts',(0.0263344437355261,-0.17376513828141,
1.19617489609154));
#23585=CARTESIAN_POINT('Ctrl Pts',(0.0755113837106313,-0.148811254225361,
1.19987949244381));
#23586=CARTESIAN_POINT('Ctrl Pts',(0.124688323685737,-0.123857370169311,
1.20358408879608));
#23587=CARTESIAN_POINT('Ctrl Pts',(0.1602722139188,-0.0721154883113449,
1.20728868514835));
#23588=CARTESIAN_POINT('Ctrl Pts',(0.165977885270282,-0.0172655742801778,
1.21099328150062));
#23589=CARTESIAN_POINT('Ctrl Pts',(0.166570721031857,-0.011566509515692,
1.21137819978008));
#23590=CARTESIAN_POINT('Ctrl Pts',(0.166840997182384,-0.00583389102255577,
1.21176311805955));
#23591=CARTESIAN_POINT('Ctrl Pts',(0.16680112293357,-9.74720745467285E-5,
1.21214803633902));
#23592=CARTESIAN_POINT('Ctrl Pts',(0.166426142970557,-0.000120642765556289,
1.19285196366098));
#23593=CARTESIAN_POINT('Ctrl Pts',(0.166555741825373,-0.0194534630140944,
1.1915621814367));
#23594=CARTESIAN_POINT('Ctrl Pts',(0.163444578249431,-0.0387458787095636,
1.19027239921243));
#23595=CARTESIAN_POINT('Ctrl Pts',(0.156909640667809,-0.0567989395012422,
1.18898261698815));
#23596=CARTESIAN_POINT('Ctrl Pts',(0.138139568114877,-0.108652114321963,
1.18527802063588));
#23597=CARTESIAN_POINT('Ctrl Pts',(0.0911236808808596,-0.150280727335013,
1.18157342428361));
#23598=CARTESIAN_POINT('Ctrl Pts',(0.0373790663566119,-0.162633207744568,
1.17786882793134));
#23599=CARTESIAN_POINT('Ctrl Pts',(-0.0163655481676351,-0.174985688154123,
1.17416423157907));
#23600=CARTESIAN_POINT('Ctrl Pts',(-0.0768388899821125,-0.158062035960183,
1.17045963522681));
#23601=CARTESIAN_POINT('Ctrl Pts',(-0.116364991298242,-0.119607456553155,
1.16675503887454));
#23602=CARTESIAN_POINT('Ctrl Pts',(-0.155891092614372,-0.0811528771461272,
1.16305044252227));
#23603=CARTESIAN_POINT('Ctrl Pts',(-0.174469953432153,-0.0211673705260111,
1.15934584617));
#23604=CARTESIAN_POINT('Ctrl Pts',(-0.163598852749046,0.0328963560619538,
1.15564124981773));
#23605=CARTESIAN_POINT('Ctrl Pts',(-0.152727752065939,0.0869600826499182,
1.15193665346547));
#23606=CARTESIAN_POINT('Ctrl Pts',(-0.112406689881943,0.135102029205731,
1.1482320571132));
#23607=CARTESIAN_POINT('Ctrl Pts',(-0.061088828941493,0.155289760903929,
1.14452746076093));
#23608=CARTESIAN_POINT('Ctrl Pts',(-0.00977096800104246,0.175477492602127,
1.14082286440866));
#23609=CARTESIAN_POINT('Ctrl Pts',(0.0525436916958626,0.16771100944271,
1.13711826805639));
#23610=CARTESIAN_POINT('Ctrl Pts',(0.0973364927906947,0.135544686484056,
1.13341367170413));
#23611=CARTESIAN_POINT('Ctrl Pts',(0.139904197214479,0.10497623587064,1.12989310235641));
#23612=CARTESIAN_POINT('Ctrl Pts',(0.166647613265987,0.0523718751412305,
1.12637253300869));
#23613=CARTESIAN_POINT('Ctrl Pts',(0.166855124306607,-5.00565220619177E-5,
1.12285196366098));
#23614=CARTESIAN_POINT('Origin',(0.,0.,1.3));
#23615=CARTESIAN_POINT('',(0.166573628657937,0.000152187718365226,1.05285196366098));
#23616=CARTESIAN_POINT('',(0.166327182499917,6.33242585386815E-6,1.07214803633902));
#23617=CARTESIAN_POINT('',(0.1666,2.04026156737949E-17,1.3));
#23618=CARTESIAN_POINT('Ctrl Pts',(0.166327182499917,6.33242585386815E-6,
1.07214803633902));
#23619=CARTESIAN_POINT('Ctrl Pts',(0.166336479007403,0.0274263312352492,
1.073974628499));
#23620=CARTESIAN_POINT('Ctrl Pts',(0.159932481000657,0.0548422420648042,
1.07580122065898));
#23621=CARTESIAN_POINT('Ctrl Pts',(0.147091342637332,0.0788092340673142,
1.07762781281897));
#23622=CARTESIAN_POINT('Ctrl Pts',(0.121047633821556,0.127417803124253,
1.08133240917123));
#23623=CARTESIAN_POINT('Ctrl Pts',(0.0685255340861956,0.161839665678967,
1.0850370055235));
#23624=CARTESIAN_POINT('Ctrl Pts',(0.0135620801901698,0.166321461139012,
1.08874160187577));
#23625=CARTESIAN_POINT('Ctrl Pts',(-0.0414013737058552,0.170803256599056,
1.09244619822804));
#23626=CARTESIAN_POINT('Ctrl Pts',(-0.0988061817625453,0.145344984964431,
1.09615079458031));
#23627=CARTESIAN_POINT('Ctrl Pts',(-0.132380708062468,0.101597768611665,
1.09985539093257));
#23628=CARTESIAN_POINT('Ctrl Pts',(-0.165955234362392,0.0578505522588977,
1.10355998728484));
#23629=CARTESIAN_POINT('Ctrl Pts',(-0.175699478905547,-0.00418560881201081,
1.10726458363711));
#23630=CARTESIAN_POINT('Ctrl Pts',(-0.157153932924644,-0.0561195137204682,
1.11096917998938));
#23631=CARTESIAN_POINT('Ctrl Pts',(-0.13860838694374,-0.108053418628926,
1.11467377634165));
#23632=CARTESIAN_POINT('Ctrl Pts',(-0.0917730504387764,-0.149885067374932,
1.11837837269391));
#23633=CARTESIAN_POINT('Ctrl Pts',(-0.0380823807348833,-0.162469968707007,
1.12208296904618));
#23634=CARTESIAN_POINT('Ctrl Pts',(0.0156082889690095,-0.175054870039082,
1.12578756539845));
#23635=CARTESIAN_POINT('Ctrl Pts',(0.076154291871832,-0.158393023957226,
1.12949216175072));
#23636=CARTESIAN_POINT('Ctrl Pts',(0.115846406425509,-0.120109818800568,
1.13319675810299));
#23637=CARTESIAN_POINT('Ctrl Pts',(0.147815265950422,-0.0892757243821015,
1.136180517515));
#23638=CARTESIAN_POINT('Ctrl Pts',(0.16625614840673,-0.044415792438328,
1.13916427692701));
#23639=CARTESIAN_POINT('Ctrl Pts',(0.166664543572935,0.000145872469707454,
1.14214803633902));
#23640=CARTESIAN_POINT('Ctrl Pts',(0.166855124306607,-5.00565220619177E-5,
1.12285196366098));
#23641=CARTESIAN_POINT('Ctrl Pts',(0.166865971312146,-0.00279025280966625,
1.12266793665643));
#23642=CARTESIAN_POINT('Ctrl Pts',(0.166804312774377,-0.00552995063608946,
1.12248390965187));
#23643=CARTESIAN_POINT('Ctrl Pts',(0.166668618800564,-0.00826597665440976,
1.12229988264732));
#23644=CARTESIAN_POINT('Ctrl Pts',(0.163937001222843,-0.0633441540763332,
1.11859528629505));
#23645=CARTESIAN_POINT('Ctrl Pts',(0.131202823574641,-0.116934346162291,
1.11489068994278));
#23646=CARTESIAN_POINT('Ctrl Pts',(0.0834470678717536,-0.144510697621526,
1.11118609359052));
#23647=CARTESIAN_POINT('Ctrl Pts',(0.035691312168866,-0.172087049080761,
1.10748149723825));
#23648=CARTESIAN_POINT('Ctrl Pts',(-0.0270860215887074,-0.173649559913274,
1.10377690088598));
#23649=CARTESIAN_POINT('Ctrl Pts',(-0.0761545306345133,-0.148483138187173,
1.10007230453371));
#23650=CARTESIAN_POINT('Ctrl Pts',(-0.125223039680319,-0.123316716461072,
1.09636770818145));
#23651=CARTESIAN_POINT('Ctrl Pts',(-0.160582724014357,-0.0714213621763564,
1.09266311182918));
#23652=CARTESIAN_POINT('Ctrl Pts',(-0.166051023599269,-0.0165472784677163,
1.08895851547691));
#23653=CARTESIAN_POINT('Ctrl Pts',(-0.171519323184182,0.0383268052409238,
1.08525391912464));
#23654=CARTESIAN_POINT('Ctrl Pts',(-0.147096238019968,0.0961796183734885,
1.08154932277237));
#23655=CARTESIAN_POINT('Ctrl Pts',(-0.103959131518119,0.130534492913072,
1.0778447264201));
#23656=CARTESIAN_POINT('Ctrl Pts',(-0.0608220250162706,0.164889367452656,
1.07414013006784));
#23657=CARTESIAN_POINT('Ctrl Pts',(0.0010291028232132,0.175746303399259,
1.07043553371557));
#23658=CARTESIAN_POINT('Ctrl Pts',(0.0532877326205867,0.15813656252862,
1.0667309373633));
#23659=CARTESIAN_POINT('Ctrl Pts',(0.10554636241796,0.140526821657981,1.06302634101103));
#23660=CARTESIAN_POINT('Ctrl Pts',(0.148212494173223,0.0944504039700999,
1.05932174465876));
#23661=CARTESIAN_POINT('Ctrl Pts',(0.161759730763308,0.0409944431478461,
1.0556171483065));
#23662=CARTESIAN_POINT('Ctrl Pts',(0.165130373342236,0.0276942445097812,
1.05469542009132));
#23663=CARTESIAN_POINT('Ctrl Pts',(0.16669841799434,0.0139372170985273,
1.05377369187615));
#23664=CARTESIAN_POINT('Ctrl Pts',(0.166573628657937,0.000152187718365227,
1.05285196366098));
#23665=CARTESIAN_POINT('Origin',(0.,0.,1.3));
#23666=CARTESIAN_POINT('',(0.16633703813182,-4.26131537097363E-5,0.982851963660979));
#23667=CARTESIAN_POINT('',(0.166641299058679,-0.000149160109009599,1.00214803633902));
#23668=CARTESIAN_POINT('',(0.1666,2.04026156737949E-17,1.3));
#23669=CARTESIAN_POINT('Ctrl Pts',(0.166641299058679,-0.000149160109009599,
1.00214803633902));
#23670=CARTESIAN_POINT('Ctrl Pts',(0.166236990763482,0.0436603970157784,
1.00508038371873));
#23671=CARTESIAN_POINT('Ctrl Pts',(0.148493576846311,0.0877597158867868,
1.00801273109843));
#23672=CARTESIAN_POINT('Ctrl Pts',(0.117498076053599,0.118494559065924,
1.01094507847814));
#23673=CARTESIAN_POINT('Ctrl Pts',(0.0783397485075339,0.157323583456734,
1.01464967483041));
#23674=CARTESIAN_POINT('Ctrl Pts',(0.0180302104029479,0.174822017275825,
1.01835427118268));
#23675=CARTESIAN_POINT('Ctrl Pts',(-0.0358295364409326,0.162981602616999,
1.02205886753494));
#23676=CARTESIAN_POINT('Ctrl Pts',(-0.089689283284813,0.151141187958173,
1.02576346388721));
#23677=CARTESIAN_POINT('Ctrl Pts',(-0.137099238867988,0.10996192482143,
1.02946806023948));
#23678=CARTESIAN_POINT('Ctrl Pts',(-0.156361968042692,0.0582897367165174,
1.03317265659175));
#23679=CARTESIAN_POINT('Ctrl Pts',(-0.175624697217396,0.00661754861160513,
1.03687725294402));
#23680=CARTESIAN_POINT('Ctrl Pts',(-0.166740199983629,-0.0555475644614757,
1.04058184929629));
#23681=CARTESIAN_POINT('Ctrl Pts',(-0.133774516953309,-0.0997553861262926,
1.04428644564855));
#23682=CARTESIAN_POINT('Ctrl Pts',(-0.100808833922988,-0.143963207791109,
1.04799104200082));
#23683=CARTESIAN_POINT('Ctrl Pts',(-0.0437619650961137,-0.170213738047662,
1.05169563835309));
#23684=CARTESIAN_POINT('Ctrl Pts',(0.0112582665697782,-0.166493272809894,
1.05540023470536));
#23685=CARTESIAN_POINT('Ctrl Pts',(0.0662784982356701,-0.162772807572126,
1.05910483105763));
#23686=CARTESIAN_POINT('Ctrl Pts',(0.11927209274058,-0.129081346840038,
1.06280942740989));
#23687=CARTESIAN_POINT('Ctrl Pts',(0.145986231044939,-0.0808379786944121,
1.06651402376216));
#23688=CARTESIAN_POINT('Ctrl Pts',(0.159528668319701,-0.0563815362072228,
1.06839202795445));
#23689=CARTESIAN_POINT('Ctrl Pts',(0.166317624329016,-0.0281854412194699,
1.07027003214673));
#23690=CARTESIAN_POINT('Ctrl Pts',(0.166327182499917,6.33242585386815E-6,
1.07214803633902));
#23691=CARTESIAN_POINT('Ctrl Pts',(0.166573628657937,0.000152187718365227,
1.05285196366098));
#23692=CARTESIAN_POINT('Ctrl Pts',(0.166196866546928,-0.0414673682413184,
1.05006909552388));
#23693=CARTESIAN_POINT('Ctrl Pts',(0.150389111841613,-0.0833421755592448,
1.04728622738679));
#23694=CARTESIAN_POINT('Ctrl Pts',(0.122171212866625,-0.113670355101641,
1.04450335924969));
#23695=CARTESIAN_POINT('Ctrl Pts',(0.0846071169549502,-0.154043688572246,
1.04079876289742));
#23696=CARTESIAN_POINT('Ctrl Pts',(0.0250505837066941,-0.173954851556829,
1.03709416654516));
#23697=CARTESIAN_POINT('Ctrl Pts',(-0.0292420016986911,-0.164291387935873,
1.03338957019289));
#23698=CARTESIAN_POINT('Ctrl Pts',(-0.0835345871040766,-0.154627924314917,
1.02968497384062));
#23699=CARTESIAN_POINT('Ctrl Pts',(-0.132563224666591,-0.115389834088422,
1.02598037748835));
#23700=CARTESIAN_POINT('Ctrl Pts',(-0.153889680451665,-0.0645346507397467,
1.02227578113608));
#23701=CARTESIAN_POINT('Ctrl Pts',(-0.175216136236738,-0.0136794673910717,
1.01857118478382));
#23702=CARTESIAN_POINT('Ctrl Pts',(-0.16884041024437,0.0487928090797828,
1.01486658843155));
#23703=CARTESIAN_POINT('Ctrl Pts',(-0.137680389518285,0.0942913851820011,
1.01116199207928));
#23704=CARTESIAN_POINT('Ctrl Pts',(-0.106520368792199,0.139789961284219,
1.00745739572701));
#23705=CARTESIAN_POINT('Ctrl Pts',(-0.0505760533323975,0.168314837017802,
1.00375279937474));
#23706=CARTESIAN_POINT('Ctrl Pts',(0.00454932345543924,0.166811444936069,
1.00004820302248));
#23707=CARTESIAN_POINT('Ctrl Pts',(0.0596747002432758,0.165308052854335,
0.996343606670208));
#23708=CARTESIAN_POINT('Ctrl Pts',(0.113981138359147,0.133776392957287,
0.992639010317939));
#23709=CARTESIAN_POINT('Ctrl Pts',(0.142614988862282,0.0866471011481969,
0.988934413965671));
#23710=CARTESIAN_POINT('Ctrl Pts',(0.158285969463688,0.0608537759501981,
0.986906930530773));
#23711=CARTESIAN_POINT('Ctrl Pts',(0.166267372459907,0.0303885726052033,
0.984879447095876));
#23712=CARTESIAN_POINT('Ctrl Pts',(0.16633703813182,-4.26131537097363E-5,
0.982851963660979));
#23713=CARTESIAN_POINT('Origin',(0.,0.,1.3));
#23714=CARTESIAN_POINT('',(0.166729862742343,-0.000130123946020723,0.912851963660979));
#23715=CARTESIAN_POINT('',(0.16681765906064,8.64047405809373E-5,0.93214803633902));
#23716=CARTESIAN_POINT('',(0.1666,2.04026156737949E-17,1.3));
#23717=CARTESIAN_POINT('Ctrl Pts',(0.16681765906064,8.64047405809373E-5,
0.93214803633902));
#23718=CARTESIAN_POINT('Ctrl Pts',(0.166849023174239,0.00505533653555562,
0.932481542586184));
#23719=CARTESIAN_POINT('Ctrl Pts',(0.166646252238729,0.0100216728157887,
0.932815048833348));
#23720=CARTESIAN_POINT('Ctrl Pts',(0.166201007638075,0.0149661744225974,
0.933148555080512));
#23721=CARTESIAN_POINT('Ctrl Pts',(0.161255218653678,0.0698898310921401,
0.93685315143278));
#23722=CARTESIAN_POINT('Ctrl Pts',(0.126391025843356,0.122119345383236,
0.940557747785048));
#23723=CARTESIAN_POINT('Ctrl Pts',(0.0775642504900456,0.147751626038697,
0.944262344137316));
#23724=CARTESIAN_POINT('Ctrl Pts',(0.0287374751367354,0.173383906694158,
0.947966940489584));
#23725=CARTESIAN_POINT('Ctrl Pts',(-0.0340518827595631,0.172418953713984,
0.951671536841852));
#23726=CARTESIAN_POINT('Ctrl Pts',(-0.0820679309643883,0.145298361306226,
0.95537613319412));
#23727=CARTESIAN_POINT('Ctrl Pts',(-0.130083979169214,0.118177768898468,
0.959080729546388));
#23728=CARTESIAN_POINT('Ctrl Pts',(-0.163326717682566,0.0649015370631265,
0.962785325898656));
#23729=CARTESIAN_POINT('Ctrl Pts',(-0.166582411702781,0.00985184688226562,
0.966489922250924));
#23730=CARTESIAN_POINT('Ctrl Pts',(-0.169838105722997,-0.045197843298595,
0.970194518603192));
#23731=CARTESIAN_POINT('Ctrl Pts',(-0.143106755250076,-0.102020991824975,
0.97389911495546));
#23732=CARTESIAN_POINT('Ctrl Pts',(-0.0986221180718627,-0.134612168562546,
0.977603711307728));
#23733=CARTESIAN_POINT('Ctrl Pts',(-0.054137480893649,-0.167203345300117,
0.981308307659997));
#23734=CARTESIAN_POINT('Ctrl Pts',(0.00810044298985758,-0.175562550248879,
0.985012904012265));
#23735=CARTESIAN_POINT('Ctrl Pts',(0.0596081167151753,-0.155864142731977,
0.988717500364533));
#23736=CARTESIAN_POINT('Ctrl Pts',(0.111115790440493,-0.136165735215075,
0.992422096716801));
#23737=CARTESIAN_POINT('Ctrl Pts',(0.151893214007622,-0.0884097152325082,
0.996126693069068));
#23738=CARTESIAN_POINT('Ctrl Pts',(0.163278367297414,-0.0344518977599609,
0.999831289421336));
#23739=CARTESIAN_POINT('Ctrl Pts',(0.165651681983942,-0.0232040140116242,
1.0006035383939));
#23740=CARTESIAN_POINT('Ctrl Pts',(0.166747775756401,-0.0116866354136458,
1.00137578736646));
#23741=CARTESIAN_POINT('Ctrl Pts',(0.166641299058679,-0.000149160109009599,
1.00214803633902));
#23742=CARTESIAN_POINT('Ctrl Pts',(0.16633703813182,-4.26131537097363E-5,
0.982851963660979));
#23743=CARTESIAN_POINT('Ctrl Pts',(0.166394664840996,-0.0252149691141755,
0.981174850743608));
#23744=CARTESIAN_POINT('Ctrl Pts',(0.161038745460081,-0.0503640488000913,
0.979497737826238));
#23745=CARTESIAN_POINT('Ctrl Pts',(0.150143538011669,-0.0728263241997442,
0.977820624908867));
#23746=CARTESIAN_POINT('Ctrl Pts',(0.126076973767522,-0.122443534017465,
0.974116028556599));
#23747=CARTESIAN_POINT('Ctrl Pts',(0.0749825823888285,-0.158951029931774,
0.970411432204331));
#23748=CARTESIAN_POINT('Ctrl Pts',(0.0202440032863241,-0.165640975250716,
0.966706835852062));
#23749=CARTESIAN_POINT('Ctrl Pts',(-0.0344945758161804,-0.172330920569658,
0.963002239499794));
#23750=CARTESIAN_POINT('Ctrl Pts',(-0.0928773426424964,-0.149203315293232,
0.959297643147526));
#23751=CARTESIAN_POINT('Ctrl Pts',(-0.128185095718787,-0.106842589675449,
0.955593046795258));
#23752=CARTESIAN_POINT('Ctrl Pts',(-0.163492848795077,-0.064481864057666,
0.95188845044299));
#23753=CARTESIAN_POINT('Ctrl Pts',(-0.175725588121342,-0.00288801809852563,
0.948183854090722));
#23754=CARTESIAN_POINT('Ctrl Pts',(-0.159284925787188,0.0497500806758803,
0.944479257738454));
#23755=CARTESIAN_POINT('Ctrl Pts',(-0.142844263453034,0.102388179450286,
0.940774661386186));
#23756=CARTESIAN_POINT('Ctrl Pts',(-0.097730199458461,0.146070531039958,
0.937070065033918));
#23757=CARTESIAN_POINT('Ctrl Pts',(-0.0445894513306832,0.160805840780395,
0.93336546868165));
#23758=CARTESIAN_POINT('Ctrl Pts',(0.00855129679709463,0.175541150520831,
0.929660872329382));
#23759=CARTESIAN_POINT('Ctrl Pts',(0.0697187290580771,0.161329418412033,
0.925956275977114));
#23760=CARTESIAN_POINT('Ctrl Pts',(0.110919243004777,0.124674377251528,
0.922251679624846));
#23761=CARTESIAN_POINT('Ctrl Pts',(0.145765426127824,0.093672621343478,
0.919118440970224));
#23762=CARTESIAN_POINT('Ctrl Pts',(0.16632871557528,0.0466165403829395,
0.915985202315602));
#23763=CARTESIAN_POINT('Ctrl Pts',(0.166729862742343,-0.000130123946020723,
0.912851963660979));
#23764=CARTESIAN_POINT('Origin',(0.,0.,1.3));
#23765=CARTESIAN_POINT('',(0.166745353727506,0.000120148921586877,0.842851963660979));
#23766=CARTESIAN_POINT('',(0.166381444272219,9.40568719243839E-5,0.86214803633902));
#23767=CARTESIAN_POINT('',(0.1666,2.04026156737949E-17,1.3));
#23768=CARTESIAN_POINT('',(-0.126907087985236,0.107935865304853,0.8));
#23769=CARTESIAN_POINT('Ctrl Pts',(0.166745353727506,0.000120148921586877,
0.842851963660979));
#23770=CARTESIAN_POINT('Ctrl Pts',(0.166350216338014,-0.0471541035618327,
0.83968176483079));
#23771=CARTESIAN_POINT('Ctrl Pts',(0.14523873930488,-0.0947247812496833,
0.836511566000602));
#23772=CARTESIAN_POINT('Ctrl Pts',(0.109671969299941,-0.125754000901643,
0.833341367170413));
#23773=CARTESIAN_POINT('Ctrl Pts',(0.0681097413514803,-0.162013787777386,
0.829636770818145));
#23774=CARTESIAN_POINT('Ctrl Pts',(0.00680803444401046,-0.175685325249421,
0.825932174465876));
#23775=CARTESIAN_POINT('Ctrl Pts',(-0.0461862781086293,-0.160386912096395,
0.822227578113608));
#23776=CARTESIAN_POINT('Ctrl Pts',(-0.0991805906612692,-0.14508849894337,
0.81852298176134));
#23777=CARTESIAN_POINT('Ctrl Pts',(-0.143867508859079,-0.100820135165284,
0.814818385409072));
#23778=CARTESIAN_POINT('Ctrl Pts',(-0.159771943968926,-0.0481139506034528,
0.811113789056804));
#23779=CARTESIAN_POINT('Ctrl Pts',(-0.175676379078773,0.00459223395837816,
0.807409192704537));
#23780=CARTESIAN_POINT('Ctrl Pts',(-0.162798331100657,0.0657362393039545,
0.803704596352268));
#23781=CARTESIAN_POINT('Ctrl Pts',(-0.126907087985236,0.107935865304854,
0.8));
#23782=CARTESIAN_POINT('',(0.127144529223414,0.10812516429919,0.8));
#23783=CARTESIAN_POINT('Origin',(0.,0.,0.8));
#23784=CARTESIAN_POINT('Ctrl Pts',(0.127144588893496,0.108125211870903,
0.8));
#23785=CARTESIAN_POINT('Ctrl Pts',(0.0920578520263333,0.149281442964014,
0.803632291818556));
#23786=CARTESIAN_POINT('Ctrl Pts',(0.0350626176413565,0.171873117908773,
0.807264583637111));
#23787=CARTESIAN_POINT('Ctrl Pts',(-0.0186760721562392,0.165810809841732,
0.810896875455666));
#23788=CARTESIAN_POINT('Ctrl Pts',(-0.0734844862772781,0.159627825248711,
0.814601471807934));
#23789=CARTESIAN_POINT('Ctrl Pts',(-0.124905415613006,0.123638729028309,
0.818306068160202));
#23790=CARTESIAN_POINT('Ctrl Pts',(-0.14943866399484,0.0742601129650432,
0.82201066451247));
#23791=CARTESIAN_POINT('Ctrl Pts',(-0.173971912376674,0.0248814969017771,
0.825715260864738));
#23792=CARTESIAN_POINT('Ctrl Pts',(-0.171617479804614,-0.0378866390043534,
0.829419857217006));
#23793=CARTESIAN_POINT('Ctrl Pts',(-0.143435789399569,-0.0852901107552215,
0.833124453569274));
#23794=CARTESIAN_POINT('Ctrl Pts',(-0.115254098994523,-0.132693582506089,
0.836829049921542));
#23795=CARTESIAN_POINT('Ctrl Pts',(-0.0612451507564931,-0.164732390101695,
0.84053364627381));
#23796=CARTESIAN_POINT('Ctrl Pts',(-0.00613536544337925,-0.166758384009028,
0.844238242626078));
#23797=CARTESIAN_POINT('Ctrl Pts',(0.0489744198697346,-0.168784377916361,
0.847942838978346));
#23798=CARTESIAN_POINT('Ctrl Pts',(0.105185042257932,-0.140797558135422,
0.851647435330614));
#23799=CARTESIAN_POINT('Ctrl Pts',(0.136776048425978,-0.0955986339274043,
0.855352031682883));
#23800=CARTESIAN_POINT('Ctrl Pts',(0.156093728823978,-0.0679598063592257,
0.857617366568262));
#23801=CARTESIAN_POINT('Ctrl Pts',(0.166205550297931,-0.0338849643656092,
0.859882701453641));
#23802=CARTESIAN_POINT('Ctrl Pts',(0.166381444272219,9.40568719243839E-5,
0.86214803633902));
#23803=CARTESIAN_POINT('Origin',(0.,0.,0.645407471946233));
#23804=CARTESIAN_POINT('',(0.205717919156333,0.000119231682504745,1.65459252805377));
#23805=CARTESIAN_POINT('',(0.20515534870289,-8.10795385496472E-5,1.66040747194623));
#23806=CARTESIAN_POINT('',(0.205475,1.17874941047504E-14,0.645407471946233));
#23807=CARTESIAN_POINT('',(-0.188262750966373,-0.0823232180103128,1.7));
#23808=CARTESIAN_POINT('Ctrl Pts',(0.20515534870289,-8.1079538549661E-5,
1.66040747194623));
#23809=CARTESIAN_POINT('Ctrl Pts',(0.205035475209089,0.0384765991859779,
1.66249119224068));
#23810=CARTESIAN_POINT('Ctrl Pts',(0.176046579400947,0.14575433740106,1.6682795088874));
#23811=CARTESIAN_POINT('Ctrl Pts',(0.00300247275662535,0.243001989931863,
1.67777242188639));
#23812=CARTESIAN_POINT('Ctrl Pts',(-0.202554499717183,0.133854462473394,
1.6888862109432));
#23813=CARTESIAN_POINT('Ctrl Pts',(-0.215637179506013,-0.0197213743559566,
1.69629540364773));
#23814=CARTESIAN_POINT('Ctrl Pts',(-0.188262750966373,-0.0823232180103128,
1.7));
#23815=CARTESIAN_POINT('',(-0.122364587709818,-0.165532040449643,1.7));
#23816=CARTESIAN_POINT('Origin',(0.,0.,1.7));
#23817=CARTESIAN_POINT('Ctrl Pts',(0.205717919156333,0.000119231682504748,
1.65459252805377));
#23818=CARTESIAN_POINT('Ctrl Pts',(0.205768208325854,0.00728313946640584,
1.65498227116049));
#23819=CARTESIAN_POINT('Ctrl Pts',(0.202179510783538,0.0824912465572326,
1.65907661061947));
#23820=CARTESIAN_POINT('Ctrl Pts',(0.109634140470589,0.216730418270261,
1.66687554643072));
#23821=CARTESIAN_POINT('Ctrl Pts',(-0.122663843019391,0.209602590285094,
1.67798933548753));
#23822=CARTESIAN_POINT('Ctrl Pts',(-0.24177601945125,0.0120092944511596,
1.68903082001062));
#23823=CARTESIAN_POINT('Ctrl Pts',(-0.175954082167323,-0.125816077227026,
1.69636770818144));
#23824=CARTESIAN_POINT('Ctrl Pts',(-0.122364641233049,-0.165532117868825,
1.7));
#23825=CARTESIAN_POINT('Origin',(0.,0.,0.645407471946233));
#23826=CARTESIAN_POINT('',(0.2051889883028,0.000102640746213675,1.58459252805377));
#23827=CARTESIAN_POINT('',(0.205663604651154,-0.000149728163284854,1.59040747194623));
#23828=CARTESIAN_POINT('',(0.205475,1.17874941047504E-14,0.645407471946233));
#23829=CARTESIAN_POINT('Ctrl Pts',(0.205663604651154,-0.000149728163284867,
1.59040747194623));
#23830=CARTESIAN_POINT('Ctrl Pts',(0.205182444335985,0.0585183956951034,
1.59359694746041));
#23831=CARTESIAN_POINT('Ctrl Pts',(0.148135327616145,0.186146531383155,
1.60049101932685));
#23832=CARTESIAN_POINT('Ctrl Pts',(-0.0684290720584363,0.233024356666725,
1.61108968754557));
#23833=CARTESIAN_POINT('Ctrl Pts',(-0.23288917800895,0.0688795811193509,
1.62220347660237));
#23834=CARTESIAN_POINT('Ctrl Pts',(-0.184175405168835,-0.158290127824162,
1.63331726565918));
#23835=CARTESIAN_POINT('Ctrl Pts',(0.0331013206128567,-0.240615925517378,
1.64443105471598));
#23836=CARTESIAN_POINT('Ctrl Pts',(0.185046630854554,-0.128496885183325,
1.65346112347833));
#23837=CARTESIAN_POINT('Ctrl Pts',(0.205248595419634,-0.0300741733602017,
1.65878659588842));
#23838=CARTESIAN_POINT('Ctrl Pts',(0.20515534870289,-8.1079538549661E-5,
1.66040747194623));
#23839=CARTESIAN_POINT('Ctrl Pts',(0.2051889883028,0.000102640746213654,
1.58459252805377));
#23840=CARTESIAN_POINT('Ctrl Pts',(0.205314142408481,0.0277738688435417,
1.58608802638021));
#23841=CARTESIAN_POINT('Ctrl Pts',(0.187212802641802,0.123834372120327,
1.59128812105892));
#23842=CARTESIAN_POINT('Ctrl Pts',(0.041212233239435,0.2393392912824,1.6001928120899));
#23843=CARTESIAN_POINT('Ctrl Pts',(-0.178731921787321,0.164428017156146,
1.6113066011467));
#23844=CARTESIAN_POINT('Ctrl Pts',(-0.235078089364662,-0.0609842187918821,
1.62242039020351));
#23845=CARTESIAN_POINT('Ctrl Pts',(-0.0762596568913861,-0.230580482955351,
1.63353417926032));
#23846=CARTESIAN_POINT('Ctrl Pts',(0.144352083897931,-0.190571029763675,
1.6442582252104));
#23847=CARTESIAN_POINT('Ctrl Pts',(0.205290198398921,-0.0608114238158697,
1.65127767480822));
#23848=CARTESIAN_POINT('Ctrl Pts',(0.205717919156333,0.000119231682504748,
1.65459252805377));
#23849=CARTESIAN_POINT('Origin',(0.,0.,0.645407471946233));
#23850=CARTESIAN_POINT('',(0.205346259354759,-0.00017652456807675,1.51459252805377));
#23851=CARTESIAN_POINT('',(0.205625119184624,0.000163390229490382,1.52040747194623));
#23852=CARTESIAN_POINT('',(0.205475,1.17874941047504E-14,0.645407471946233));
#23853=CARTESIAN_POINT('Ctrl Pts',(0.205625119184624,0.000163390229490371,
1.52040747194623));
#23854=CARTESIAN_POINT('Ctrl Pts',(0.205719589271595,0.0110330279545173,
1.52099810632787));
#23855=CARTESIAN_POINT('Ctrl Pts',(0.199992588366042,0.0899798330776656,
1.52529333706177));
#23856=CARTESIAN_POINT('Ctrl Pts',(0.0977367556084749,0.222326520064881,
1.53329316414794));
#23857=CARTESIAN_POINT('Ctrl Pts',(-0.133782052044684,0.202691772286445,
1.54440695320474));
#23858=CARTESIAN_POINT('Ctrl Pts',(-0.242848712699985,-0.00246927953082339,
1.55552074226155));
#23859=CARTESIAN_POINT('Ctrl Pts',(-0.129633034711377,-0.205369738746763,
1.56663453131835));
#23860=CARTESIAN_POINT('Ctrl Pts',(0.102236927935064,-0.220293776124516,
1.57774832037515));
#23861=CARTESIAN_POINT('Ctrl Pts',(0.20084133199376,-0.0871629660671419,
1.58567263391778));
#23862=CARTESIAN_POINT('Ctrl Pts',(0.205741315141077,-0.00962500803198312,
1.58989235110814));
#23863=CARTESIAN_POINT('Ctrl Pts',(0.205663604651154,-0.000149728163284867,
1.59040747194623));
#23864=CARTESIAN_POINT('Ctrl Pts',(0.205346259354759,-0.000176524568076758,
1.51459252805377));
#23865=CARTESIAN_POINT('Ctrl Pts',(0.204952685935524,0.0478618563462208,
1.51719378159994));
#23866=CARTESIAN_POINT('Ctrl Pts',(0.164184854806731,0.1649162911311,1.52349963149837));
#23867=CARTESIAN_POINT('Ctrl Pts',(-0.0308180903310451,0.240897960470908,
1.53351007774908));
#23868=CARTESIAN_POINT('Ctrl Pts',(-0.219105973246366,0.104757609325286,
1.54462386680588));
#23869=CARTESIAN_POINT('Ctrl Pts',(-0.206843620635952,-0.127268531807556,
1.55573765586268));
#23870=CARTESIAN_POINT('Ctrl Pts',(-0.00525505851706014,-0.242804414954791,
1.56685144491949));
#23871=CARTESIAN_POINT('Ctrl Pts',(0.173370196153793,-0.15045712725832,
1.57646973564985));
#23872=CARTESIAN_POINT('Ctrl Pts',(0.20500411501816,-0.0407723333551383,
1.58238343002794));
#23873=CARTESIAN_POINT('Ctrl Pts',(0.2051889883028,0.000102640746213654,
1.58459252805377));
#23874=CARTESIAN_POINT('Origin',(0.,0.,0.645407471946233));
#23875=CARTESIAN_POINT('',(0.205812292792875,8.2771271442428E-7,1.44459252805377));
#23876=CARTESIAN_POINT('',(0.20514810115636,4.68968264668604E-5,1.45040747194623));
#23877=CARTESIAN_POINT('',(0.205475,1.17874941047504E-14,0.645407471946233));
#23878=CARTESIAN_POINT('Ctrl Pts',(0.20514810115636,4.68968264668648E-5,
1.45040747194623));
#23879=CARTESIAN_POINT('Ctrl Pts',(0.205212209277079,0.0314508805486537,
1.45210386154759));
#23880=CARTESIAN_POINT('Ctrl Pts',(0.183673234943095,0.131351887215635,
1.45750484750122));
#23881=CARTESIAN_POINT('Ctrl Pts',(0.028210615278035,0.241217190661839,
1.46661042980711));
#23882=CARTESIAN_POINT('Ctrl Pts',(-0.187360277963068,0.154524103926572,
1.47772421886392));
#23883=CARTESIAN_POINT('Ctrl Pts',(-0.23143818564818,-0.0736066521476796,
1.48883800792072));
#23884=CARTESIAN_POINT('Ctrl Pts',(-0.0636780941176189,-0.234364395962394,
1.49995179697753));
#23885=CARTESIAN_POINT('Ctrl Pts',(0.15035425339619,-0.183462731047792,
1.51047495165269));
#23886=CARTESIAN_POINT('Ctrl Pts',(0.205127050891722,-0.0571438705105598,
1.5172935099756));
#23887=CARTESIAN_POINT('Ctrl Pts',(0.205625119184624,0.000163390229490371,
1.52040747194623));
#23888=CARTESIAN_POINT('Ctrl Pts',(0.205812290976358,8.27708256686491E-7,
1.44459252805377));
#23889=CARTESIAN_POINT('Ctrl Pts',(0.205812293621698,4.5117938930396E-5,
1.44459494046739));
#23890=CARTESIAN_POINT('Ctrl Pts',(0.205792223959932,0.0681032095145843,
1.44830194923329));
#23891=CARTESIAN_POINT('Ctrl Pts',(0.13158183823911,0.204126920402922,1.45571355435144));
#23892=CARTESIAN_POINT('Ctrl Pts',(-0.10013585656473,0.221256389923926,
1.46682734340825));
#23893=CARTESIAN_POINT('Ctrl Pts',(-0.240198066802314,0.0358673761285168,
1.47794113246505));
#23894=CARTESIAN_POINT('Ctrl Pts',(-0.160404261381875,-0.182351453033287,
1.48905492152186));
#23895=CARTESIAN_POINT('Ctrl Pts',(0.0662093815164626,-0.233661930697804,
1.50016871057866));
#23896=CARTESIAN_POINT('Ctrl Pts',(0.193364787149743,-0.109147888339539,
1.5086812460893));
#23897=CARTESIAN_POINT('Ctrl Pts',(0.20551319671518,-0.0205523937625982,
1.51348918524767));
#23898=CARTESIAN_POINT('Ctrl Pts',(0.205346259354759,-0.000176524568076758,
1.51459252805377));
#23899=CARTESIAN_POINT('Origin',(0.,0.,0.645407471946233));
#23900=CARTESIAN_POINT('',(0.205343844683429,0.000176004178461642,1.37459252805377));
#23901=CARTESIAN_POINT('',(0.205453133831238,-0.000187888241826064,1.38040747194623));
#23902=CARTESIAN_POINT('',(0.205475,1.17874941047504E-14,0.645407471946233));
#23903=CARTESIAN_POINT('Ctrl Pts',(0.205453133831238,-0.000187888241826079,
1.38040747194623));
#23904=CARTESIAN_POINT('Ctrl Pts',(0.204982640394683,0.0514920396676331,
1.38320961676732));
#23905=CARTESIAN_POINT('Ctrl Pts',(0.159017805479884,0.172241441932577,
1.38971635794067));
#23906=CARTESIAN_POINT('Ctrl Pts',(-0.0437982449057285,0.238879228826581,
1.39992769546629));
#23907=CARTESIAN_POINT('Ctrl Pts',(-0.224449621610114,0.0927574233548304,
1.41104148452309));
#23908=CARTESIAN_POINT('Ctrl Pts',(-0.199659714256911,-0.13826630374757,
1.42215527357989));
#23909=CARTESIAN_POINT('Ctrl Pts',(0.00788099391586731,-0.242733314804761,
1.4332690626367));
#23910=CARTESIAN_POINT('Ctrl Pts',(0.177630548818419,-0.142990752308629,
1.44268646209214));
#23911=CARTESIAN_POINT('Ctrl Pts',(0.205072209179237,-0.037129523063069,
1.44839926519532));
#23912=CARTESIAN_POINT('Ctrl Pts',(0.20514810115636,4.68968264668648E-5,
1.45040747194623));
#23913=CARTESIAN_POINT('Ctrl Pts',(0.205343844683429,0.000176004178461609,
1.37459252805377));
#23914=CARTESIAN_POINT('Ctrl Pts',(0.2055108740339,0.0206415845782027,1.37570069568712));
#23915=CARTESIAN_POINT('Ctrl Pts',(0.193294976926761,0.109328542053589,
1.38051345967274));
#23916=CARTESIAN_POINT('Ctrl Pts',(0.0659057470887793,0.233747753644337,
1.38903082001062));
#23917=CARTESIAN_POINT('Ctrl Pts',(-0.160641042350602,0.182142898149225,
1.40014460906743));
#23918=CARTESIAN_POINT('Ctrl Pts',(-0.240151263944613,-0.0361794176709605,
1.41125839812423));
#23919=CARTESIAN_POINT('Ctrl Pts',(-0.0998483101275995,-0.221386302178844,
1.42237218718103));
#23920=CARTESIAN_POINT('Ctrl Pts',(0.131796641356581,-0.203959577192589,
1.43348356382421));
#23921=CARTESIAN_POINT('Ctrl Pts',(0.205808231334455,-0.0679686858761153,
1.44089034411512));
#23922=CARTESIAN_POINT('Ctrl Pts',(0.205812290976358,8.27708256686491E-7,
1.44459252805377));
#23923=CARTESIAN_POINT('Origin',(0.,0.,0.645407471946233));
#23924=CARTESIAN_POINT('',(0.205190393281102,-0.000103909026722956,1.30459252805377));
#23925=CARTESIAN_POINT('',(0.205784930460293,6.78762012092915E-5,1.31040747194623));
#23926=CARTESIAN_POINT('',(0.205475,1.17874941047504E-14,0.645407471946233));
#23927=CARTESIAN_POINT('Ctrl Pts',(0.205784930460293,6.78762012092937E-5,
1.31040747194623));
#23928=CARTESIAN_POINT('Ctrl Pts',(0.205801002271222,0.00380171834571078,
1.31061077563477));
#23929=CARTESIAN_POINT('Ctrl Pts',(0.204016743590097,0.0755578983061786,
1.31451867567558));
#23930=CARTESIAN_POINT('Ctrl Pts',(0.120352309668968,0.210942868533614,
1.32213117206866));
#23931=CARTESIAN_POINT('Ctrl Pts',(-0.111952589707427,0.215518421220722,
1.33324496112546));
#23932=CARTESIAN_POINT('Ctrl Pts',(-0.241786014095534,0.0228275188203595,
1.34435875018226));
#23933=CARTESIAN_POINT('Ctrl Pts',(-0.150309957742793,-0.190757670439842,
1.35547253923907));
#23934=CARTESIAN_POINT('Ctrl Pts',(0.0787465075641072,-0.229740200603712,
1.36658632829588));
#23935=CARTESIAN_POINT('Ctrl Pts',(0.196145957186436,-0.101629499882189,
1.37489797253159));
#23936=CARTESIAN_POINT('Ctrl Pts',(0.205604659733481,-0.0168317924834936,
1.37950502041505));
#23937=CARTESIAN_POINT('Ctrl Pts',(0.205453133831238,-0.000187888241826079,
1.38040747194623));
#23938=CARTESIAN_POINT('Ctrl Pts',(0.205190393281102,-0.000103909026722949,
1.30459252805377));
#23939=CARTESIAN_POINT('Ctrl Pts',(0.205002798510851,0.0408596785255145,
1.30680645090684));
#23940=CARTESIAN_POINT('Ctrl Pts',(0.173264151191812,0.15063609956695,1.31272497011219));
#23941=CARTESIAN_POINT('Ctrl Pts',(-0.00557045627447471,0.242797343170749,
1.3223480856698));
#23942=CARTESIAN_POINT('Ctrl Pts',(-0.207008825709279,0.126999708315969,
1.3334618747266));
#23943=CARTESIAN_POINT('Ctrl Pts',(-0.218969669332857,-0.105042199835232,
1.3445756637834));
#23944=CARTESIAN_POINT('Ctrl Pts',(-0.0305050913306782,-0.240937791217362,
1.35568945284021));
#23945=CARTESIAN_POINT('Ctrl Pts',(0.164305043004325,-0.164739584440547,
1.36569507426366));
#23946=CARTESIAN_POINT('Ctrl Pts',(0.204952496128017,-0.0477747021046654,
1.37199609933485));
#23947=CARTESIAN_POINT('Ctrl Pts',(0.205343844683429,0.000176004178461609,
1.37459252805377));
#23948=CARTESIAN_POINT('Origin',(0.,0.,0.645407471946233));
#23949=CARTESIAN_POINT('',(0.205723053630104,-0.00012021653370823,1.23459252805377));
#23950=CARTESIAN_POINT('',(0.2052527421894,0.000145096082381024,1.24040747194623));
#23951=CARTESIAN_POINT('',(0.205475,1.17874941047504E-14,0.645407471946233));
#23952=CARTESIAN_POINT('Ctrl Pts',(0.2052527421894,0.000145096082381054,
1.24040747194623));
#23953=CARTESIAN_POINT('Ctrl Pts',(0.205410551512377,0.0243477880181972,
1.2417165308545));
#23954=CARTESIAN_POINT('Ctrl Pts',(0.19025975845005,0.116852155262949,1.24673018611503));
#23955=CARTESIAN_POINT('Ctrl Pts',(0.053170711887795,0.236969296798376,
1.25544843772783));
#23956=CARTESIAN_POINT('Ctrl Pts',(-0.170254416296827,0.17319066360285,
1.26656222678464));
#23957=CARTESIAN_POINT('Ctrl Pts',(-0.237843746428552,-0.0491113481040567,
1.27767601584144));
#23958=CARTESIAN_POINT('Ctrl Pts',(-0.0877319981226961,-0.226461185930791,
1.28878980489824));
#23959=CARTESIAN_POINT('Ctrl Pts',(0.138466900336863,-0.197076087766382,
1.29970029026651));
#23960=CARTESIAN_POINT('Ctrl Pts',(0.205508142006035,-0.0642362896597867,
1.3069061792825));
#23961=CARTESIAN_POINT('Ctrl Pts',(0.205784930460293,6.78762012092937E-5,
1.31040747194623));
#23962=CARTESIAN_POINT('Ctrl Pts',(0.205723053630104,-0.000120216533708221,
1.23459252805377));
#23963=CARTESIAN_POINT('Ctrl Pts',(0.205298918797858,0.0608969853087639,
1.23791220612657));
#23964=CARTESIAN_POINT('Ctrl Pts',(0.144198668474879,0.190744063350028,
1.24493648055164));
#23965=CARTESIAN_POINT('Ctrl Pts',(-0.0765564251386213,0.230479269358191,
1.25566535132897));
#23966=CARTESIAN_POINT('Ctrl Pts',(-0.23515855594305,0.0606797610465845,
1.26677914038578));
#23967=CARTESIAN_POINT('Ctrl Pts',(-0.178517393613401,-0.164660620706261,
1.27789292944258));
#23968=CARTESIAN_POINT('Ctrl Pts',(0.0415227636155418,-0.239285268948212,
1.28900671849938));
#23969=CARTESIAN_POINT('Ctrl Pts',(0.187294592944535,-0.123653783093607,
1.29790658470311));
#23970=CARTESIAN_POINT('Ctrl Pts',(0.205316704165066,-0.0276854186132918,
1.30310185455457));
#23971=CARTESIAN_POINT('Ctrl Pts',(0.205190393281102,-0.000103909026722949,
1.30459252805377));
#23972=CARTESIAN_POINT('Origin',(0.,0.,0.645407471946233));
#23973=CARTESIAN_POINT('',(0.205554604385647,0.000179910838621594,1.16459252805377));
#23974=CARTESIAN_POINT('',(0.205260574591088,-0.000148793951100861,1.17040747194623));
#23975=CARTESIAN_POINT('',(0.205475,1.17874941047504E-14,0.645407471946233));
#23976=CARTESIAN_POINT('Ctrl Pts',(0.205260574591088,-0.000148793951100864,
1.17040747194623));
#23977=CARTESIAN_POINT('Ctrl Pts',(0.204961311968991,0.044493502374408,
1.17282228607422));
#23978=CARTESIAN_POINT('Ctrl Pts',(0.168697767785137,0.158064764697474,
1.17894169655448));
#23979=CARTESIAN_POINT('Ctrl Pts',(-0.0186902364010947,0.242140965743205,
1.18876570338701));
#23980=CARTESIAN_POINT('Ctrl Pts',(-0.213572804428157,0.115621059658089,
1.19987949244381));
#23981=CARTESIAN_POINT('Ctrl Pts',(-0.212969762481792,-0.116728113564033,
1.21099328150062));
#23982=CARTESIAN_POINT('Ctrl Pts',(-0.0174330816944656,-0.242234720654174,
1.22210707055742));
#23983=CARTESIAN_POINT('Ctrl Pts',(0.169149144270981,-0.157353841391122,
1.23191180070596));
#23984=CARTESIAN_POINT('Ctrl Pts',(0.204963955993594,-0.0441450839941835,
1.23801193450223));
#23985=CARTESIAN_POINT('Ctrl Pts',(0.2052527421894,0.000145096082381054,
1.24040747194623));
#23986=CARTESIAN_POINT('Ctrl Pts',(0.205554604385647,0.00017991083862162,
1.16459252805377));
#23987=CARTESIAN_POINT('Ctrl Pts',(0.205676289601756,0.0134574818611262,
1.16531336499402));
#23988=CARTESIAN_POINT('Ctrl Pts',(0.198454332603713,0.094840644563722,
1.16973879828655));
#23989=CARTESIAN_POINT('Ctrl Pts',(0.0898833437085198,0.225615966539919,
1.17786882793134));
#23990=CARTESIAN_POINT('Ctrl Pts',(-0.140804956527845,0.197877598659039,
1.18898261698814));
#23991=CARTESIAN_POINT('Ctrl Pts',(-0.242612883217311,-0.0109803793588139,
1.20009640604495));
#23992=CARTESIAN_POINT('Ctrl Pts',(-0.12235448648082,-0.2097878916237,1.21121019510175));
#23993=CARTESIAN_POINT('Ctrl Pts',(0.109896359325859,-0.21657416752884,
1.22232398415856));
#23994=CARTESIAN_POINT('Ctrl Pts',(0.202230669468777,-0.082312541395209,
1.23011809514256));
#23995=CARTESIAN_POINT('Ctrl Pts',(0.20577223226921,-0.00719519062340044,
1.2342076097743));
#23996=CARTESIAN_POINT('Ctrl Pts',(0.205723053630104,-0.000120216533708221,
1.23459252805377));
#23997=CARTESIAN_POINT('Origin',(0.,0.,0.645407471946233));
#23998=CARTESIAN_POINT('',(0.205138522353965,7.81005524626288E-6,1.09459252805377));
#23999=CARTESIAN_POINT('',(0.205789655863746,-6.17368779781373E-5,1.10040747194623));
#24000=CARTESIAN_POINT('',(0.205475,1.17874941047504E-14,0.645407471946233));
#24001=CARTESIAN_POINT('Ctrl Pts',(0.205789655863746,-6.17368779781361E-5,
1.10040747194623));
#24002=CARTESIAN_POINT('Ctrl Pts',(0.205533723504375,0.0645925032691717,
1.10392804129395));
#24003=CARTESIAN_POINT('Ctrl Pts',(0.137841967409279,0.197742342810066,
1.11115320699393));
#24004=CARTESIAN_POINT('Ctrl Pts',(-0.0889063286388705,0.226002736612265,
1.12208296904618));
#24005=CARTESIAN_POINT('Ctrl Pts',(-0.238095468835566,0.0478760895194249,
1.13319675810299));
#24006=CARTESIAN_POINT('Ctrl Pts',(-0.169353126220915,-0.174072085260317,
1.14431054715979));
#24007=CARTESIAN_POINT('Ctrl Pts',(0.0544000534188783,-0.236690106290626,
1.1554243362166));
#24008=CARTESIAN_POINT('Ctrl Pts',(0.190562019135808,-0.116130140045317,
1.16412331114541));
#24009=CARTESIAN_POINT('Ctrl Pts',(0.2054204144752,-0.0239927989965278,
1.16911768972195));
#24010=CARTESIAN_POINT('Ctrl Pts',(0.205260574591088,-0.000148793951100864,
1.17040747194623));
#24011=CARTESIAN_POINT('Ctrl Pts',(0.205138522353965,7.81005524630105E-6,
1.09459252805377));
#24012=CARTESIAN_POINT('Ctrl Pts',(0.205149988139531,0.033826082896543,
1.09641912021375));
#24013=CARTESIAN_POINT('Ctrl Pts',(0.181232693643337,0.1362174972132,1.101950308726));
#24014=CARTESIAN_POINT('Ctrl Pts',(0.019737729131079,0.242057848222183,
1.11118609359052));
#24015=CARTESIAN_POINT('Ctrl Pts',(-0.192661783512051,0.147861479120299,
1.12229988264732));
#24016=CARTESIAN_POINT('Ctrl Pts',(-0.228715780766039,-0.0816741786716276,
1.13341367170413));
#24017=CARTESIAN_POINT('Ctrl Pts',(-0.0554236300753314,-0.236452534483491,
1.14452746076093));
#24018=CARTESIAN_POINT('Ctrl Pts',(0.15406839794226,-0.178801760545413,
1.15492041287748));
#24019=CARTESIAN_POINT('Ctrl Pts',(0.205050912928411,-0.0547799216762583,
1.16160876864176));
#24020=CARTESIAN_POINT('Ctrl Pts',(0.205554604385647,0.00017991083862162,
1.16459252805377));
#24021=CARTESIAN_POINT('Origin',(0.,0.,0.645407471946233));
#24022=CARTESIAN_POINT('',(0.20552593591886,-0.000183965626637278,1.02459252805377));
#24023=CARTESIAN_POINT('',(0.20544247508097,0.000187699708462681,1.03040747194623));
#24024=CARTESIAN_POINT('',(0.205475,1.17874941047504E-14,0.645407471946233));
#24025=CARTESIAN_POINT('Ctrl Pts',(0.20544247508097,0.000187699708462687,
1.03040747194623));
#24026=CARTESIAN_POINT('Ctrl Pts',(0.205596383177594,0.0171893738494543,
1.0313292001614));
#24027=CARTESIAN_POINT('Ctrl Pts',(0.195889593181661,0.102350581389175,
1.03595552472885));
#24028=CARTESIAN_POINT('Ctrl Pts',(0.0775529135379212,0.230145861972334,
1.04428644564855));
#24029=CARTESIAN_POINT('Ctrl Pts',(-0.151298115744515,0.18997487313149,
1.05540023470536));
#24030=CARTESIAN_POINT('Ctrl Pts',(-0.241664263837854,-0.0240822717379046,
1.06651402376216));
#24031=CARTESIAN_POINT('Ctrl Pts',(-0.110832370586897,-0.216096640074974,
1.07762781281897));
#24032=CARTESIAN_POINT('Ctrl Pts',(0.121445648389767,-0.210315303100593,
1.08874160187577));
#24033=CARTESIAN_POINT('Ctrl Pts',(0.204196124007957,-0.074841794914668,
1.09633482158486));
#24034=CARTESIAN_POINT('Ctrl Pts',(0.205803033945758,-0.00344133971228389,
1.10022344494168));
#24035=CARTESIAN_POINT('Ctrl Pts',(0.205789655863746,-6.17368779781361E-5,
1.10040747194623));
#24036=CARTESIAN_POINT('Ctrl Pts',(0.20552593591886,-0.000183965626637285,
1.02459252805377));
#24037=CARTESIAN_POINT('Ctrl Pts',(0.205027284976747,0.0538482597648122,
1.02752487543347));
#24038=CARTESIAN_POINT('Ctrl Pts',(0.155496650182077,0.176951247041673,
1.03416181916545));
#24039=CARTESIAN_POINT('Ctrl Pts',(-0.0521449271278155,0.237197146991165,
1.04450335924969));
#24040=CARTESIAN_POINT('Ctrl Pts',(-0.227563185653378,0.0848326375129703,
1.0556171483065));
#24041=CARTESIAN_POINT('Ctrl Pts',(-0.194690279246867,-0.145180146557101,
1.0667309373633));
#24042=CARTESIAN_POINT('Ctrl Pts',(0.0163848475034698,-0.242307896337387,
1.0778447264201));
#24043=CARTESIAN_POINT('Ctrl Pts',(0.180236614284166,-0.138136714556845,
1.08713192331693));
#24044=CARTESIAN_POINT('Ctrl Pts',(0.205126733847568,-0.0347623261378718,
1.09271452386148));
#24045=CARTESIAN_POINT('Ctrl Pts',(0.205138522353965,7.81005524630105E-6,
1.09459252805377));
#24046=CARTESIAN_POINT('Origin',(0.,0.,0.645407471946233));
#24047=CARTESIAN_POINT('',(0.205743448352251,0.000106566711118361,0.954592528053768));
#24048=CARTESIAN_POINT('',(0.205150677731907,-5.25566492129599E-5,0.960407471946232));
#24049=CARTESIAN_POINT('',(0.205475,1.17874941047504E-14,0.645407471946233));
#24050=CARTESIAN_POINT('Ctrl Pts',(0.205150677731907,-5.25566492129668E-5,
0.960407471946232));
#24051=CARTESIAN_POINT('Ctrl Pts',(0.205064756039612,0.0374795435537448,
0.962434955381129));
#24052=CARTESIAN_POINT('Ctrl Pts',(0.177234439623409,0.143708517228788,
0.968167035168295));
#24053=CARTESIAN_POINT('Ctrl Pts',(0.00662091032790181,0.242770948244842,
0.977603711307729));
#24054=CARTESIAN_POINT('Ctrl Pts',(-0.200374735874429,0.13722805194188,
0.988717500364533));
#24055=CARTESIAN_POINT('Ctrl Pts',(-0.223965113394512,-0.0939212459185429,
0.999831289421336));
#24056=CARTESIAN_POINT('Ctrl Pts',(-0.0425576829655005,-0.239103357370329,
1.01094507847814));
#24057=CARTESIAN_POINT('Ctrl Pts',(0.159527519870246,-0.171541476398135,
1.02113713931977));
#24058=CARTESIAN_POINT('Ctrl Pts',(0.204977798041595,-0.0511435023372491,
1.02762460380914));
#24059=CARTESIAN_POINT('Ctrl Pts',(0.20544247508097,0.000187699708462687,
1.03040747194623));
#24060=CARTESIAN_POINT('Ctrl Pts',(0.205743448352251,0.000106566711118368,
0.954592528053768));
#24061=CARTESIAN_POINT('Ctrl Pts',(0.205782131072789,0.00623496563411944,
0.954926034300931));
#24062=CARTESIAN_POINT('Ctrl Pts',(0.202754080859383,0.0803990246761448,
0.958964136900363));
#24063=CARTESIAN_POINT('Ctrl Pts',(0.112884009708659,0.215032004451281,
0.966706835852063));
#24064=CARTESIAN_POINT('Ctrl Pts',(-0.119438498942156,0.211461649464463,
0.977820624908867));
#24065=CARTESIAN_POINT('Ctrl Pts',(-0.242437629122786,0.0143379927471741,
0.988934413965671));
#24066=CARTESIAN_POINT('Ctrl Pts',(-0.143530830111561,-0.195909362177039,
1.00004820302247));
#24067=CARTESIAN_POINT('Ctrl Pts',(0.086751356142284,-0.226838671363958,
1.01116199207928));
#24068=CARTESIAN_POINT('Ctrl Pts',(0.19782031948766,-0.0967615068704032,
1.01934343375638));
#24069=CARTESIAN_POINT('Ctrl Pts',(0.205657258244577,-0.0144136339232786,
1.02382027908121));
#24070=CARTESIAN_POINT('Ctrl Pts',(0.20552593591886,-0.000183965626637285,
1.02459252805377));
#24071=CARTESIAN_POINT('Origin',(0.,0.,0.645407471946233));
#24072=CARTESIAN_POINT('',(0.205205445749305,0.000116004416325019,0.884592528053768));
#24073=CARTESIAN_POINT('',(0.205635165348036,-0.000160487501855341,0.890407471946233));
#24074=CARTESIAN_POINT('',(0.205475,1.17874941047504E-14,0.645407471946233));
#24075=CARTESIAN_POINT('Ctrl Pts',(0.205635165348036,-0.000160487501855345,
0.890407471946233));
#24076=CARTESIAN_POINT('Ctrl Pts',(0.20514041316225,0.0574941994909011,
0.893540710600855));
#24077=CARTESIAN_POINT('Ctrl Pts',(0.149792439928844,0.184149942781777,
0.900378545607745));
#24078=CARTESIAN_POINT('Ctrl Pts',(-0.0648937601106981,0.234030453531351,
0.910920976966904));
#24079=CARTESIAN_POINT('Ctrl Pts',(-0.231817150854124,0.0724044416546206,
0.922034766023707));
#24080=CARTESIAN_POINT('Ctrl Pts',(-0.186555648217912,-0.155494636948999,
0.933148555080512));
#24081=CARTESIAN_POINT('Ctrl Pts',(0.029462341223335,-0.241067470577576,
0.944262344137316));
#24082=CARTESIAN_POINT('Ctrl Pts',(0.184024675492061,-0.130631009068519,
0.953348649759223));
#24083=CARTESIAN_POINT('Ctrl Pts',(0.205221751249722,-0.031098714158076,
0.958730359028861));
#24084=CARTESIAN_POINT('Ctrl Pts',(0.205150677731907,-5.25566492129668E-5,
0.960407471946232));
#24085=CARTESIAN_POINT('Ctrl Pts',(0.205205445749305,0.000116004416325009,
0.884592528053768));
#24086=CARTESIAN_POINT('Ctrl Pts',(0.205343275267841,0.0267417723340512,
0.886031789520656));
#24087=CARTESIAN_POINT('Ctrl Pts',(0.188156931475396,0.121730614284078,
0.891175647339813));
#24088=CARTESIAN_POINT('Ctrl Pts',(0.0448304764247631,0.238686010114805,
0.900024101511237));
#24089=CARTESIAN_POINT('Ctrl Pts',(-0.176220286722883,0.167116974718297,
0.911137890568042));
#24090=CARTESIAN_POINT('Ctrl Pts',(-0.235976306336092,-0.0574188764093974,
0.922251679624847));
#24091=CARTESIAN_POINT('Ctrl Pts',(-0.0797396575425977,-0.229397140881452,
0.933365468681649));
#24092=CARTESIAN_POINT('Ctrl Pts',(0.142604551604849,-0.192546391773689,
0.944145751491291));
#24093=CARTESIAN_POINT('Ctrl Pts',(0.205352442373934,-0.0618394542260256,
0.951221437948663));
#24094=CARTESIAN_POINT('Ctrl Pts',(0.205743448352251,0.000106566711118368,
0.954592528053768));
#24095=CARTESIAN_POINT('Origin',(0.,0.,0.645407471946233));
#24096=CARTESIAN_POINT('',(0.205269394176581,-0.000252214316689744,0.814592528053768));
#24097=CARTESIAN_POINT('',(0.205654271051376,0.000148184871923512,0.820407471946232));
#24098=CARTESIAN_POINT('',(0.205475,1.17874941047504E-14,0.645407471946233));
#24099=CARTESIAN_POINT('',(0.0530170217188605,-0.198517432567172,0.8));
#24100=CARTESIAN_POINT('Ctrl Pts',(0.0530170217188587,-0.198517432567173,
0.8));
#24101=CARTESIAN_POINT('Ctrl Pts',(0.119028790974553,-0.18088801151799,
0.803704596352268));
#24102=CARTESIAN_POINT('Ctrl Pts',(0.192500600447326,-0.111310459456284,
0.80856877237019));
#24103=CARTESIAN_POINT('Ctrl Pts',(0.205431969941924,-0.0216798251681207,
0.813432948388113));
#24104=CARTESIAN_POINT('Ctrl Pts',(0.205269394176581,-0.000252214316689755,
0.814592528053767));
#24105=CARTESIAN_POINT('',(-0.0531250535940746,-0.19887604744663,0.8));
#24106=CARTESIAN_POINT('Origin',(0.,0.,0.8));
#24107=CARTESIAN_POINT('Ctrl Pts',(-0.053125080564462,-0.198876136975597,
0.8));
#24108=CARTESIAN_POINT('Ctrl Pts',(0.0113386551506616,-0.21601151578625,
0.803632291818556));
#24109=CARTESIAN_POINT('Ctrl Pts',(0.149296237339328,-0.184051126983177,
0.810434782467299));
#24110=CARTESIAN_POINT('Ctrl Pts',(0.205166930984713,-0.0581571994559903,
0.817237273116043));
#24111=CARTESIAN_POINT('Ctrl Pts',(0.205654271051376,0.000148184871923506,
0.820407471946232));
#24112=CARTESIAN_POINT('Origin',(0.,0.,3.1));
#24113=CARTESIAN_POINT('',(-0.126245549239308,1.45328325776573E-5,2.71934196736194));
#24114=CARTESIAN_POINT('',(-0.126374981062586,-0.000161346902988299,2.70565803263806));
#24115=CARTESIAN_POINT('',(-0.12645,1.54856587752183E-17,3.1));
#24116=CARTESIAN_POINT('',(-0.0958116152722464,0.0825211298936403,2.7));
#24117=CARTESIAN_POINT('Ctrl Pts',(-0.126374981062586,-0.000161346902988299,
2.70565803263806));
#24118=CARTESIAN_POINT('Ctrl Pts',(-0.126107573254536,0.0297492098111863,
2.70377202175871));
#24119=CARTESIAN_POINT('Ctrl Pts',(-0.115369380269341,0.0598134784363487,
2.70188601087935));
#24120=CARTESIAN_POINT('Ctrl Pts',(-0.0958116152722464,0.0825211298936403,
2.7));
#24121=CARTESIAN_POINT('',(-0.12645,1.54856587752183E-17,2.7));
#24122=CARTESIAN_POINT('Origin',(0.,0.,2.7));
#24123=CARTESIAN_POINT('',(-0.12645,-1.54856587752183E-17,2.6));
#24124=CARTESIAN_POINT('',(-0.12645,1.54856587752183E-17,3.1));
#24125=CARTESIAN_POINT('Origin',(0.,0.,2.6));
#24126=CARTESIAN_POINT('',(0.095991445127536,0.0826500758460347,2.7));
#24127=CARTESIAN_POINT('Origin',(0.,0.,2.7));
#24128=CARTESIAN_POINT('Ctrl Pts',(0.0959918005672157,0.0826503307119909,
2.7));
#24129=CARTESIAN_POINT('Ctrl Pts',(0.0697118516972522,0.11301027640157,
2.70253749952686));
#24130=CARTESIAN_POINT('Ctrl Pts',(0.0277082938822606,0.129939474688335,
2.70507499905372));
#24131=CARTESIAN_POINT('Ctrl Pts',(-0.0122513412479025,0.126048724837631,
2.70761249858058));
#24132=CARTESIAN_POINT('Ctrl Pts',(-0.0537056163258554,0.122012446376998,
2.71024491008919));
#24133=CARTESIAN_POINT('Ctrl Pts',(-0.092960208469122,0.0955696038330054,
2.7128773215978));
#24134=CARTESIAN_POINT('Ctrl Pts',(-0.1122448026076,0.0586681233168463,
2.71550973310641));
#24135=CARTESIAN_POINT('Ctrl Pts',(-0.121602899042457,0.0407612070094829,
2.71678714452492));
#24136=CARTESIAN_POINT('Ctrl Pts',(-0.126258460357629,0.0203914906379236,
2.71806455594343));
#24137=CARTESIAN_POINT('Ctrl Pts',(-0.126245549239308,1.45328325776573E-5,
2.71934196736194));
#24138=CARTESIAN_POINT('Origin',(0.,0.,3.1));
#24139=CARTESIAN_POINT('',(-0.126511755116174,-0.000105182036976022,2.76934196736194));
#24140=CARTESIAN_POINT('',(-0.12664039552615,3.66938896950461E-5,2.75565803263806));
#24141=CARTESIAN_POINT('',(-0.12645,1.54856587752183E-17,3.1));
#24142=CARTESIAN_POINT('Ctrl Pts',(-0.12664039552615,3.66938896950461E-5,
2.75565803263806));
#24143=CARTESIAN_POINT('Ctrl Pts',(-0.126647890342436,0.00202721792373194,
2.75553223565232));
#24144=CARTESIAN_POINT('Ctrl Pts',(-0.126604975133189,0.00401740611511355,
2.75540643866659));
#24145=CARTESIAN_POINT('Ctrl Pts',(-0.126510633504476,0.00600514734308786,
2.75528064168085));
#24146=CARTESIAN_POINT('Ctrl Pts',(-0.124536452742414,0.0476003640650105,
2.75264823017224));
#24147=CARTESIAN_POINT('Ctrl Pts',(-0.10004305012127,0.0881240748873803,
2.75001581866363));
#24148=CARTESIAN_POINT('Ctrl Pts',(-0.064133889095878,0.109212690295602,
2.74738340715501));
#24149=CARTESIAN_POINT('Ctrl Pts',(-0.0282247280704852,0.130301305703824,
2.7447509956464));
#24150=CARTESIAN_POINT('Ctrl Pts',(0.0191001913591554,0.131954825697897,
2.74211858413779));
#24151=CARTESIAN_POINT('Ctrl Pts',(0.0563882647159258,0.113411365221879,
2.73948617262918));
#24152=CARTESIAN_POINT('Ctrl Pts',(0.0936763380726957,0.0948679047458623,
2.73685376112057));
#24153=CARTESIAN_POINT('Ctrl Pts',(0.120927565356595,0.0561274637997562,
2.73422134961196));
#24154=CARTESIAN_POINT('Ctrl Pts',(0.125787645771127,0.0147753877020813,
2.73158893810334));
#24155=CARTESIAN_POINT('Ctrl Pts',(0.13064772618566,-0.0265766883955932,
2.72895652659473));
#24156=CARTESIAN_POINT('Ctrl Pts',(0.113116659730824,-0.0705403996448371,
2.72632411508612));
#24157=CARTESIAN_POINT('Ctrl Pts',(0.0811433928446468,-0.0972323182667412,
2.72369170357751));
#24158=CARTESIAN_POINT('Ctrl Pts',(0.0491701259584694,-0.123924236888645,
2.7210592920689));
#24159=CARTESIAN_POINT('Ctrl Pts',(0.00275465864095025,-0.133344362883211,
2.71842688056028));
#24160=CARTESIAN_POINT('Ctrl Pts',(-0.0370665720412133,-0.121131225367919,
2.71579446905167));
#24161=CARTESIAN_POINT('Ctrl Pts',(-0.0768878027233769,-0.108918087852628,
2.71316205754306));
#24162=CARTESIAN_POINT('Ctrl Pts',(-0.110114796770184,-0.0750716868274789,
2.71052964603445));
#24163=CARTESIAN_POINT('Ctrl Pts',(-0.121670218183899,-0.0351354691109218,
2.70789723452584));
#24164=CARTESIAN_POINT('Ctrl Pts',(-0.124946671651124,-0.023811852747613,
2.70715083389658));
#24165=CARTESIAN_POINT('Ctrl Pts',(-0.126480809379052,-0.0119986372375087,
2.70640443326732));
#24166=CARTESIAN_POINT('Ctrl Pts',(-0.126374981062586,-0.000161346902988299,
2.70565803263806));
#24167=CARTESIAN_POINT('Ctrl Pts',(-0.126245549239308,1.45328325776573E-5,
2.71934196736194));
#24168=CARTESIAN_POINT('Ctrl Pts',(-0.126231853912779,-0.0216001006849982,
2.72069696745204));
#24169=CARTESIAN_POINT('Ctrl Pts',(-0.120965346567412,-0.0432228820262939,
2.72205196754215));
#24170=CARTESIAN_POINT('Ctrl Pts',(-0.110486681315658,-0.0619230805928583,
2.72340696763225));
#24171=CARTESIAN_POINT('Ctrl Pts',(-0.0901293697515468,-0.0982526854980795,
2.72603937914086));
#24172=CARTESIAN_POINT('Ctrl Pts',(-0.0501001504896328,-0.123551776820195,
2.72867179064947));
#24173=CARTESIAN_POINT('Ctrl Pts',(-0.00855140384117574,-0.126362344661561,
2.73130420215808));
#24174=CARTESIAN_POINT('Ctrl Pts',(0.0329973428072813,-0.129172912502927,
2.7339366136667));
#24175=CARTESIAN_POINT('Ctrl Pts',(0.076065616842282,-0.109494956863544,
2.73656902517531));
#24176=CARTESIAN_POINT('Ctrl Pts',(0.10113334277539,-0.0762433600374486,
2.73920143668392));
#24177=CARTESIAN_POINT('Ctrl Pts',(0.126201068708497,-0.0429917632113539,
2.74183384819253));
#24178=CARTESIAN_POINT('Ctrl Pts',(0.133268246539712,0.00383347480145232,
2.74446625970114));
#24179=CARTESIAN_POINT('Ctrl Pts',(0.119129452671912,0.0430029706396828,
2.74709867120975));
#24180=CARTESIAN_POINT('Ctrl Pts',(0.104990658804112,0.0821724664779139,
2.74973108271837));
#24181=CARTESIAN_POINT('Ctrl Pts',(0.0696458932372969,0.113686220141568,
2.75236349422698));
#24182=CARTESIAN_POINT('Ctrl Pts',(0.0291183743037611,0.123260050517998,
2.75499590573559));
#24183=CARTESIAN_POINT('Ctrl Pts',(-0.0114091446297752,0.132833880894428,
2.7576283172442));
#24184=CARTESIAN_POINT('Ctrl Pts',(-0.0571194169300318,0.120467787983633,
2.76026072875281));
#24185=CARTESIAN_POINT('Ctrl Pts',(-0.0872917850925406,0.0917667415677358,
2.76289314026143));
#24186=CARTESIAN_POINT('Ctrl Pts',(-0.111930332277198,0.0683296655464438,
2.76504274929493));
#24187=CARTESIAN_POINT('Ctrl Pts',(-0.126207827945274,0.0340000461494869,
2.76719235832844));
#24188=CARTESIAN_POINT('Ctrl Pts',(-0.126511755116174,-0.000105182036976022,
2.76934196736194));
#24189=CARTESIAN_POINT('Origin',(0.,0.,3.1));
#24190=CARTESIAN_POINT('',(-0.126553655479795,9.34644642624216E-5,2.81934196736194));
#24191=CARTESIAN_POINT('',(-0.126295222915983,7.47437243418914E-5,2.80565803263806));
#24192=CARTESIAN_POINT('',(-0.12645,1.54856587752183E-17,3.1));
#24193=CARTESIAN_POINT('Ctrl Pts',(-0.126295222915983,7.47437243418914E-5,
2.80565803263806));
#24194=CARTESIAN_POINT('Ctrl Pts',(-0.126381902901803,0.0159778826374278,
2.80466003803733));
#24195=CARTESIAN_POINT('Ctrl Pts',(-0.12359488800886,0.0318517555514631,
2.8036620434366));
#24196=CARTESIAN_POINT('Ctrl Pts',(-0.117794192788123,0.0465350551086,2.80266404883586));
#24197=CARTESIAN_POINT('Ctrl Pts',(-0.102493692318657,0.0852652112740412,
2.80003163732725));
#24198=CARTESIAN_POINT('Ctrl Pts',(-0.0662256093040858,0.115711992156929,
2.79739922581864));
#24199=CARTESIAN_POINT('Ctrl Pts',(-0.0254308011719313,0.124073552736451,
2.79476681431003));
#24200=CARTESIAN_POINT('Ctrl Pts',(0.0153640069602226,0.132435113315973,
2.79213440280142));
#24201=CARTESIAN_POINT('Ctrl Pts',(0.0606855402099605,0.11871145359213,
2.78950199129281));
#24202=CARTESIAN_POINT('Ctrl Pts',(0.089988893871543,0.0891234665506248,
2.78686957978419));
#24203=CARTESIAN_POINT('Ctrl Pts',(0.119292247533126,0.0595354795091193,
2.78423716827558));
#24204=CARTESIAN_POINT('Ctrl Pts',(0.132577421606553,0.0140831651499525,
2.78160475676697));
#24205=CARTESIAN_POINT('Ctrl Pts',(0.123822034418855,-0.0266288104888323,
2.77897234525835));
#24206=CARTESIAN_POINT('Ctrl Pts',(0.115066647231157,-0.067340786127616,
2.77633993374974));
#24207=CARTESIAN_POINT('Ctrl Pts',(0.084270698782333,-0.103312423046018,
2.77370752224113));
#24208=CARTESIAN_POINT('Ctrl Pts',(0.045394477490254,-0.11823815061478,
2.77107511073252));
#24209=CARTESIAN_POINT('Ctrl Pts',(0.00651825619817509,-0.133163878183541,
2.76844269922391));
#24210=CARTESIAN_POINT('Ctrl Pts',(-0.0404382379371578,-0.127043696402664,
2.7658102877153));
#24211=CARTESIAN_POINT('Ctrl Pts',(-0.0741890055533361,-0.102650244201489,
2.76317787620668));
#24212=CARTESIAN_POINT('Ctrl Pts',(-0.106326900403039,-0.0794224998497761,
2.76067126168381));
#24213=CARTESIAN_POINT('Ctrl Pts',(-0.126491054782899,-0.0396262314391609,
2.75816464716093));
#24214=CARTESIAN_POINT('Ctrl Pts',(-0.12664039552615,3.66938896950461E-5,
2.75565803263806));
#24215=CARTESIAN_POINT('Ctrl Pts',(-0.126511755116174,-0.000105182036976022,
2.76934196736194));
#24216=CARTESIAN_POINT('Ctrl Pts',(-0.12658001719922,-0.00776522082814862,
2.76982476983705));
#24217=CARTESIAN_POINT('Ctrl Pts',(-0.125943379547996,-0.015413940155386,
2.77030757231215));
#24218=CARTESIAN_POINT('Ctrl Pts',(-0.124560912333973,-0.022925385115547,
2.77079037478726));
#24219=CARTESIAN_POINT('Ctrl Pts',(-0.117023207388135,-0.0638804654619373,
2.77342278629587));
#24220=CARTESIAN_POINT('Ctrl Pts',(-0.0873133334716985,-0.100754626233721,
2.77605519780449));
#24221=CARTESIAN_POINT('Ctrl Pts',(-0.0488993400374831,-0.116832476461904,
2.7786876093131));
#24222=CARTESIAN_POINT('Ctrl Pts',(-0.0104853466032667,-0.132910326690088,
2.78132002082171));
#24223=CARTESIAN_POINT('Ctrl Pts',(0.0366327663487292,-0.128191866374669,
2.78395243233032));
#24224=CARTESIAN_POINT('Ctrl Pts',(0.0710957359713387,-0.104815935790865,
2.78658484383893));
#24225=CARTESIAN_POINT('Ctrl Pts',(0.105558705593947,-0.0814400052070627,
2.78921725534754));
#24226=CARTESIAN_POINT('Ctrl Pts',(0.12736653188717,-0.0394066043548766,
2.79184966685616));
#24227=CARTESIAN_POINT('Ctrl Pts',(0.126633373335447,0.00222985575585417,
2.79448207836477));
#24228=CARTESIAN_POINT('Ctrl Pts',(0.125900214783723,0.0438663158665862,
2.79711448987338));
#24229=CARTESIAN_POINT('Ctrl Pts',(0.102626071387052,0.0851058352358628,
2.79974690138199));
#24230=CARTESIAN_POINT('Ctrl Pts',(0.067361470922124,0.107253965297467,
2.8023793128906));
#24231=CARTESIAN_POINT('Ctrl Pts',(0.032096870457197,0.12940209535907,2.80501172439922));
#24232=CARTESIAN_POINT('Ctrl Pts',(-0.0151581870759861,0.132458836113002,
2.80764413590783));
#24233=CARTESIAN_POINT('Ctrl Pts',(-0.052982302223486,0.115038507268346,
2.81027654741644));
#24234=CARTESIAN_POINT('Ctrl Pts',(-0.0908064173709864,0.0976181784236899,
2.81290895892505));
#24235=CARTESIAN_POINT('Ctrl Pts',(-0.119199590132803,0.059720779980445,
2.81554137043366));
#24236=CARTESIAN_POINT('Ctrl Pts',(-0.12529077505034,0.0185257648347912,
2.81817378194227));
#24237=CARTESIAN_POINT('Ctrl Pts',(-0.126191803554164,0.0124320600196876,
2.81856317708216));
#24238=CARTESIAN_POINT('Ctrl Pts',(-0.126604835154177,0.00626619900254654,
2.81895257222205));
#24239=CARTESIAN_POINT('Ctrl Pts',(-0.126553655479795,9.34644642624216E-5,
2.81934196736194));
#24240=CARTESIAN_POINT('Origin',(0.,0.,3.1));
#24241=CARTESIAN_POINT('',(-0.126249156657861,1.39511119994357E-5,2.86934196736194));
#24242=CARTESIAN_POINT('',(-0.126382098607383,-0.000107526861324363,2.85565803263806));
#24243=CARTESIAN_POINT('',(-0.12645,1.54856587752183E-17,3.1));
#24244=CARTESIAN_POINT('Ctrl Pts',(-0.126382098607383,-0.000107526861324363,
2.85565803263806));
#24245=CARTESIAN_POINT('Ctrl Pts',(-0.126136963881609,0.0296424659657165,
2.85378784042233));
#24246=CARTESIAN_POINT('Ctrl Pts',(-0.115629819550324,0.0595483512746711,
2.8519176482066));
#24247=CARTESIAN_POINT('Ctrl Pts',(-0.0964566207792818,0.0820798491866498,
2.85004745599088));
#24248=CARTESIAN_POINT('Ctrl Pts',(-0.0694691546368386,0.113794329607957,
2.84741504448226));
#24249=CARTESIAN_POINT('Ctrl Pts',(-0.0253122344935349,0.130898446561428,
2.84478263297365));
#24250=CARTESIAN_POINT('Ctrl Pts',(0.0159971616939493,0.125638656106515,
2.84215022146504));
#24251=CARTESIAN_POINT('Ctrl Pts',(0.0573065578814334,0.120378865651602,
2.83951780995643));
#24252=CARTESIAN_POINT('Ctrl Pts',(0.0957684301130981,0.0927551677883048,
2.83688539844782));
#24253=CARTESIAN_POINT('Ctrl Pts',(0.113947449240963,0.0552897840743664,
2.83425298693921));
#24254=CARTESIAN_POINT('Ctrl Pts',(0.132126468368828,0.017824400360428,
2.83162057543059));
#24255=CARTESIAN_POINT('Ctrl Pts',(0.130022634392893,-0.0294826692041511,
2.82898816392198));
#24256=CARTESIAN_POINT('Ctrl Pts',(0.108589645677727,-0.0651864287383833,
2.82635575241337));
#24257=CARTESIAN_POINT('Ctrl Pts',(0.0871566569625619,-0.100890188272616,
2.82372334090476));
#24258=CARTESIAN_POINT('Ctrl Pts',(0.0463945135081664,-0.124990637776501,
2.82109092939615));
#24259=CARTESIAN_POINT('Ctrl Pts',(0.00478129192095443,-0.126562708640517,
2.81845851788753));
#24260=CARTESIAN_POINT('Ctrl Pts',(-0.036831929666257,-0.128134779504533,
2.81582610637892));
#24261=CARTESIAN_POINT('Ctrl Pts',(-0.0792962293862848,-0.10717847172868,
2.81319369487031));
#24262=CARTESIAN_POINT('Ctrl Pts',(-0.103361920284118,-0.0731935521167569,
2.8105612833617));
#24263=CARTESIAN_POINT('Ctrl Pts',(-0.118303874448411,-0.0520929274442991,
2.80892686645382));
#24264=CARTESIAN_POINT('Ctrl Pts',(-0.126153267003299,-0.0259698452031535,
2.80729244954594));
#24265=CARTESIAN_POINT('Ctrl Pts',(-0.126295222915983,7.47437243418914E-5,
2.80565803263806));
#24266=CARTESIAN_POINT('Ctrl Pts',(-0.126553655479795,9.34644642624216E-5,
2.81934196736194));
#24267=CARTESIAN_POINT('Ctrl Pts',(-0.126258847364269,-0.0354630774409815,
2.82158498373066));
#24268=CARTESIAN_POINT('Ctrl Pts',(-0.110561244917173,-0.0712476866904275,
2.82382800009939));
#24269=CARTESIAN_POINT('Ctrl Pts',(-0.0840069629213228,-0.0947829738698732,
2.82607101646811));
#24270=CARTESIAN_POINT('Ctrl Pts',(-0.0528427688015115,-0.122404065580821,
2.82870342797672));
#24271=CARTESIAN_POINT('Ctrl Pts',(-0.00672518348863185,-0.133153617154654,
2.83133583948533));
#24272=CARTESIAN_POINT('Ctrl Pts',(0.0334400182730099,-0.122158697506542,
2.83396825099395));
#24273=CARTESIAN_POINT('Ctrl Pts',(0.0736052200346521,-0.111163777858429,
2.83660066250256));
#24274=CARTESIAN_POINT('Ctrl Pts',(0.107818038245057,-0.0784243869883676,
2.83923307401117));
#24275=CARTESIAN_POINT('Ctrl Pts',(0.120569301232658,-0.0387817708073496,
2.84186548551978));
#24276=CARTESIAN_POINT('Ctrl Pts',(0.13332056422026,0.000860845373668366,
2.84449789702839));
#24277=CARTESIAN_POINT('Ctrl Pts',(0.124610271985061,0.0474066868656423,
2.847130308537));
#24278=CARTESIAN_POINT('Ctrl Pts',(0.0983869277745218,0.0797558433812344,
2.84976272004562));
#24279=CARTESIAN_POINT('Ctrl Pts',(0.0721635835639831,0.112104999896826,
2.85239513155423));
#24280=CARTESIAN_POINT('Ctrl Pts',(0.0284271873781034,0.130257471436035,
2.85502754306284));
#24281=CARTESIAN_POINT('Ctrl Pts',(-0.0129959127687897,0.125984476806968,
2.85765995457145));
#24282=CARTESIAN_POINT('Ctrl Pts',(-0.0544190129156822,0.121711482177902,
2.86029236608007));
#24283=CARTESIAN_POINT('Ctrl Pts',(-0.0935288170235893,0.0950130213805616,
2.86292477758868));
#24284=CARTESIAN_POINT('Ctrl Pts',(-0.11259627866674,0.0579918974128127,
2.86555718909729));
#24285=CARTESIAN_POINT('Ctrl Pts',(-0.121734428756244,0.0402493895934286,
2.86681878185217));
#24286=CARTESIAN_POINT('Ctrl Pts',(-0.126269172738684,0.0201359308353815,
2.86808037460706));
#24287=CARTESIAN_POINT('Ctrl Pts',(-0.126249156657861,1.39511119994357E-5,
2.86934196736194));
#24288=CARTESIAN_POINT('Origin',(0.,0.,3.1));
#24289=CARTESIAN_POINT('',(-0.126504381589359,-0.000106615302056266,2.91934196736194));
#24290=CARTESIAN_POINT('',(-0.126643227510109,3.12951648517141E-5,2.90565803263806));
#24291=CARTESIAN_POINT('',(-0.12645,1.54856587752183E-17,3.1));
#24292=CARTESIAN_POINT('Ctrl Pts',(-0.126643227510109,3.12951648517141E-5,
2.90565803263806));
#24293=CARTESIAN_POINT('Ctrl Pts',(-0.126649060558016,0.00177143581201147,
2.90554805431595));
#24294=CARTESIAN_POINT('Ctrl Pts',(-0.126616264808321,0.00351135171962892,
2.90543807599384));
#24295=CARTESIAN_POINT('Ctrl Pts',(-0.126544152713349,0.00524963660346066,
2.90532809767173));
#24296=CARTESIAN_POINT('Ctrl Pts',(-0.124818097022822,0.0468567555849086,
2.90269568616312));
#24297=CARTESIAN_POINT('Ctrl Pts',(-0.100566951953931,0.0875294297116145,
2.9000632746545));
#24298=CARTESIAN_POINT('Ctrl Pts',(-0.0647841163292417,0.1088301407863,
2.89743086314589));
#24299=CARTESIAN_POINT('Ctrl Pts',(-0.0290012807045523,0.130130851860986,
2.89479845163728));
#24300=CARTESIAN_POINT('Ctrl Pts',(0.0183132454759347,0.13205959988365,
2.89216604012867));
#24301=CARTESIAN_POINT('Ctrl Pts',(0.0557110953405879,0.113742055209456,
2.88953362862006));
#24302=CARTESIAN_POINT('Ctrl Pts',(0.0931089452052417,0.0954245105352619,
2.88690121711144));
#24303=CARTESIAN_POINT('Ctrl Pts',(0.120590118754061,0.0568606731642085,
2.88426880560283));
#24304=CARTESIAN_POINT('Ctrl Pts',(0.125696998005905,0.0155320946228576,
2.88163639409422));
#24305=CARTESIAN_POINT('Ctrl Pts',(0.130803877257748,-0.025796483918492,
2.87900398258561));
#24306=CARTESIAN_POINT('Ctrl Pts',(0.113536462212617,-0.0698898036301388,
2.87637157107699));
#24307=CARTESIAN_POINT('Ctrl Pts',(0.081722324704119,-0.0967597174754642,
2.87373915956838));
#24308=CARTESIAN_POINT('Ctrl Pts',(0.0499081871956208,-0.12362963132079,
2.87110674805977));
#24309=CARTESIAN_POINT('Ctrl Pts',(0.0035473272237559,-0.133276139299794,
2.86847433655116));
#24310=CARTESIAN_POINT('Ctrl Pts',(-0.0363441991716402,-0.12132633857832,
2.86584192504255));
#24311=CARTESIAN_POINT('Ctrl Pts',(-0.0762357255670363,-0.109376537856846,
2.86320951353394));
#24312=CARTESIAN_POINT('Ctrl Pts',(-0.109657918385963,-0.0758304284348936,
2.86057710202533));
#24313=CARTESIAN_POINT('Ctrl Pts',(-0.121460008724635,-0.035894951779346,
2.85794469051671));
#24314=CARTESIAN_POINT('Ctrl Pts',(-0.124877324339263,-0.0243315656302484,
2.85718247122383));
#24315=CARTESIAN_POINT('Ctrl Pts',(-0.126482006208201,-0.0122324936456281,
2.85642025193094));
#24316=CARTESIAN_POINT('Ctrl Pts',(-0.126382098607383,-0.000107526861324363,
2.85565803263806));
#24317=CARTESIAN_POINT('Ctrl Pts',(-0.126249156657861,1.39511119994357E-5,
2.86934196736194));
#24318=CARTESIAN_POINT('Ctrl Pts',(-0.126227407627626,-0.0218501465218449,
2.87071278611567));
#24319=CARTESIAN_POINT('Ctrl Pts',(-0.120828074559444,-0.0437243044457016,
2.8720836048694));
#24320=CARTESIAN_POINT('Ctrl Pts',(-0.110113563989691,-0.0625778327914941,
2.87345442362312));
#24321=CARTESIAN_POINT('Ctrl Pts',(-0.0895382684910942,-0.0987826518898959,
2.87608683513174));
#24322=CARTESIAN_POINT('Ctrl Pts',(-0.049362558315506,-0.12384850294854,
2.87871924664035));
#24323=CARTESIAN_POINT('Ctrl Pts',(-0.00779867057972899,-0.126412668959158,
2.88135165814896));
#24324=CARTESIAN_POINT('Ctrl Pts',(0.0337652171560469,-0.128976834969775,
2.88398406965757));
#24325=CARTESIAN_POINT('Ctrl Pts',(0.0767172824520115,-0.109039315932365,
2.88661648116618));
#24326=CARTESIAN_POINT('Ctrl Pts',(0.101586725761179,-0.0756380809090063,
2.88924889267479));
#24327=CARTESIAN_POINT('Ctrl Pts',(0.126456169070347,-0.0422368458856463,
2.89188130418341));
#24328=CARTESIAN_POINT('Ctrl Pts',(0.133242990392717,0.00462810512366429,
2.89451371569202));
#24329=CARTESIAN_POINT('Ctrl Pts',(0.118870624347205,0.0437122042621813,
2.89714612720063));
#24330=CARTESIAN_POINT('Ctrl Pts',(0.104498258301693,0.0827963034006972,
2.89977853870924));
#24331=CARTESIAN_POINT('Ctrl Pts',(0.0689667048882996,0.11409955066842,
2.90241095021785));
#24332=CARTESIAN_POINT('Ctrl Pts',(0.0283829370476986,0.123431726145854,
2.90504336172646));
#24333=CARTESIAN_POINT('Ctrl Pts',(-0.0122008307929037,0.132763901623287,
2.90767577323508));
#24334=CARTESIAN_POINT('Ctrl Pts',(-0.0578368130607139,0.120125005310431,
2.91030818474369));
#24335=CARTESIAN_POINT('Ctrl Pts',(-0.0878375513946906,0.0912444338001155,
2.9129405962523));
#24336=CARTESIAN_POINT('Ctrl Pts',(-0.112155666680576,0.0678343076994951,
2.91507438662218));
#24337=CARTESIAN_POINT('Ctrl Pts',(-0.126200703597521,0.0337526498432798,
2.91720817699206));
#24338=CARTESIAN_POINT('Ctrl Pts',(-0.126504381589359,-0.000106615302056266,
2.91934196736194));
#24339=CARTESIAN_POINT('Origin',(0.,0.,3.1));
#24340=CARTESIAN_POINT('',(-0.126560384998288,9.09688539718206E-5,2.96934196736194));
#24341=CARTESIAN_POINT('',(-0.126299886768127,7.7729991388234E-5,2.95565803263806));
#24342=CARTESIAN_POINT('',(-0.12645,1.54856587752183E-17,3.1));
#24343=CARTESIAN_POINT('Ctrl Pts',(-0.126299886768127,7.7729991388234E-5,
2.95565803263806));
#24344=CARTESIAN_POINT('Ctrl Pts',(-0.126388830708229,0.0157273402429332,
2.95467585670095));
#24345=CARTESIAN_POINT('Ctrl Pts',(-0.123692081773928,0.0313473916688532,
2.95369368076385));
#24346=CARTESIAN_POINT('Ctrl Pts',(-0.118069607334697,0.0458317476680533,
2.95271150482674));
#24347=CARTESIAN_POINT('Ctrl Pts',(-0.103000345442256,0.0846524762021514,
2.95007909331813));
#24348=CARTESIAN_POINT('Ctrl Pts',(-0.066914478664464,0.115315070279254,
2.94744668180952));
#24349=CARTESIAN_POINT('Ctrl Pts',(-0.0261702583026162,0.123919727448441,
2.9448142703009));
#24350=CARTESIAN_POINT('Ctrl Pts',(0.0145739620592316,0.132524384617628,
2.94218185879229));
#24351=CARTESIAN_POINT('Ctrl Pts',(0.0599765360051347,0.119071104878899,
2.93954944728368));
#24352=CARTESIAN_POINT('Ctrl Pts',(0.0894558125827043,0.0896584567433833,
2.93691703577507));
#24353=CARTESIAN_POINT('Ctrl Pts',(0.118935089160275,0.0602458086078669,
2.93428462426646));
#24354=CARTESIAN_POINT('Ctrl Pts',(0.13249106836951,0.0148737920755634,
2.93165221275785));
#24355=CARTESIAN_POINT('Ctrl Pts',(0.123978626527973,-0.0258897940256335,
2.92901980124923));
#24356=CARTESIAN_POINT('Ctrl Pts',(0.115466184686436,-0.0666533801268299,
2.92638738974062));
#24357=CARTESIAN_POINT('Ctrl Pts',(0.0848853217941264,-0.10280853579692,
2.92375497823201));
#24358=CARTESIAN_POINT('Ctrl Pts',(0.0460987903596358,-0.117965600062524,
2.9211225667234));
#24359=CARTESIAN_POINT('Ctrl Pts',(0.00731225892514568,-0.133122664328129,
2.91849015521479));
#24360=CARTESIAN_POINT('Ctrl Pts',(-0.0396799410515272,-0.127281637189249,
2.91585774370617));
#24361=CARTESIAN_POINT('Ctrl Pts',(-0.0735755578837821,-0.103090341701714,
2.91322533219756));
#24362=CARTESIAN_POINT('Ctrl Pts',(-0.106055065170122,-0.0799097233361643,
2.91070289901106));
#24363=CARTESIAN_POINT('Ctrl Pts',(-0.126509442293762,-0.0398801022208299,
2.90818046582456));
#24364=CARTESIAN_POINT('Ctrl Pts',(-0.126643227510109,3.12951648517141E-5,
2.90565803263806));
#24365=CARTESIAN_POINT('Ctrl Pts',(-0.126504381589359,-0.000106615302056266,
2.91934196736194));
#24366=CARTESIAN_POINT('Ctrl Pts',(-0.126575344636262,-0.00801880085773389,
2.91984058850067));
#24367=CARTESIAN_POINT('Ctrl Pts',(-0.125895951346516,-0.0159188425067759,
2.9203392096394));
#24368=CARTESIAN_POINT('Ctrl Pts',(-0.124421945835367,-0.0236677318103004,
2.92083783077814));
#24369=CARTESIAN_POINT('Ctrl Pts',(-0.116640107541925,-0.0645770792026294,
2.92347024228675));
#24370=CARTESIAN_POINT('Ctrl Pts',(-0.0867109365548968,-0.101273527279515,
2.92610265379536));
#24371=CARTESIAN_POINT('Ctrl Pts',(-0.0482017639084,-0.117122039303909,
2.92873506530397));
#24372=CARTESIAN_POINT('Ctrl Pts',(-0.0096925912619021,-0.132970551328304,
2.93136747681259));
#24373=CARTESIAN_POINT('Ctrl Pts',(0.0373965830440653,-0.127971127300206,
2.9339998883212));
#24374=CARTESIAN_POINT('Ctrl Pts',(0.071719547440819,-0.104390079267275,
2.93663229982981));
#24375=CARTESIAN_POINT('Ctrl Pts',(0.106042511837572,-0.0808090312343449,
2.93926471133842));
#24376=CARTESIAN_POINT('Ctrl Pts',(0.127599266325111,-0.0386463591965834,
2.94189712284703));
#24377=CARTESIAN_POINT('Ctrl Pts',(0.126617818746111,0.00298498082453686,
2.94452953435564));
#24378=CARTESIAN_POINT('Ctrl Pts',(0.125636371167111,0.0446163208456583,
2.94716194586426));
#24379=CARTESIAN_POINT('Ctrl Pts',(0.10211672152157,0.0857163288501385,
2.94979435737287));
#24380=CARTESIAN_POINT('Ctrl Pts',(0.0667206710566959,0.107653769967896,
2.95242676888148));
#24381=CARTESIAN_POINT('Ctrl Pts',(0.0313246205918224,0.129591211085654,
2.95505918039009));
#24382=CARTESIAN_POINT('Ctrl Pts',(-0.0159478306923833,0.13236608531669,
2.9576915918987));
#24383=CARTESIAN_POINT('Ctrl Pts',(-0.0536673890921198,0.114720501579208,
2.96032400340732));
#24384=CARTESIAN_POINT('Ctrl Pts',(-0.0913869474918552,0.0970749178417258,
2.96295641491593));
#24385=CARTESIAN_POINT('Ctrl Pts',(-0.119553613007122,0.059008876135727,
2.96558882642454));
#24386=CARTESIAN_POINT('Ctrl Pts',(-0.125399024116903,0.0177782700249248,
2.96822123793315));
#24387=CARTESIAN_POINT('Ctrl Pts',(-0.12622857074271,0.0119270630632909,
2.96859481440941));
#24388=CARTESIAN_POINT('Ctrl Pts',(-0.126608575570408,0.00601212294639071,
2.96896839088568));
#24389=CARTESIAN_POINT('Ctrl Pts',(-0.126560384998288,9.09688539718206E-5,
2.96934196736194));
#24390=CARTESIAN_POINT('Origin',(0.,0.,3.1));
#24391=CARTESIAN_POINT('',(-0.126250113253048,1.79623087654263E-5,3.01934196736194));
#24392=CARTESIAN_POINT('',(-0.126375290424941,-0.000106230050797054,3.00565803263806));
#24393=CARTESIAN_POINT('',(-0.12645,1.54856587752183E-17,3.1));
#24394=CARTESIAN_POINT('Ctrl Pts',(-0.126375290424941,-0.000106230050797054,
3.00565803263806));
#24395=CARTESIAN_POINT('Ctrl Pts',(-0.126136144258534,0.0293961593132966,
3.00380365908596));
#24396=CARTESIAN_POINT('Ctrl Pts',(-0.115821844223656,0.0590492800488679,
3.00194928553385));
#24397=CARTESIAN_POINT('Ctrl Pts',(-0.0969443855366137,0.0815031740695626,
3.00009491198175));
#24398=CARTESIAN_POINT('Ctrl Pts',(-0.0701465273355013,0.11337802957871,
2.99746250047314));
#24399=CARTESIAN_POINT('Ctrl Pts',(-0.0260923921578653,0.130745171841498,
2.99483008896453));
#24400=CARTESIAN_POINT('Ctrl Pts',(0.0152476360635642,0.125731821210699,
2.99219767745592));
#24401=CARTESIAN_POINT('Ctrl Pts',(0.0565876642849942,0.120718470579899,
2.98956526594731));
#24402=CARTESIAN_POINT('Ctrl Pts',(0.0952135855502181,0.0933246270555131,
2.98693285443869));
#24403=CARTESIAN_POINT('Ctrl Pts',(0.113615704700958,0.0559683206447137,
2.98430044293008));
#24404=CARTESIAN_POINT('Ctrl Pts',(0.132017823851697,0.0186120142339143,
2.98166803142147));
#24405=CARTESIAN_POINT('Ctrl Pts',(0.130196140887953,-0.0287067550632971,
2.97903561991286));
#24406=CARTESIAN_POINT('Ctrl Pts',(0.108976451346127,-0.0645376969103253,
2.97640320840425));
#24407=CARTESIAN_POINT('Ctrl Pts',(0.0877567618043009,-0.100368638757354,
2.97377079689564));
#24408=CARTESIAN_POINT('Ctrl Pts',(0.0471390656843917,-0.124711753154198,
2.97113838538702));
#24409=CARTESIAN_POINT('Ctrl Pts',(0.00553595882347027,-0.126531950235485,
2.96850597387841));
#24410=CARTESIAN_POINT('Ctrl Pts',(-0.03606714803745,-0.128352147316772,
2.9658735623698));
#24411=CARTESIAN_POINT('Ctrl Pts',(-0.078655665639383,-0.107649427082503,
2.96324115086119));
#24412=CARTESIAN_POINT('Ctrl Pts',(-0.102923595936805,-0.0738086354698221,
2.96060873935258));
#24413=CARTESIAN_POINT('Ctrl Pts',(-0.118136947531953,-0.0525941414955858,
2.95895850378107));
#24414=CARTESIAN_POINT('Ctrl Pts',(-0.126150444648563,-0.0262164832362216,
2.95730826820956));
#24415=CARTESIAN_POINT('Ctrl Pts',(-0.126299886768127,7.7729991388234E-5,
2.95565803263806));
#24416=CARTESIAN_POINT('Ctrl Pts',(-0.126560384998288,9.09688539718206E-5,
2.96934196736194));
#24417=CARTESIAN_POINT('Ctrl Pts',(-0.126269000075926,-0.0357113665330736,
2.97160080239429));
#24418=CARTESIAN_POINT('Ctrl Pts',(-0.110322654377183,-0.0717408868526332,
2.97385963742664));
#24419=CARTESIAN_POINT('Ctrl Pts',(-0.0834402350166293,-0.0952822612815302,
2.97611847245899));
#24420=CARTESIAN_POINT('Ctrl Pts',(-0.0521118781022804,-0.122717015961572,
2.9787508839676));
#24421=CARTESIAN_POINT('Ctrl Pts',(-0.00593100756928766,-0.133191354806051,
2.98138329547621));
#24422=CARTESIAN_POINT('Ctrl Pts',(0.0341679124015605,-0.12195710679034,
2.98401570698482));
#24423=CARTESIAN_POINT('Ctrl Pts',(0.0742668323724097,-0.110722858774629,
2.98664811849343));
#24424=CARTESIAN_POINT('Ctrl Pts',(0.108283801781115,-0.0777800238987277,
2.98928053000205));
#24425=CARTESIAN_POINT('Ctrl Pts',(0.120798430769142,-0.038062071124208,
2.99191294151066));
#24426=CARTESIAN_POINT('Ctrl Pts',(0.133313059757168,0.00165588165031116,
2.99454535301927));
#24427=CARTESIAN_POINT('Ctrl Pts',(0.124325348324518,0.0481489523234473,
2.99717776452788));
#24428=CARTESIAN_POINT('Ctrl Pts',(0.0979095575425482,0.0803411518237943,
2.9998101760365));
#24429=CARTESIAN_POINT('Ctrl Pts',(0.0714937667605778,0.112533351324142,
3.00244258754511));
#24430=CARTESIAN_POINT('Ctrl Pts',(0.0276498966292865,0.130424679651699,
3.00507499905372));
#24431=CARTESIAN_POINT('Ctrl Pts',(-0.0137469851400152,0.125904735947905,
3.00770741056233));
#24432=CARTESIAN_POINT('Ctrl Pts',(-0.0551438669093158,0.121384792244111,
3.01033982207094));
#24433=CARTESIAN_POINT('Ctrl Pts',(-0.0940937603166274,0.0944535765089676,
3.01297223357955));
#24434=CARTESIAN_POINT('Ctrl Pts',(-0.112940108892359,0.0573194028051013,
3.01560464508816));
#24435=CARTESIAN_POINT('Ctrl Pts',(-0.121859038434214,0.039745861833548,
3.01685041917942));
#24436=CARTESIAN_POINT('Ctrl Pts',(-0.126275572181929,0.0198872634041666,
3.01809619327068));
#24437=CARTESIAN_POINT('Ctrl Pts',(-0.126250113253048,1.79623087654263E-5,
3.01934196736194));
#24438=CARTESIAN_POINT('Origin',(0.,0.,3.1));
#24439=CARTESIAN_POINT('',(-0.126496969333234,-0.000107906771987382,3.06934196736194));
#24440=CARTESIAN_POINT('',(-0.126645757366777,2.69067085927681E-5,3.05565803263806));
#24441=CARTESIAN_POINT('',(-0.12645,1.54856587752183E-17,3.1));
#24442=CARTESIAN_POINT('Ctrl Pts',(-0.126645757366777,2.69067085927681E-5,
3.05565803263806));
#24443=CARTESIAN_POINT('Ctrl Pts',(-0.126650109530876,0.00151667558283516,
3.05556387297957));
#24444=CARTESIAN_POINT('Ctrl Pts',(-0.126626072178,0.00300630074643505,
3.05546971332109));
#24445=CARTESIAN_POINT('Ctrl Pts',(-0.126573208557277,0.0044949022237674,
3.0553755536626));
#24446=CARTESIAN_POINT('Ctrl Pts',(-0.125095305962741,0.0461115746257868,
3.05274314215399));
#24447=CARTESIAN_POINT('Ctrl Pts',(-0.10108714199637,0.0869281462553232,
3.05011073064538));
#24448=CARTESIAN_POINT('Ctrl Pts',(-0.0654319685934297,0.108441868097491,
3.04747831913677));
#24449=CARTESIAN_POINT('Ctrl Pts',(-0.0297767951904896,0.129955589939659,
3.04484590762816));
#24450=CARTESIAN_POINT('Ctrl Pts',(0.0175253876490204,0.132166461994459,
3.04221349611954));
#24451=CARTESIAN_POINT('Ctrl Pts',(0.0550318084723819,0.114072263617167,
3.03958108461093));
#24452=CARTESIAN_POINT('Ctrl Pts',(0.092538229295744,0.095978065239874,
3.03694867310232));
#24453=CARTESIAN_POINT('Ctrl Pts',(0.120248888102957,0.0575787964304887,
3.03431626159371));
#24454=CARTESIAN_POINT('Ctrl Pts',(0.125602137884551,0.0162814074734155,
3.0316838500851));
#24455=CARTESIAN_POINT('Ctrl Pts',(0.130955387666146,-0.0250159814836577,
3.02905143857648));
#24456=CARTESIAN_POINT('Ctrl Pts',(0.113951228422121,-0.0692114905884188,
3.02641902706787));
#24457=CARTESIAN_POINT('Ctrl Pts',(0.0822978942873024,-0.0962706490388489,
3.02378661555926));
#24458=CARTESIAN_POINT('Ctrl Pts',(0.0506445601524839,-0.123329807489279,
3.02115420405065));
#24459=CARTESIAN_POINT('Ctrl Pts',(0.00434205112687179,-0.133252615285378,
3.01852179254204));
#24460=CARTESIAN_POINT('Ctrl Pts',(-0.0356200281006283,-0.121540918494949,
3.01588938103343));
#24461=CARTESIAN_POINT('Ctrl Pts',(-0.0755821073281284,-0.10982922170452,
3.01325696952481));
#24462=CARTESIAN_POINT('Ctrl Pts',(-0.109203756757516,-0.0764830203275614,
3.0106245580162));
#24463=CARTESIAN_POINT('Ctrl Pts',(-0.121243790859916,-0.0366186352613279,
3.00799214650759));
#24464=CARTESIAN_POINT('Ctrl Pts',(-0.124802354366684,-0.0248362810993748,
3.00721410855108));
#24465=CARTESIAN_POINT('Ctrl Pts',(-0.126475628781476,-0.012484522820876,
3.00643607059457));
#24466=CARTESIAN_POINT('Ctrl Pts',(-0.126375290424941,-0.000106230050797054,
3.00565803263806));
#24467=CARTESIAN_POINT('Ctrl Pts',(-0.126250113253048,1.79623087654263E-5,
3.01934196736194));
#24468=CARTESIAN_POINT('Ctrl Pts',(-0.126221775608494,-0.0220980188702133,
3.0207286047793));
#24469=CARTESIAN_POINT('Ctrl Pts',(-0.120690113995694,-0.0442272599176159,
3.02211524219665));
#24470=CARTESIAN_POINT('Ctrl Pts',(-0.109738425578795,-0.063233377942656,
3.023501879614));
#24471=CARTESIAN_POINT('Ctrl Pts',(-0.0889475899453455,-0.0993148533139586,
3.02613429112261));
#24472=CARTESIAN_POINT('Ctrl Pts',(-0.0486231149342947,-0.124140672383972,
3.02876670263122));
#24473=CARTESIAN_POINT('Ctrl Pts',(-0.00704467496461261,-0.126456928197685,
3.03139911413984));
#24474=CARTESIAN_POINT('Ctrl Pts',(0.0345337650050683,-0.128773184011397,
3.03403152564845));
#24475=CARTESIAN_POINT('Ctrl Pts',(0.0773661699333803,-0.108579876568808,
3.03666393715706));
#24476=CARTESIAN_POINT('Ctrl Pts',(0.102035984081992,-0.0750309275363891,
3.03929634866567));
#24477=CARTESIAN_POINT('Ctrl Pts',(0.126705798230605,-0.0414819785039689,
3.04192876017428));
#24478=CARTESIAN_POINT('Ctrl Pts',(0.133213021599516,0.00542261211828284,
3.0445611716829));
#24479=CARTESIAN_POINT('Ctrl Pts',(0.118607834643087,0.0444203072460051,
3.04719358319151));
#24480=CARTESIAN_POINT('Ctrl Pts',(0.104002647686659,0.0834180023737263,
3.04982599470012));
#24481=CARTESIAN_POINT('Ctrl Pts',(0.0682850504048921,0.114508802006919,
3.05245840620873));
#24482=CARTESIAN_POINT('Ctrl Pts',(0.0276463521492325,0.123598791852477,
3.05509081771734));
#24483=CARTESIAN_POINT('Ctrl Pts',(-0.0129923461064282,0.132688781698037,
3.05772322922596));
#24484=CARTESIAN_POINT('Ctrl Pts',(-0.0585521453359818,0.119777961755961,
3.06035564073457));
#24485=CARTESIAN_POINT('Ctrl Pts',(-0.0883801220659878,0.0907189955750862,
3.06298805224318));
#24486=CARTESIAN_POINT('Ctrl Pts',(-0.112378957568068,0.0673388865067503,
3.06510602394943));
#24487=CARTESIAN_POINT('Ctrl Pts',(-0.126193947985427,0.0335054291562246,
3.06722399565569));
#24488=CARTESIAN_POINT('Ctrl Pts',(-0.126496969333234,-0.000107906771987382,
3.06934196736194));
#24489=CARTESIAN_POINT('Origin',(0.,0.,3.1));
#24490=CARTESIAN_POINT('',(-0.126566979141993,8.83287276302464E-5,3.11934196736194));
#24491=CARTESIAN_POINT('',(-0.126304742691185,8.06358209441624E-5,3.10565803263806));
#24492=CARTESIAN_POINT('',(-0.12645,1.54856587752183E-17,3.1));
#24493=CARTESIAN_POINT('Ctrl Pts',(-0.126304742691185,8.06358209441624E-5,
3.10565803263806));
#24494=CARTESIAN_POINT('Ctrl Pts',(-0.12639574781383,0.0154767095828029,
3.10469167536458));
#24495=CARTESIAN_POINT('Ctrl Pts',(-0.123787659959305,0.0308430184790688,
3.1037253180911));
#24496=CARTESIAN_POINT('Ctrl Pts',(-0.118340823679398,0.0451268292855474,
3.10275896081762));
#24497=CARTESIAN_POINT('Ctrl Pts',(-0.103503335617549,0.0840367324711176,
3.10012654930901));
#24498=CARTESIAN_POINT('Ctrl Pts',(-0.0676009656676162,0.114913977953889,
3.09749413780039));
#24499=CARTESIAN_POINT('Ctrl Pts',(-0.0269087833345171,0.123761458661173,
3.09486172629178));
#24500=CARTESIAN_POINT('Ctrl Pts',(0.0137833989985814,0.132608939368457,
3.09222931478317));
#24501=CARTESIAN_POINT('Ctrl Pts',(0.0592653937148459,0.119426655300253,
3.08959690327456));
#24502=CARTESIAN_POINT('Ctrl Pts',(0.0889195472648929,0.0901903286649502,
3.08696449176595));
#24503=CARTESIAN_POINT('Ctrl Pts',(0.11857370081494,0.0609540020296468,
3.08433208025733));
#24504=CARTESIAN_POINT('Ctrl Pts',(0.13240001319877,0.015663632827244,3.08169966874872));
#24505=CARTESIAN_POINT('Ctrl Pts',(0.124130814751194,-0.0251499920415489,
3.07906725724011));
#24506=CARTESIAN_POINT('Ctrl Pts',(0.115861616303618,-0.0659636169103418,
3.0764348457315));
#24507=CARTESIAN_POINT('Ctrl Pts',(0.085496907024637,-0.102300497445525,
3.07380243422289));
#24508=CARTESIAN_POINT('Ctrl Pts',(0.0468014538280004,-0.117688594137541,
3.07117002271428));
#24509=CARTESIAN_POINT('Ctrl Pts',(0.0081060006313637,-0.133076690829557,
3.06853761120566));
#24510=CARTESIAN_POINT('Ctrl Pts',(-0.0389201964829282,-0.127516003678407,
3.06590519969705));
#24511=CARTESIAN_POINT('Ctrl Pts',(-0.0729594744287227,-0.103527273515581,
3.06327278818844));
#24512=CARTESIAN_POINT('Ctrl Pts',(-0.105781189400045,-0.0803966047281269,
3.06073453633831));
#24513=CARTESIAN_POINT('Ctrl Pts',(-0.12652843654431,-0.0401326336098284,
3.05819628448819));
#24514=CARTESIAN_POINT('Ctrl Pts',(-0.126645757366777,2.69067085927681E-5,
3.05565803263806));
#24515=CARTESIAN_POINT('Ctrl Pts',(-0.126496969333234,-0.000107906771987382,
3.06934196736194));
#24516=CARTESIAN_POINT('Ctrl Pts',(-0.126570570997419,-0.00827233967750279,
3.0698564071643));
#24517=CARTESIAN_POINT('Ctrl Pts',(-0.125847009061939,-0.0164237861126916,
3.07037084696666));
#24518=CARTESIAN_POINT('Ctrl Pts',(-0.124278591835651,-0.0244092963007763,
3.07088528676901));
#24519=CARTESIAN_POINT('Ctrl Pts',(-0.116252930644851,-0.0652715095760922,
3.07351769827763));
#24520=CARTESIAN_POINT('Ctrl Pts',(-0.0861054540327919,-0.101788823707051,
3.07615010978624));
#24521=CARTESIAN_POINT('Ctrl Pts',(-0.0475024541674668,-0.117407405995615,
3.07878252129485));
#24522=CARTESIAN_POINT('Ctrl Pts',(-0.00889945430214065,-0.133025988284179,
3.08141493280346));
#24523=CARTESIAN_POINT('Ctrl Pts',(0.0381590688164514,-0.127745838730347,
3.08404734431207));
#24524=CARTESIAN_POINT('Ctrl Pts',(0.072340798251519,-0.103960526368831,
3.08667975582068));
#24525=CARTESIAN_POINT('Ctrl Pts',(0.106522527686585,-0.0801752140073166,
3.0893121673293));
#24526=CARTESIAN_POINT('Ctrl Pts',(0.127827463438127,-0.0378847388381192,
3.09194457883791));
#24527=CARTESIAN_POINT('Ctrl Pts',(0.1265977664655,0.00374000808798695,
3.09457699034652));
#24528=CARTESIAN_POINT('Ctrl Pts',(0.125368069492872,0.0453647550140949,
3.09720940185513));
#24529=CARTESIAN_POINT('Ctrl Pts',(0.101603739796073,0.0863237736971122,
3.09984181336374));
#24530=CARTESIAN_POINT('Ctrl Pts',(0.066077495668981,0.108049741788989,
3.10247422487236));
#24531=CARTESIAN_POINT('Ctrl Pts',(0.0305512515418895,0.129775709880865,
3.10510663638097));
#24532=CARTESIAN_POINT('Ctrl Pts',(-0.0167369070154944,0.132268627381602,
3.10773904788958));
#24533=CARTESIAN_POINT('Ctrl Pts',(-0.0543505659626984,0.114398418319861,
3.11037145939819));
#24534=CARTESIAN_POINT('Ctrl Pts',(-0.0919642249099026,0.096528209258119,
3.1130038709068));
#24535=CARTESIAN_POINT('Ctrl Pts',(-0.119903384246927,0.0582948736338987,
3.11563628241541));
#24536=CARTESIAN_POINT('Ctrl Pts',(-0.125502814331461,0.0170301417913753,
3.11826869392403));
#24537=CARTESIAN_POINT('Ctrl Pts',(-0.126263804720884,0.011422059561536,
3.11862645173666));
#24538=CARTESIAN_POINT('Ctrl Pts',(-0.126612176704445,0.00575798695415024,
3.1189842095493));
#24539=CARTESIAN_POINT('Ctrl Pts',(-0.126566979141993,8.83287276302464E-5,
3.11934196736194));
#24540=CARTESIAN_POINT('Origin',(0.,0.,3.1));
#24541=CARTESIAN_POINT('',(-0.126251310180948,2.19509288584552E-5,3.16934196736194));
#24542=CARTESIAN_POINT('',(-0.126368593930883,-0.000104790611567188,3.15565803263806));
#24543=CARTESIAN_POINT('',(-0.12645,1.54856587752183E-17,3.1));
#24544=CARTESIAN_POINT('Ctrl Pts',(-0.126368593930883,-0.000104790611567188,
3.15565803263806));
#24545=CARTESIAN_POINT('Ctrl Pts',(-0.126135626550864,0.029149858613393,
3.15381947774958));
#24546=CARTESIAN_POINT('Ctrl Pts',(-0.116012034435359,0.0585500300902377,
3.15198092286111));
#24547=CARTESIAN_POINT('Ctrl Pts',(-0.0974287026581059,0.0809236008148654,
3.15014236797263));
#24548=CARTESIAN_POINT('Ctrl Pts',(-0.0708214054023045,0.112957697503196,
3.14750995646402));
#24549=CARTESIAN_POINT('Ctrl Pts',(-0.0268716218413343,0.130587246038798,
3.1448775449554));
#24550=CARTESIAN_POINT('Ctrl Pts',(0.014497568206441,0.125820514172312,
3.14224513344679));
#24551=CARTESIAN_POINT('Ctrl Pts',(0.0558667582542159,0.121053782305825,
3.13961272193818));
#24552=CARTESIAN_POINT('Ctrl Pts',(0.0946553547887964,0.0938907700372525,
3.13698031042957));
#24553=CARTESIAN_POINT('Ctrl Pts',(0.113279919572572,0.0566448681887155,
3.13434789892096));
#24554=CARTESIAN_POINT('Ctrl Pts',(0.131904484356347,0.0193989663401779,
3.13171548741235));
#24555=CARTESIAN_POINT('Ctrl Pts',(0.130365017389317,-0.0279298250883239,
3.12908307590374));
#24556=CARTESIAN_POINT('Ctrl Pts',(0.109359381568105,-0.0638866725814309,
3.12645066439512));
#24557=CARTESIAN_POINT('Ctrl Pts',(0.0883537457468925,-0.0998435200745383,
3.12381825288651));
#24558=CARTESIAN_POINT('Ctrl Pts',(0.0478819410714995,-0.12442842363225,
3.1211858413779));
#24559=CARTESIAN_POINT('Ctrl Pts',(0.00629042865298903,-0.126496686825572,
3.11855342986929));
#24560=CARTESIAN_POINT('Ctrl Pts',(-0.0353010837655206,-0.128564950018895,
3.11592101836068));
#24561=CARTESIAN_POINT('Ctrl Pts',(-0.0780123039271484,-0.108116572847827,
3.11328860685206));
#24562=CARTESIAN_POINT('Ctrl Pts',(-0.102481610921079,-0.0744211038181091,
3.11065619534345));
#24563=CARTESIAN_POINT('Ctrl Pts',(-0.117968244532349,-0.0530952287799418,
3.10899014110832));
#24564=CARTESIAN_POINT('Ctrl Pts',(-0.12614784474654,-0.0264630603867145,
3.10732408687319));
#24565=CARTESIAN_POINT('Ctrl Pts',(-0.126304742691185,8.06358209441624E-5,
3.10565803263806));
#24566=CARTESIAN_POINT('Ctrl Pts',(-0.126566979141993,8.83287276302464E-5,
3.11934196736194));
#24567=CARTESIAN_POINT('Ctrl Pts',(-0.126279609310085,-0.0359598261533815,
3.12161662105791));
#24568=CARTESIAN_POINT('Ctrl Pts',(-0.110082106605306,-0.0722337808796859,
3.12389127475389));
#24569=CARTESIAN_POINT('Ctrl Pts',(-0.0828705393299942,-0.0957781595443726,
3.12616592844986));
#24570=CARTESIAN_POINT('Ctrl Pts',(-0.0513791334119502,-0.12302560097677,
3.12879833995848));
#24571=CARTESIAN_POINT('Ctrl Pts',(-0.00513662074381884,-0.133224355780737,
3.13143075146709));
#24572=CARTESIAN_POINT('Ctrl Pts',(0.034894591212013,-0.121751179208655,
3.1340631629757));
#24573=CARTESIAN_POINT('Ctrl Pts',(0.0749258031678458,-0.110278002636571,
3.13669557448431));
#24574=CARTESIAN_POINT('Ctrl Pts',(0.108745714411378,-0.0771328946884361,
3.13932798599292));
#24575=CARTESIAN_POINT('Ctrl Pts',(0.12102326443306,-0.0373410176684702,
3.14196039750153));
#24576=CARTESIAN_POINT('Ctrl Pts',(0.133300814454742,0.00245085935149471,
3.14459280901015));
#24577=CARTESIAN_POINT('Ctrl Pts',(0.124036003254574,0.0488895054432904,
3.14722522051876));
#24578=CARTESIAN_POINT('Ctrl Pts',(0.097428705282154,0.0809236029943958,
3.14985763202737));
#24579=CARTESIAN_POINT('Ctrl Pts',(0.0708214073097326,0.112957700545502,
3.15249004353598));
#24580=CARTESIAN_POINT('Ctrl Pts',(0.0268716225650577,0.130587249555918,
3.15512245504459));
#24581=CARTESIAN_POINT('Ctrl Pts',(-0.0144975685969178,0.125820517561044,
3.15775486655321));
#24582=CARTESIAN_POINT('Ctrl Pts',(-0.0558667597588919,0.121053785566171,
3.16038727806182));
#24583=CARTESIAN_POINT('Ctrl Pts',(-0.0946553573381664,0.0938907725660106,
3.16301968957043));
#24584=CARTESIAN_POINT('Ctrl Pts',(-0.113279922623555,0.0566448697143249,
3.16565210107904));
#24585=CARTESIAN_POINT('Ctrl Pts',(-0.121981975887314,0.039242271290916,
3.16688205650667));
#24586=CARTESIAN_POINT('Ctrl Pts',(-0.126282044039751,0.0196384895744722,
3.16811201193431));
#24587=CARTESIAN_POINT('Ctrl Pts',(-0.126251310180948,2.19509288584552E-5,
3.16934196736194));
#24588=CARTESIAN_POINT('Origin',(0.,0.,3.1));
#24589=CARTESIAN_POINT('',(-0.126489518850073,-0.000109039769437509,3.21934196736194));
#24590=CARTESIAN_POINT('',(-0.126647930997008,2.24668189870201E-5,3.20565803263806));
#24591=CARTESIAN_POINT('',(-0.12645,1.54856587752183E-17,3.1));
#24592=CARTESIAN_POINT('Ctrl Pts',(-0.126647930997008,2.24668189870201E-5,
3.20565803263806));
#24593=CARTESIAN_POINT('Ctrl Pts',(-0.126650996831423,0.00126189995630808,
3.2055796916432));
#24594=CARTESIAN_POINT('Ctrl Pts',(-0.126634359036856,0.00250124877863209,
3.20550135064834));
#24595=CARTESIAN_POINT('Ctrl Pts',(-0.126597763055832,0.00374000798724603,
3.20542300965348));
#24596=CARTESIAN_POINT('Ctrl Pts',(-0.125368066116328,0.0453647537922705,
3.20279059814487));
#24597=CARTESIAN_POINT('Ctrl Pts',(-0.10160373705958,0.0863237713721372,
3.20015818663626));
#24598=CARTESIAN_POINT('Ctrl Pts',(-0.0660774938893213,0.10804973887887,
3.19752577512764));
#24599=CARTESIAN_POINT('Ctrl Pts',(-0.0305512507190632,0.129775706385603,
3.19489336361903));
#24600=CARTESIAN_POINT('Ctrl Pts',(0.0167369065647044,0.132268623819202,
3.19226095211042));
#24601=CARTESIAN_POINT('Ctrl Pts',(0.0543505644988585,0.114398415238764,
3.18962854060181));
#24602=CARTESIAN_POINT('Ctrl Pts',(0.091964222433013,0.0965282066583261,
3.1869961290932));
#24603=CARTESIAN_POINT('Ctrl Pts',(0.119903381017553,0.0582948720638503,
3.18436371758459));
#24604=CARTESIAN_POINT('Ctrl Pts',(0.125502810951281,0.0170301413327138,
3.18173130607597));
#24605=CARTESIAN_POINT('Ctrl Pts',(0.13110224088501,-0.0242345893984227,
3.17909889456736));
#24606=CARTESIAN_POINT('Ctrl Pts',(0.114361942167926,-0.0685307162662204,
3.17646648305875));
#24607=CARTESIAN_POINT('Ctrl Pts',(0.0828705370980449,-0.0957781569647633,
3.17383407155014));
#24608=CARTESIAN_POINT('Ctrl Pts',(0.0513791320281642,-0.123025597663306,
3.17120166004152));
#24609=CARTESIAN_POINT('Ctrl Pts',(0.00513662060548718,-0.133224352192594,
3.16856924853291));
#24610=CARTESIAN_POINT('Ctrl Pts',(-0.0348945902721819,-0.121751175929524,
3.1659368370243));
#24611=CARTESIAN_POINT('Ctrl Pts',(-0.0749258011498519,-0.110277999666453,
3.16330442551569));
#24612=CARTESIAN_POINT('Ctrl Pts',(-0.108745711482513,-0.0771328926110206,
3.16067201400708));
#24613=CARTESIAN_POINT('Ctrl Pts',(-0.121023261173527,-0.0373410166627737,
3.15803960249846));
#24614=CARTESIAN_POINT('Ctrl Pts',(-0.124725803146683,-0.0253409763781187,
3.15724574587833));
#24615=CARTESIAN_POINT('Ctrl Pts',(-0.126469185269255,-0.0127364488245176,
3.15645188925819));
#24616=CARTESIAN_POINT('Ctrl Pts',(-0.126368593930883,-0.000104790611567188,
3.15565803263806));
#24617=CARTESIAN_POINT('Ctrl Pts',(-0.126251310180948,2.19509288584552E-5,
3.16934196736194));
#24618=CARTESIAN_POINT('Ctrl Pts',(-0.126216265913324,-0.0223457977660937,
3.17074442344292));
#24619=CARTESIAN_POINT('Ctrl Pts',(-0.120550447304899,-0.0447301326243598,
3.1721468795239));
#24620=CARTESIAN_POINT('Ctrl Pts',(-0.109359384513483,-0.0638866743021069,
3.17354933560488));
#24621=CARTESIAN_POINT('Ctrl Pts',(-0.0883537481265213,-0.0998435227636405,
3.17618174711349));
#24622=CARTESIAN_POINT('Ctrl Pts',(-0.0478819423610949,-0.124428426983496,
3.1788141586221));
#24623=CARTESIAN_POINT('Ctrl Pts',(-0.00629042882239688,-0.126496690232519,
3.18144657013071));
#24624=CARTESIAN_POINT('Ctrl Pts',(0.0353010847163008,-0.128564953481541,
3.18407898163933));
#24625=CARTESIAN_POINT('Ctrl Pts',(0.0780123060282702,-0.108116575759732,
3.18671139314794));
#24626=CARTESIAN_POINT('Ctrl Pts',(0.102481613681232,-0.0744211058224891,
3.18934380465655));
#24627=CARTESIAN_POINT('Ctrl Pts',(0.126950921334194,-0.040725635885246,
3.19197621616516));
#24628=CARTESIAN_POINT('Ctrl Pts',(0.133178315328148,0.00621692626743081,
3.19460862767377));
#24629=CARTESIAN_POINT('Ctrl Pts',(0.118340826866677,0.0451268305009631,
3.19724103918239));
#24630=CARTESIAN_POINT('Ctrl Pts',(0.103503338405205,0.0840367347344954,
3.199873450691));
#24631=CARTESIAN_POINT('Ctrl Pts',(0.0676009674883078,0.114913981048883,
3.20250586219961));
#24632=CARTESIAN_POINT('Ctrl Pts',(0.026908784059242,0.123761461994453,
3.20513827370822));
#24633=CARTESIAN_POINT('Ctrl Pts',(-0.0137833993698235,0.132608942940023,
3.20777068521683));
#24634=CARTESIAN_POINT('Ctrl Pts',(-0.0592653953110574,0.119426658516775,
3.21040309672544));
#24635=CARTESIAN_POINT('Ctrl Pts',(-0.0889195496597795,0.0901903310940448,
3.21303550823405));
#24636=CARTESIAN_POINT('Ctrl Pts',(-0.11260033459284,0.0668432083338218,
3.21513766127668));
#24637=CARTESIAN_POINT('Ctrl Pts',(-0.126187596109782,0.0332583119648893,
3.21723981431931));
#24638=CARTESIAN_POINT('Ctrl Pts',(-0.126489518850073,-0.000109039769437509,
3.21934196736194));
#24639=CARTESIAN_POINT('Origin',(0.,0.,3.1));
#24640=CARTESIAN_POINT('',(-0.126573425356775,8.55484528903966E-5,3.26934196736194));
#24641=CARTESIAN_POINT('',(-0.126309785017077,8.34376343069358E-5,3.25565803263806));
#24642=CARTESIAN_POINT('',(-0.12645,1.54856587752183E-17,3.1));
#24643=CARTESIAN_POINT('Ctrl Pts',(-0.126309785017077,8.34376343069358E-5,
3.25565803263806));
#24644=CARTESIAN_POINT('Ctrl Pts',(-0.126402648710969,0.0152259667938181,
3.2547074940282));
#24645=CARTESIAN_POINT('Ctrl Pts',(-0.123881624579711,0.0303386118332616,
3.25375695541835));
#24646=CARTESIAN_POINT('Ctrl Pts',(-0.118607831448617,0.0444203060496175,
3.25280641680849));
#24647=CARTESIAN_POINT('Ctrl Pts',(-0.104002644885555,0.0834180001270126,
3.25017400529988));
#24648=CARTESIAN_POINT('Ctrl Pts',(-0.0682850485657758,0.114508798922838,
3.24754159379127));
#24649=CARTESIAN_POINT('Ctrl Pts',(-0.0276463514046418,0.123598788523579,
3.24490918228266));
#24650=CARTESIAN_POINT('Ctrl Pts',(0.0129923457564923,0.13268877812432,
3.24227677077404));
#24651=CARTESIAN_POINT('Ctrl Pts',(0.0585521437589804,0.119777958529977,
3.23964435926544));
#24652=CARTESIAN_POINT('Ctrl Pts',(0.0883801196856296,0.090718993131753,
3.23701194775682));
#24653=CARTESIAN_POINT('Ctrl Pts',(0.118208095612278,0.0616600277335293,
3.23437953624821));
#24654=CARTESIAN_POINT('Ctrl Pts',(0.132304249463088,0.0164529165314243,
3.2317471247396));
#24655=CARTESIAN_POINT('Ctrl Pts',(0.124278588488448,-0.024409295643347,
3.22911471323098));
#24656=CARTESIAN_POINT('Ctrl Pts',(0.116252927513807,-0.0652715078181186,
3.22648230172237));
#24657=CARTESIAN_POINT('Ctrl Pts',(0.0861054517137156,-0.101788820965557,
3.22384989021376));
#24658=CARTESIAN_POINT('Ctrl Pts',(0.0475024528880895,-0.117407402833467,
3.22121747870515));
#24659=CARTESIAN_POINT('Ctrl Pts',(0.00889945406246312,-0.133025984701378,
3.21858506719654));
#24660=CARTESIAN_POINT('Ctrl Pts',(-0.0381590677886978,-0.127745835289761,
3.21595265568793));
#24661=CARTESIAN_POINT('Ctrl Pts',(-0.0723407963031478,-0.103960523568861,
3.21332024417931));
#24662=CARTESIAN_POINT('Ctrl Pts',(-0.105505271014729,-0.0808830665952798,
3.21076617366556));
#24663=CARTESIAN_POINT('Ctrl Pts',(-0.126547978765194,-0.0403854911787608,
3.20821210315181));
#24664=CARTESIAN_POINT('Ctrl Pts',(-0.126647930997008,2.24668189870201E-5,
3.20565803263806));
#24665=CARTESIAN_POINT('Ctrl Pts',(-0.126489518850073,-0.000109039769437509,
3.21934196736194));
#24666=CARTESIAN_POINT('Ctrl Pts',(-0.126565677476903,-0.00852580124482262,
3.21987222582793));
#24667=CARTESIAN_POINT('Ctrl Pts',(-0.125796519899578,-0.0169287208447501,
3.22040248429391));
#24668=CARTESIAN_POINT('Ctrl Pts',(-0.124130818094417,-0.0251499927189283,
3.22093274275989));
#24669=CARTESIAN_POINT('Ctrl Pts',(-0.115861619424122,-0.065963618686957,
3.2235651542685));
#24670=CARTESIAN_POINT('Ctrl Pts',(-0.0854969093273219,-0.102300500200801,
3.22619756577711));
#24671=CARTESIAN_POINT('Ctrl Pts',(-0.0468014550884958,-0.117688597307262,
3.22882997728573));
#24672=CARTESIAN_POINT('Ctrl Pts',(-0.00810600084966979,-0.133076694413723,
3.23146238879434));
#24673=CARTESIAN_POINT('Ctrl Pts',(0.038920197531182,-0.127516007112802,
3.23409480030295));
#24674=CARTESIAN_POINT('Ctrl Pts',(0.0729594763937567,-0.103527276303882,
3.23672721181156));
#24675=CARTESIAN_POINT('Ctrl Pts',(0.106998755256331,-0.0795385454949616,
3.23935962332018));
#24676=CARTESIAN_POINT('Ctrl Pts',(0.128051114600629,-0.0371217711780427,
3.24199203482878));
#24677=CARTESIAN_POINT('Ctrl Pts',(0.126573211966284,0.00449490234484176,
3.2446244463374));
#24678=CARTESIAN_POINT('Ctrl Pts',(0.125095309331938,0.0461115758677259,
3.24725685784601));
#24679=CARTESIAN_POINT('Ctrl Pts',(0.10108714471895,0.0869281485965757,
3.24988926935462));
#24680=CARTESIAN_POINT('Ctrl Pts',(0.0654319703557041,0.108441871018171,
3.25252168086323));
#24681=CARTESIAN_POINT('Ctrl Pts',(0.0297767959924581,0.129955593439766,
3.25515409237185));
#24682=CARTESIAN_POINT('Ctrl Pts',(-0.0175253881210462,0.132166465554107,
3.25778650388046));
#24683=CARTESIAN_POINT('Ctrl Pts',(-0.0550318099545696,0.114072266689479,
3.26041891538907));
#24684=CARTESIAN_POINT('Ctrl Pts',(-0.0925382317880931,0.09597806782485,
3.26305132689768));
#24685=CARTESIAN_POINT('Ctrl Pts',(-0.120248891341636,0.0575787979812516,
3.26568373840629));
#24686=CARTESIAN_POINT('Ctrl Pts',(-0.125602141267406,0.0162814079119122,
3.26831614991491));
#24687=CARTESIAN_POINT('Ctrl Pts',(-0.126297505847784,0.0109170511726472,
3.26865808906392));
#24688=CARTESIAN_POINT('Ctrl Pts',(-0.126615635779588,0.00550379470022512,
3.26900002821293));
#24689=CARTESIAN_POINT('Ctrl Pts',(-0.126573425356775,8.55484528903966E-5,
3.26934196736194));
#24690=CARTESIAN_POINT('Origin',(0.,0.,3.1));
#24691=CARTESIAN_POINT('',(-0.126252746279467,2.59119664437757E-5,3.31934196736194));
#24692=CARTESIAN_POINT('',(-0.126362016509238,-0.00010321110317447,3.30565803263806));
#24693=CARTESIAN_POINT('',(-0.12645,1.54856587752183E-17,3.1));
#24694=CARTESIAN_POINT('Ctrl Pts',(-0.126362016509238,-0.00010321110317447,
3.30565803263806));
#24695=CARTESIAN_POINT('Ctrl Pts',(-0.126135404540093,0.0289035586789932,
3.30383529641321));
#24696=CARTESIAN_POINT('Ctrl Pts',(-0.116200394811108,0.0580506048820654,
3.30201256018836));
#24697=CARTESIAN_POINT('Ctrl Pts',(-0.0979095549055491,0.080341149659951,
3.30018982396351));
#24698=CARTESIAN_POINT('Ctrl Pts',(-0.0714937648350404,0.112533348293265,
3.2975574124549));
#24699=CARTESIAN_POINT('Ctrl Pts',(-0.0276498958846022,0.130424676138957,
3.29492500094628));
#24700=CARTESIAN_POINT('Ctrl Pts',(0.0137469847697539,0.125904732556904,
3.29229258943767));
#24701=CARTESIAN_POINT('Ctrl Pts',(0.05514386542411,0.12138478897485,3.28966017792906));
#24702=CARTESIAN_POINT('Ctrl Pts',(0.0940937577823839,0.0944535739650504,
3.28702776642045));
#24703=CARTESIAN_POINT('Ctrl Pts',(0.112940105850529,0.057319401261323,
3.28439535491184));
#24704=CARTESIAN_POINT('Ctrl Pts',(0.131786453918674,0.0201852285575958,
3.28176294340322));
#24705=CARTESIAN_POINT('Ctrl Pts',(0.13052925769669,-0.0271519018400594,
3.27913053189461));
#24706=CARTESIAN_POINT('Ctrl Pts',(0.109738422623206,-0.0632333762395775,
3.276498120386));
#24707=CARTESIAN_POINT('Ctrl Pts',(0.0889475875497212,-0.099314850639096,
3.27386570887739));
#24708=CARTESIAN_POINT('Ctrl Pts',(0.0486231136247353,-0.124140669040477,
3.27123329736878));
#24709=CARTESIAN_POINT('Ctrl Pts',(0.00704467477488957,-0.126456924791809,
3.26860088586016));
#24710=CARTESIAN_POINT('Ctrl Pts',(-0.0345337640749562,-0.128773180543141,
3.26596847435155));
#24711=CARTESIAN_POINT('Ctrl Pts',(-0.0773661678496626,-0.108579873644424,
3.26333606284294));
#24712=CARTESIAN_POINT('Ctrl Pts',(-0.102035981333843,-0.0750309255155824,
3.26070365133433));
#24713=CARTESIAN_POINT('Ctrl Pts',(-0.117797761200207,-0.0535961815725874,
3.25902177843557));
#24714=CARTESIAN_POINT('Ctrl Pts',(-0.126145472985543,-0.026709592283637,
3.25733990553681));
#24715=CARTESIAN_POINT('Ctrl Pts',(-0.126309785017077,8.34376343069358E-5,
3.25565803263806));
#24716=CARTESIAN_POINT('Ctrl Pts',(-0.126573425356775,8.55484528903966E-5,
3.26934196736194));
#24717=CARTESIAN_POINT('Ctrl Pts',(-0.126290679707385,-0.0362084626390545,
3.27163243972154));
#24718=CARTESIAN_POINT('Ctrl Pts',(-0.109839596819478,-0.0727263630692267,
3.27392291208114));
#24719=CARTESIAN_POINT('Ctrl Pts',(-0.0822978965038287,-0.0962706516317226,
3.27621338444074));
#24720=CARTESIAN_POINT('Ctrl Pts',(-0.0506445615164858,-0.123329810810936,
3.27884579594935));
#24721=CARTESIAN_POINT('Ctrl Pts',(-0.00434205124380389,-0.133252618874282,
3.28147820745796));
#24722=CARTESIAN_POINT('Ctrl Pts',(0.0356200290599969,-0.121540921768417,
3.28411061896657));
#24723=CARTESIAN_POINT('Ctrl Pts',(0.0755821093637979,-0.109829224662552,
3.28674303047519));
#24724=CARTESIAN_POINT('Ctrl Pts',(0.109203759698717,-0.0764830223874748,
3.2893754419838));
#24725=CARTESIAN_POINT('Ctrl Pts',(0.121243794125388,-0.0366186362475693,
3.29200785349241));
#24726=CARTESIAN_POINT('Ctrl Pts',(0.133283828552059,0.00324574989233616,
3.29464026500102));
#24727=CARTESIAN_POINT('Ctrl Pts',(0.123742247070482,0.0496283198970706,
3.29727267650964));
#24728=CARTESIAN_POINT('Ctrl Pts',(0.0969443881476166,0.0815031762647041,
3.29990508801825));
#24729=CARTESIAN_POINT('Ctrl Pts',(0.0701465292247518,0.113378032632337,
3.30253749952686));
#24730=CARTESIAN_POINT('Ctrl Pts',(0.0260923928606002,0.130745175362871,
3.30516991103547));
#24731=CARTESIAN_POINT('Ctrl Pts',(-0.0152476364742436,0.125731824597042,
3.30780232254408));
#24732=CARTESIAN_POINT('Ctrl Pts',(-0.0565876658090873,0.120718473831214,
3.31043473405269));
#24733=CARTESIAN_POINT('Ctrl Pts',(-0.095213588114623,0.0933246295690233,
3.31306714556131));
#24734=CARTESIAN_POINT('Ctrl Pts',(-0.113615707760984,0.0559683221521016,
3.31569955706992));
#24735=CARTESIAN_POINT('Ctrl Pts',(-0.122103244730499,0.0387386200124153,
3.31691369383393));
#24736=CARTESIAN_POINT('Ctrl Pts',(-0.12628858288157,0.0193896083672227,
3.31812783059793));
#24737=CARTESIAN_POINT('Ctrl Pts',(-0.126252746279467,2.59119664437757E-5,
3.31934196736194));
#24738=CARTESIAN_POINT('Origin',(0.,0.,3.1));
#24739=CARTESIAN_POINT('',(-0.126482040448775,-0.000110013702131137,3.36934196736194));
#24740=CARTESIAN_POINT('',(-0.126649735277799,1.79833793418055E-5,3.35565803263806));
#24741=CARTESIAN_POINT('',(-0.12645,1.54856587752183E-17,3.1));
#24742=CARTESIAN_POINT('Ctrl Pts',(-0.126649735277799,1.79833793418055E-5,
3.35565803263806));
#24743=CARTESIAN_POINT('Ctrl Pts',(-0.126651722007443,0.00100711151136191,
3.35559551030682));
#24744=CARTESIAN_POINT('Ctrl Pts',(-0.126641125668946,0.0019961959922384,
3.35553298797559));
#24745=CARTESIAN_POINT('Ctrl Pts',(-0.126617815335903,0.00298498074413288,
3.35547046564436));
#24746=CARTESIAN_POINT('Ctrl Pts',(-0.12563636778334,0.0446163196439928,
3.35283805413574));
#24747=CARTESIAN_POINT('Ctrl Pts',(-0.102116718771259,0.085716326541524,
3.35020564262713));
#24748=CARTESIAN_POINT('Ctrl Pts',(-0.0667206692597134,0.107653767068442,
3.34757323111852));
#24749=CARTESIAN_POINT('Ctrl Pts',(-0.0313246197481669,0.12959120759536,
3.34494081960991));
#24750=CARTESIAN_POINT('Ctrl Pts',(0.0159478302628458,0.132366081751665,
3.3423084081013));
#24751=CARTESIAN_POINT('Ctrl Pts',(0.0536673876466801,0.114720498489436,
3.33967599659268));
#24752=CARTESIAN_POINT('Ctrl Pts',(0.0913869450305144,0.0970749152272078,
3.33704358508407));
#24753=CARTESIAN_POINT('Ctrl Pts',(0.11955360978717,0.059008874546446,3.33441117357546));
#24754=CARTESIAN_POINT('Ctrl Pts',(0.12539902073952,0.0177782695461103,
3.33177876206685));
#24755=CARTESIAN_POINT('Ctrl Pts',(0.13124443169187,-0.0234523354542255,
3.32914635055824));
#24756=CARTESIAN_POINT('Ctrl Pts',(0.114768588839913,-0.0678475047741352,
3.32651393904963));
#24757=CARTESIAN_POINT('Ctrl Pts',(0.083440232769335,-0.0952822587152781,
3.32388152754101));
#24758=CARTESIAN_POINT('Ctrl Pts',(0.0521118766987572,-0.122717012656421,
3.3212491160324));
#24759=CARTESIAN_POINT('Ctrl Pts',(0.00593100740955835,-0.133191351218797,
3.31861670452379));
#24760=CARTESIAN_POINT('Ctrl Pts',(-0.0341679114813036,-0.121957103505662,
3.31598429301518));
#24761=CARTESIAN_POINT('Ctrl Pts',(-0.0742668303721658,-0.110722855792528,
3.31335188150657));
#24762=CARTESIAN_POINT('Ctrl Pts',(-0.108283798864691,-0.0777800218038817,
3.31071946999795));
#24763=CARTESIAN_POINT('Ctrl Pts',(-0.120798427515664,-0.0380620700990904,
3.30808705848934));
#24764=CARTESIAN_POINT('Ctrl Pts',(-0.124647668210362,-0.0258456503973156,
3.30727738320558));
#24765=CARTESIAN_POINT('Ctrl Pts',(-0.126462679516819,-0.0129882705177865,
3.30646770792182));
#24766=CARTESIAN_POINT('Ctrl Pts',(-0.126362016509238,-0.00010321110317447,
3.30565803263806));
#24767=CARTESIAN_POINT('Ctrl Pts',(-0.126252746279467,2.59119664437757E-5,
3.31934196736194));
#24768=CARTESIAN_POINT('Ctrl Pts',(-0.126210884316958,-0.0225934851076951,
3.32076024210655));
#24769=CARTESIAN_POINT('Ctrl Pts',(-0.120409070525885,-0.0452329200835406,
3.32217851685115));
#24770=CARTESIAN_POINT('Ctrl Pts',(-0.108976454281191,-0.064537698648537,
3.32359679159575));
#24771=CARTESIAN_POINT('Ctrl Pts',(-0.0877567641678496,-0.100368641460601,
3.32622920310437));
#24772=CARTESIAN_POINT('Ctrl Pts',(-0.047139066953979,-0.124711756513075,
3.32886161461298));
#24773=CARTESIAN_POINT('Ctrl Pts',(-0.00553595897255799,-0.126531953643381,
3.33149402612159));
#24774=CARTESIAN_POINT('Ctrl Pts',(0.0360671490088627,-0.128352150773687,
3.3341264376302));
#24775=CARTESIAN_POINT('Ctrl Pts',(0.0786556677578339,-0.107649429981826,
3.33675884913881));
#24776=CARTESIAN_POINT('Ctrl Pts',(0.102923598708863,-0.0738086374577052,
3.33939126064743));
#24777=CARTESIAN_POINT('Ctrl Pts',(0.127191529659892,-0.0399678449335842,
3.34202367215604));
#24778=CARTESIAN_POINT('Ctrl Pts',(0.133138872812978,0.00701101932279596,
3.34465608366465));
#24779=CARTESIAN_POINT('Ctrl Pts',(0.118069610514671,0.0458317489024548,
3.34728849517326));
#24780=CARTESIAN_POINT('Ctrl Pts',(0.103000348216365,0.0846524784821133,
3.34992090668187));
#24781=CARTESIAN_POINT('Ctrl Pts',(0.0669144804666656,0.11531507338505,
3.35255331819048));
#24782=CARTESIAN_POINT('Ctrl Pts',(0.0261702590074494,0.123919730785983,
3.3551857296991));
#24783=CARTESIAN_POINT('Ctrl Pts',(-0.0145739624517671,0.132524388186917,
3.35781814120771));
#24784=CARTESIAN_POINT('Ctrl Pts',(-0.059976537620501,0.119071108085846,
3.36045055271632));
#24785=CARTESIAN_POINT('Ctrl Pts',(-0.0894558149920353,0.0896584591581523,
3.36308296422493));
#24786=CARTESIAN_POINT('Ctrl Pts',(-0.112819802593213,0.0663472783512584,
3.36516929860394));
#24787=CARTESIAN_POINT('Ctrl Pts',(-0.126181642003826,0.033011291498231,
3.36725563298294));
#24788=CARTESIAN_POINT('Ctrl Pts',(-0.126482040448775,-0.000110013702131137,
3.36934196736194));
#24789=CARTESIAN_POINT('Origin',(0.,0.,3.1));
#24790=CARTESIAN_POINT('',(-0.126579711874066,8.26312290282544E-5,3.41934196736194));
#24791=CARTESIAN_POINT('',(-0.126315008613134,8.61315354740502E-5,3.40565803263806));
#24792=CARTESIAN_POINT('',(-0.12645,1.54856587752183E-17,3.1));
#24793=CARTESIAN_POINT('Ctrl Pts',(-0.126315008613134,8.61315354740502E-5,
3.40565803263806));
#24794=CARTESIAN_POINT('Ctrl Pts',(-0.12640952887744,0.0149751122618111,
3.40472331269183));
#24795=CARTESIAN_POINT('Ctrl Pts',(-0.123973978584825,0.029834173019371,
3.4037885927456));
#24796=CARTESIAN_POINT('Ctrl Pts',(-0.118870621145655,0.0437122030848606,
3.40285387279937));
#24797=CARTESIAN_POINT('Ctrl Pts',(-0.104498255487237,0.0827963011707195,
3.40022146129076));
#24798=CARTESIAN_POINT('Ctrl Pts',(-0.0689667030308244,0.114099547595362,
3.39758904978215));
#24799=CARTESIAN_POINT('Ctrl Pts',(-0.0283829362832705,0.123431722821457,
3.39495663827353));
#24800=CARTESIAN_POINT('Ctrl Pts',(0.0122008304642834,0.132763898047552,
3.39232422676492));
#24801=CARTESIAN_POINT('Ctrl Pts',(0.0578368115029788,0.120125002075099,
3.38969181525631));
#24802=CARTESIAN_POINT('Ctrl Pts',(0.0878375490289461,0.0912444313426293,
3.3870594037477));
#24803=CARTESIAN_POINT('Ctrl Pts',(0.117838286554913,0.0623638606101592,
3.38442699223909));
#24804=CARTESIAN_POINT('Ctrl Pts',(0.132203780568153,0.0172416151176717,
3.38179458073047));
#24805=CARTESIAN_POINT('Ctrl Pts',(0.124421942484303,-0.0236677311728431,
3.37916216922186));
#24806=CARTESIAN_POINT('Ctrl Pts',(0.116640104400452,-0.0645770774633583,
3.37652975771325));
#24807=CARTESIAN_POINT('Ctrl Pts',(0.0867109342195124,-0.1012735245519,
3.37389734620464));
#24808=CARTESIAN_POINT('Ctrl Pts',(0.0482017626101867,-0.117122036149449,
3.37126493469603));
#24809=CARTESIAN_POINT('Ctrl Pts',(0.00969259100086189,-0.132970547746997,
3.36863252318742));
#24810=CARTESIAN_POINT('Ctrl Pts',(-0.0373965820368482,-0.127971123853552,
3.3660001116788));
#24811=CARTESIAN_POINT('Ctrl Pts',(-0.0717195455091802,-0.104390076455735,
3.36336770017019));
#24812=CARTESIAN_POINT('Ctrl Pts',(-0.105227305247545,-0.0813691018472357,
3.36079781099281));
#24813=CARTESIAN_POINT('Ctrl Pts',(-0.126568073655319,-0.0406386849075436,
3.35822792181544));
#24814=CARTESIAN_POINT('Ctrl Pts',(-0.126649735277799,1.79833793418055E-5,
3.35565803263806));
#24815=CARTESIAN_POINT('Ctrl Pts',(-0.126482040448775,-0.000110013702131137,
3.36934196736194));
#24816=CARTESIAN_POINT('Ctrl Pts',(-0.126560666733329,-0.00877918363707953,
3.36988804449155));
#24817=CARTESIAN_POINT('Ctrl Pts',(-0.125744482172779,-0.0174336462000347,
3.37043412162116));
#24818=CARTESIAN_POINT('Ctrl Pts',(-0.123978629867097,-0.0258897947229394,
3.37098019875077));
#24819=CARTESIAN_POINT('Ctrl Pts',(-0.115466187796289,-0.0666533819220227,
3.37361261025938));
#24820=CARTESIAN_POINT('Ctrl Pts',(-0.0848853240803387,-0.102808538565874,
3.37624502176799));
#24821=CARTESIAN_POINT('Ctrl Pts',(-0.046098791601206,-0.117965603239704,
3.3788774332766));
#24822=CARTESIAN_POINT('Ctrl Pts',(-0.00731225912207339,-0.133122667913533,
3.38150984478522));
#24823=CARTESIAN_POINT('Ctrl Pts',(0.0396799421202415,-0.127281640617341,
3.38414225629383));
#24824=CARTESIAN_POINT('Ctrl Pts',(0.0735755598654084,-0.103090344478252,
3.38677466780244));
#24825=CARTESIAN_POINT('Ctrl Pts',(0.107471177610575,-0.0788990483391635,
3.38940707931105));
#24826=CARTESIAN_POINT('Ctrl Pts',(0.128270211858594,-0.0363574833571786,
3.39203949081966));
#24827=CARTESIAN_POINT('Ctrl Pts',(0.126544156121574,0.00524963674486975,
3.39467190232827));
#24828=CARTESIAN_POINT('Ctrl Pts',(0.124818100384554,0.0468567568469189,
3.39730431383689));
#24829=CARTESIAN_POINT('Ctrl Pts',(0.100566954662495,0.0875294320690312,
3.3999367253455));
#24830=CARTESIAN_POINT('Ctrl Pts',(0.0647841180740634,0.108830143717421,
3.40256913685411));
#24831=CARTESIAN_POINT('Ctrl Pts',(0.0290012814856321,0.13013085536581,
3.40520154836272));
#24832=CARTESIAN_POINT('Ctrl Pts',(-0.0183132459691715,0.132059603440478,
3.40783395987133));
#24833=CARTESIAN_POINT('Ctrl Pts',(-0.0557110968410662,0.113742058272906,
3.41046637137995));
#24834=CARTESIAN_POINT('Ctrl Pts',(-0.0931089477129611,0.0954245131053351,
3.41309878288856));
#24835=CARTESIAN_POINT('Ctrl Pts',(-0.120590122001947,0.056860674695525,
3.41573119439717));
#24836=CARTESIAN_POINT('Ctrl Pts',(-0.125697001391323,0.0155320950411155,
3.41836360590578));
#24837=CARTESIAN_POINT('Ctrl Pts',(-0.126329675264624,0.0104120382364903,
3.41868972639117));
#24838=CARTESIAN_POINT('Ctrl Pts',(-0.126618950983805,0.00524954849512788,
3.41901584687656));
#24839=CARTESIAN_POINT('Ctrl Pts',(-0.126579711874066,8.26312290282544E-5,
3.41934196736194));
#24840=CARTESIAN_POINT('Origin',(0.,0.,3.1));
#24841=CARTESIAN_POINT('',(-0.126254420230949,2.98387352259399E-5,3.46934196736194));
#24842=CARTESIAN_POINT('',(-0.126355565467006,-0.000101493988421879,3.45565803263806));
#24843=CARTESIAN_POINT('',(-0.12645,1.54856587752183E-17,3.1));
#24844=CARTESIAN_POINT('Ctrl Pts',(-0.126355565467006,-0.000101493988421879,
3.45565803263806));
#24845=CARTESIAN_POINT('Ctrl Pts',(-0.126135472102513,0.0286572548844595,
3.45385111507683));
#24846=CARTESIAN_POINT('Ctrl Pts',(-0.116386929963108,0.0575510084273647,
3.45204419751561));
#24847=CARTESIAN_POINT('Ctrl Pts',(-0.0983869251245805,0.079755841232973,
3.45023727995438));
#24848=CARTESIAN_POINT('Ctrl Pts',(-0.0721635816202546,0.112104996877157,
3.44760486844577));
#24849=CARTESIAN_POINT('Ctrl Pts',(-0.0284271866124946,0.130257467927816,
3.44497245693716));
#24850=CARTESIAN_POINT('Ctrl Pts',(0.0129959124187107,0.125984473413918,
3.44234004542855));
#24851=CARTESIAN_POINT('Ctrl Pts',(0.0544190114499162,0.121711478900021,
3.43970763391994));
#24852=CARTESIAN_POINT('Ctrl Pts',(0.0935288145045671,0.0950130188215667,
3.43707522241132));
#24853=CARTESIAN_POINT('Ctrl Pts',(0.112596275634196,0.0579918958508686,
3.43444281090271));
#24854=CARTESIAN_POINT('Ctrl Pts',(0.131663736763825,0.0209707728801704,
3.4318103993941));
#24855=CARTESIAN_POINT('Ctrl Pts',(0.130688855968432,-0.0263730129827715,
3.42917798788549));
#24856=CARTESIAN_POINT('Ctrl Pts',(0.110113561023984,-0.0625778311060434,
3.42654557637688));
#24857=CARTESIAN_POINT('Ctrl Pts',(0.0895382660795356,-0.0987826492293151,
3.42391316486827));
#24858=CARTESIAN_POINT('Ctrl Pts',(0.0493625569860325,-0.123848499612917,
3.42128075335965));
#24859=CARTESIAN_POINT('Ctrl Pts',(0.00779867036970612,-0.12641266555449,
3.41864834185104));
#24860=CARTESIAN_POINT('Ctrl Pts',(-0.0337652162466206,-0.128976831496062,
3.41601593034243));
#24861=CARTESIAN_POINT('Ctrl Pts',(-0.0767172803857706,-0.109039312995606,
3.41338351883382));
#24862=CARTESIAN_POINT('Ctrl Pts',(-0.101586723025134,-0.0756380788718395,
3.41075110732521));
#24863=CARTESIAN_POINT('Ctrl Pts',(-0.117625493100354,-0.0540969964234629,
3.40905341576282));
#24864=CARTESIAN_POINT('Ctrl Pts',(-0.126143335529839,-0.0269560826095475,
3.40735572420044));
#24865=CARTESIAN_POINT('Ctrl Pts',(-0.126315008613134,8.61315354740502E-5,
3.40565803263806));
#24866=CARTESIAN_POINT('Ctrl Pts',(-0.126579711874066,8.26312290282544E-5,
3.41934196736194));
#24867=CARTESIAN_POINT('Ctrl Pts',(-0.126302216866535,-0.0364572840554096,
3.42164825838517));
#24868=CARTESIAN_POINT('Ctrl Pts',(-0.109595120153288,-0.0732186276029635,
3.42395454940839));
#24869=CARTESIAN_POINT('Ctrl Pts',(-0.0817223269051259,-0.0967597200814019,
3.42626084043162));
#24870=CARTESIAN_POINT('Ctrl Pts',(-0.0499081885397876,-0.123629634650501,
3.42889325194023));
#24871=CARTESIAN_POINT('Ctrl Pts',(-0.00354732731934525,-0.133276142889689,
3.43152566344884));
#24872=CARTESIAN_POINT('Ctrl Pts',(0.0363442001504806,-0.121326341846207,
3.43415807495745));
#24873=CARTESIAN_POINT('Ctrl Pts',(0.0762357276203061,-0.109376540802726,
3.43679048646606));
#24874=CARTESIAN_POINT('Ctrl Pts',(0.109657921339515,-0.0758304304765741,
3.43942289797468));
#24875=CARTESIAN_POINT('Ctrl Pts',(0.121460011995994,-0.0358949527457304,
3.44205530948329));
#24876=CARTESIAN_POINT('Ctrl Pts',(0.133262102652474,0.00404052498511346,
3.4446877209919));
#24877=CARTESIAN_POINT('Ctrl Pts',(0.123444090246223,0.0503653701206494,
3.44732013250051));
#24878=CARTESIAN_POINT('Ctrl Pts',(0.0964566233770265,0.0820798513966518,
3.44995254400912));
#24879=CARTESIAN_POINT('Ctrl Pts',(0.0694691565078302,0.113794332672654,
3.45258495551774));
#24880=CARTESIAN_POINT('Ctrl Pts',(0.0253122351756883,0.130898450089123,
3.45521736702635));
#24881=CARTESIAN_POINT('Ctrl Pts',(-0.0159971621245858,0.12563865949158,
3.45784977853496));
#24882=CARTESIAN_POINT('Ctrl Pts',(-0.0573065594248602,0.120378868894038,
3.46048219004357));
#24883=CARTESIAN_POINT('Ctrl Pts',(-0.0957684326932668,0.0927551702824843,
3.46311460155218));
#24884=CARTESIAN_POINT('Ctrl Pts',(-0.113947452310361,0.0552897855612304,
3.46574701306079));
#24885=CARTESIAN_POINT('Ctrl Pts',(-0.122222848532838,0.0382349107810562,
3.46694533116118));
#24886=CARTESIAN_POINT('Ctrl Pts',(-0.126295183358791,0.0191406182899676,
3.46814364926156));
#24887=CARTESIAN_POINT('Ctrl Pts',(-0.126254420230949,2.98387352259399E-5,
3.46934196736194));
#24888=CARTESIAN_POINT('Origin',(0.,0.,3.1));
#24889=CARTESIAN_POINT('',(-0.126474550616365,-0.00011099430647141,3.51934196736194));
#24890=CARTESIAN_POINT('',(-0.12665116202208,1.34725138570783E-5,3.50565803263806));
#24891=CARTESIAN_POINT('',(-0.12645,1.54856587752183E-17,3.1));
#24892=CARTESIAN_POINT('Ctrl Pts',(-0.12665116202208,1.34725138570783E-5,
3.50565803263806));
#24893=CARTESIAN_POINT('Ctrl Pts',(-0.126652289762307,0.000752320916696393,
3.50561132897045));
#24894=CARTESIAN_POINT('Ctrl Pts',(-0.126646377467723,0.00149115078533116,
3.50556462530284));
#24895=CARTESIAN_POINT('Ctrl Pts',(-0.126633369929918,0.00222985570861129,
3.50551792163523));
#24896=CARTESIAN_POINT('Ctrl Pts',(-0.125900211401467,0.0438663147077999,
3.50288551012662));
#24897=CARTESIAN_POINT('Ctrl Pts',(-0.102626068622182,0.0851058329421116,
3.50025309861801));
#24898=CARTESIAN_POINT('Ctrl Pts',(-0.067361469104998,0.107253962401741,
3.4976206871094));
#24899=CARTESIAN_POINT('Ctrl Pts',(-0.0320968695878142,0.129402091861371,
3.49498827560079));
#24900=CARTESIAN_POINT('Ctrl Pts',(0.0151581866672683,0.132458832546319,
3.49235586409217));
#24901=CARTESIAN_POINT('Ctrl Pts',(0.0529823007948782,0.115038504173862,
3.48972345258356));
#24902=CARTESIAN_POINT('Ctrl Pts',(0.0908064149224882,0.0976181758014056,
3.48709104107495));
#24903=CARTESIAN_POINT('Ctrl Pts',(0.119199586922625,0.0597207783715444,
3.48445862956634));
#24904=CARTESIAN_POINT('Ctrl Pts',(0.125290771676778,0.0185257643337426,
3.48182621805773));
#24905=CARTESIAN_POINT('Ctrl Pts',(0.131381956430931,-0.0226692497040593,
3.47919380654911));
#24906=CARTESIAN_POINT('Ctrl Pts',(0.115171153939098,-0.0671618803498017,
3.4765613950405));
#24907=CARTESIAN_POINT('Ctrl Pts',(0.0840069606582608,-0.0947829713159226,
3.47392898353189));
#24908=CARTESIAN_POINT('Ctrl Pts',(0.0528427673774234,-0.122404062282043,
3.47129657202328));
#24909=CARTESIAN_POINT('Ctrl Pts',(0.00672518330758078,-0.133153613568543,
3.46866416051467));
#24910=CARTESIAN_POINT('Ctrl Pts',(-0.0334400173720784,-0.122158694217057,
3.46603174900606));
#24911=CARTESIAN_POINT('Ctrl Pts',(-0.0736052180517379,-0.111163774865571,
3.46339933749744));
#24912=CARTESIAN_POINT('Ctrl Pts',(-0.107818035341214,-0.0784243848761005,
3.46076692598883));
#24913=CARTESIAN_POINT('Ctrl Pts',(-0.120569297985506,-0.0387817697625104,
3.45813451448022));
#24914=CARTESIAN_POINT('Ctrl Pts',(-0.12456794717085,-0.0263503019894106,
3.45730902053283));
#24915=CARTESIAN_POINT('Ctrl Pts',(-0.126456115566329,-0.013239986655944,
3.45648352658544));
#24916=CARTESIAN_POINT('Ctrl Pts',(-0.126355565467006,-0.000101493988421879,
3.45565803263806));
#24917=CARTESIAN_POINT('Ctrl Pts',(-0.126254420230949,2.98387352259399E-5,
3.46934196736194));
#24918=CARTESIAN_POINT('Ctrl Pts',(-0.126205636746063,-0.0228410859189539,
3.47077606077017));
#24919=CARTESIAN_POINT('Ctrl Pts',(-0.120265979813939,-0.045735623724726,
3.4722101541784));
#24920=CARTESIAN_POINT('Ctrl Pts',(-0.108589648601543,-0.0651864304899691,
3.47364424758663));
#24921=CARTESIAN_POINT('Ctrl Pts',(-0.0871566593098471,-0.100890190988961,
3.47627665909524));
#24922=CARTESIAN_POINT('Ctrl Pts',(-0.0463945147606729,-0.124990641155991,
3.47890907060385));
#24923=CARTESIAN_POINT('Ctrl Pts',(-0.00478129205129982,-0.126562712056682,
3.48154148211247));
#24924=CARTESIAN_POINT('Ctrl Pts',(0.0368319306580732,-0.128134782957373,
3.48417389362108));
#24925=CARTESIAN_POINT('Ctrl Pts',(0.0792962315276452,-0.107178474591724,
3.48680630512969));
#24926=CARTESIAN_POINT('Ctrl Pts',(0.103361923070995,-0.0731935540746058,
3.4894387166383));
#24927=CARTESIAN_POINT('Ctrl Pts',(0.127427614614345,-0.0392086335574879,
3.49207112814691));
#24928=CARTESIAN_POINT('Ctrl Pts',(0.133094696831473,0.00780489911109889,
3.49470353965553));
#24929=CARTESIAN_POINT('Ctrl Pts',(0.117794195954941,0.0465350563376696,
3.49733595116414));
#24930=CARTESIAN_POINT('Ctrl Pts',(0.102493695078409,0.0852652135642405,
3.49996836267275));
#24931=CARTESIAN_POINT('Ctrl Pts',(0.0662256111082176,0.115711995348795,
3.50260077418136));
#24932=CARTESIAN_POINT('Ctrl Pts',(0.0254308018677658,0.124073556121702,
3.50523318568997));
#24933=CARTESIAN_POINT('Ctrl Pts',(-0.0153640073726858,0.13243511689461,
3.50786559719859));
#24934=CARTESIAN_POINT('Ctrl Pts',(-0.0606855418833975,0.118711456655871,
3.5104980087072));
#24935=CARTESIAN_POINT('Ctrl Pts',(-0.0899888963160071,0.0891234688732135,
3.51313042021581));
#24936=CARTESIAN_POINT('Ctrl Pts',(-0.113037365625426,0.0658511220193964,
3.51520093593118));
#24937=CARTESIAN_POINT('Ctrl Pts',(-0.12617608552629,0.032764207609907,
3.51727145164656));
#24938=CARTESIAN_POINT('Ctrl Pts',(-0.126474550616365,-0.00011099430647141,
3.51934196736194));
#24939=CARTESIAN_POINT('Origin',(0.,0.,3.1));
#24940=CARTESIAN_POINT('',(-0.126585968300139,7.56654190205152E-5,3.56934196736194));
#24941=CARTESIAN_POINT('',(-0.126320239448181,8.84447983197572E-5,3.55565803263806));
#24942=CARTESIAN_POINT('',(-0.12645,1.54856587752183E-17,3.1));
#24943=CARTESIAN_POINT('',(0.0958116152722374,0.0825211298936506,3.6));
#24944=CARTESIAN_POINT('Ctrl Pts',(-0.126585968300139,7.56654190205153E-5,
3.56934196736194));
#24945=CARTESIAN_POINT('Ctrl Pts',(-0.126314022279117,-0.0367013527487602,
3.57166407704879));
#24946=CARTESIAN_POINT('Ctrl Pts',(-0.109347743467702,-0.0736867832767084,
3.57398618673564));
#24947=CARTESIAN_POINT('Ctrl Pts',(-0.0811433985852254,-0.0972323262171825,
3.57630829642249));
#24948=CARTESIAN_POINT('Ctrl Pts',(-0.0491701276919849,-0.123924242866945,
3.57894070793111));
#24949=CARTESIAN_POINT('Ctrl Pts',(-0.00275464590947525,-0.133344354062013,
3.58157311943972));
#24950=CARTESIAN_POINT('Ctrl Pts',(0.0370665801591162,-0.121131220741312,
3.58420553094833));
#24951=CARTESIAN_POINT('Ctrl Pts',(0.0768878062277077,-0.108918087420612,
3.58683794245694));
#24952=CARTESIAN_POINT('Ctrl Pts',(0.110114776582381,-0.0750717095841421,
3.58947035396555));
#24953=CARTESIAN_POINT('Ctrl Pts',(0.121670197120012,-0.035135491975585,
3.59210276547417));
#24954=CARTESIAN_POINT('Ctrl Pts',(0.133225617657642,0.004800725632972,
3.59473517698278));
#24955=CARTESIAN_POINT('Ctrl Pts',(0.12310948837823,0.0508267830136165,
3.59736758849139));
#24956=CARTESIAN_POINT('Ctrl Pts',(0.0958116152722374,0.0825211298936506,
3.6));
#24957=CARTESIAN_POINT('',(-0.0959914412498779,0.0826500850312143,3.6));
#24958=CARTESIAN_POINT('Origin',(0.,0.,3.6));
#24959=CARTESIAN_POINT('Ctrl Pts',(-0.0959917963302685,0.0826503396631676,
3.6));
#24960=CARTESIAN_POINT('Ctrl Pts',(-0.0697118464080321,0.11301028941478,
3.59746250047314));
#24961=CARTESIAN_POINT('Ctrl Pts',(-0.0277082920252644,0.129939468632456,
3.59492500094628));
#24962=CARTESIAN_POINT('Ctrl Pts',(0.0122513409849536,0.126048715034846,
3.59238750141942));
#24963=CARTESIAN_POINT('Ctrl Pts',(0.0537056138636675,0.122012432687161,
3.58975508991081));
#24964=CARTESIAN_POINT('Ctrl Pts',(0.0929602052199782,0.095569602745952,
3.5871226784022));
#24965=CARTESIAN_POINT('Ctrl Pts',(0.112244799198078,0.058668125616663,
3.58449026689359));
#24966=CARTESIAN_POINT('Ctrl Pts',(0.131529393176178,0.0217666484873742,
3.58185785538498));
#24967=CARTESIAN_POINT('Ctrl Pts',(0.130843989776067,-0.0255934758299944,
3.57922544387636));
#24968=CARTESIAN_POINT('Ctrl Pts',(0.11048667870984,-0.0619230812123589,
3.57659303236775));
#24969=CARTESIAN_POINT('Ctrl Pts',(0.0901293676436137,-0.0982526865947235,
3.57396062085914));
#24970=CARTESIAN_POINT('Ctrl Pts',(0.0501001489112715,-0.123551773042084,
3.57132820935053));
#24971=CARTESIAN_POINT('Ctrl Pts',(0.00855140333287623,-0.126362339932449,
3.56869579784192));
#24972=CARTESIAN_POINT('Ctrl Pts',(-0.032997342245519,-0.129172906822815,
3.5660633863333));
#24973=CARTESIAN_POINT('Ctrl Pts',(-0.0760656146699672,-0.109494954156186,
3.56343097482469));
#24974=CARTESIAN_POINT('Ctrl Pts',(-0.101133339862815,-0.0762433587436205,
3.56079856331608));
#24975=CARTESIAN_POINT('Ctrl Pts',(-0.117450622825668,-0.0545989659182217,
3.55908505309007));
#24976=CARTESIAN_POINT('Ctrl Pts',(-0.126140944400475,-0.0272033229899018,
3.55737154286407));
#24977=CARTESIAN_POINT('Ctrl Pts',(-0.126320239448181,8.84447983197572E-5,
3.55565803263806));
#24978=CARTESIAN_POINT('Origin',(0.,0.,3.71042117235887));
#24979=CARTESIAN_POINT('',(-0.154532329218545,4.4775541170855E-5,2.73957882764113));
#24980=CARTESIAN_POINT('',(-0.154050519949587,1.7733618556367E-5,2.73542117235887));
#24981=CARTESIAN_POINT('',(-0.1543,1.43283619370552E-14,3.71042117235887));
#24982=CARTESIAN_POINT('',(0.03985138418574,-0.149064942821847,2.7));
#24983=CARTESIAN_POINT('Ctrl Pts',(-0.154050519949587,1.77336185563769E-5,
2.73542117235887));
#24984=CARTESIAN_POINT('Ctrl Pts',(-0.154066274679179,0.0248826176783822,
2.73414376094036));
#24985=CARTESIAN_POINT('Ctrl Pts',(-0.136678442565,0.100960491967761,2.73023393801324));
#24986=CARTESIAN_POINT('Ctrl Pts',(-0.0176337922607613,0.181151847216363,
2.72369170357751));
#24987=CARTESIAN_POINT('Ctrl Pts',(0.14217180017934,0.113903091069576,2.71579446905167));
#24988=CARTESIAN_POINT('Ctrl Pts',(0.172848115381474,-0.0569943527276058,
2.70789723452584));
#24989=CARTESIAN_POINT('Ctrl Pts',(0.0891618565332066,-0.135882161272415,
2.70263241150861));
#24990=CARTESIAN_POINT('Ctrl Pts',(0.0398513841857358,-0.149064942821848,
2.7));
#24991=CARTESIAN_POINT('',(-0.0398513841857137,-0.149064942821854,2.7));
#24992=CARTESIAN_POINT('Origin',(0.,0.,2.7));
#24993=CARTESIAN_POINT('Ctrl Pts',(-0.154532329218545,4.47755411708581E-5,
2.73957882764113));
#24994=CARTESIAN_POINT('Ctrl Pts',(-0.154541474731814,0.00247370285197769,
2.73945303065539));
#24995=CARTESIAN_POINT('Ctrl Pts',(-0.153393280968798,0.0557210645369631,
2.73669482216104));
#24996=CARTESIAN_POINT('Ctrl Pts',(-0.0921890914137533,0.156981837366664,
2.73130420215808));
#24997=CARTESIAN_POINT('Ctrl Pts',(0.081054919689294,0.163034936656946,
2.72340696763225));
#24998=CARTESIAN_POINT('Ctrl Pts',(0.180814453969382,0.0212164304176998,
2.71550973310641));
#24999=CARTESIAN_POINT('Ctrl Pts',(0.117409156055766,-0.137788854076994,
2.70770741056233));
#25000=CARTESIAN_POINT('Ctrl Pts',(0.00742265010309158,-0.161856516962739,
2.70253749952686));
#25001=CARTESIAN_POINT('Ctrl Pts',(-0.0399441884684105,-0.149319082708151,
2.7));
#25002=CARTESIAN_POINT('Origin',(0.,0.,3.71042117235887));
#25003=CARTESIAN_POINT('',(-0.154111134012939,9.12056675990702E-5,2.78957882764113));
#25004=CARTESIAN_POINT('',(-0.154375356381381,-0.000128347871137961,2.78542117235887));
#25005=CARTESIAN_POINT('',(-0.1543,1.43283619370552E-14,3.71042117235887));
#25006=CARTESIAN_POINT('Ctrl Pts',(-0.154375356381381,-0.000128347871137957,
2.78542117235887));
#25007=CARTESIAN_POINT('Ctrl Pts',(-0.154004490723256,0.0414883916240874,
2.78327156332537));
#25008=CARTESIAN_POINT('Ctrl Pts',(-0.115247407249284,0.134678118697344,
2.77848954278325));
#25009=CARTESIAN_POINT('Ctrl Pts',(0.0418557848916964,0.17717956471448,
2.77107511073252));
#25010=CARTESIAN_POINT('Ctrl Pts',(0.171243621830244,0.0618160489303277,
2.76317787620668));
#25011=CARTESIAN_POINT('Ctrl Pts',(0.145372553280857,-0.109598760687136,
2.75528064168085));
#25012=CARTESIAN_POINT('Ctrl Pts',(-0.0122890050489303,-0.181634550845065,
2.74738340715501));
#25013=CARTESIAN_POINT('Ctrl Pts',(-0.13512250192602,-0.104001863717814,
2.74076358404769));
#25014=CARTESIAN_POINT('Ctrl Pts',(-0.154033808293727,-0.0263574182340484,
2.73677617244897));
#25015=CARTESIAN_POINT('Ctrl Pts',(-0.154050519949587,1.77336185563769E-5,
2.73542117235887));
#25016=CARTESIAN_POINT('Ctrl Pts',(-0.154111134012939,9.12056675990824E-5,
2.78957882764113));
#25017=CARTESIAN_POINT('Ctrl Pts',(-0.154216904845773,0.0194969338944761,
2.7885808330404));
#25018=CARTESIAN_POINT('Ctrl Pts',(-0.141845660080373,0.0899592653630177,
2.78495042693105));
#25019=CARTESIAN_POINT('Ctrl Pts',(-0.0365555263461618,0.178349534836247,
2.7786876093131));
#25020=CARTESIAN_POINT('Ctrl Pts',(0.129354617910885,0.128110846926664,
2.77079037478726));
#25021=CARTESIAN_POINT('Ctrl Pts',(0.177988125847537,-0.0382780523762908,
2.76289314026143));
#25022=CARTESIAN_POINT('Ctrl Pts',(0.0652523050728403,-0.169960699505811,
2.75499590573559));
#25023=CARTESIAN_POINT('Ctrl Pts',(-0.10390483603623,-0.147913217635949,
2.74722446819549));
#25024=CARTESIAN_POINT('Ctrl Pts',(-0.154350096899974,-0.0483537169716228,
2.742085442164));
#25025=CARTESIAN_POINT('Ctrl Pts',(-0.154532329218545,4.47755411708581E-5,
2.73957882764113));
#25026=CARTESIAN_POINT('Origin',(0.,0.,3.71042117235887));
#25027=CARTESIAN_POINT('',(-0.154217143654561,-0.000131209131675823,2.83957882764113));
#25028=CARTESIAN_POINT('',(-0.154426485097132,0.00011404955978979,2.83542117235887));
#25029=CARTESIAN_POINT('',(-0.1543,1.43283619370552E-14,3.71042117235887));
#25030=CARTESIAN_POINT('Ctrl Pts',(-0.154426485097132,0.000114049559789811,
2.83542117235887));
#25031=CARTESIAN_POINT('Ctrl Pts',(-0.154488936846892,0.00764629898056818,
2.83503177721898));
#25032=CARTESIAN_POINT('Ctrl Pts',(-0.15057776842572,0.0660334076153961,
2.83200997057048));
#25033=CARTESIAN_POINT('Ctrl Pts',(-0.0761594594163292,0.165362226259928,
2.82635575241337));
#25034=CARTESIAN_POINT('Ctrl Pts',(0.0968288057644592,0.154172306963803,
2.81845851788754));
#25035=CARTESIAN_POINT('Ctrl Pts',(0.182029287997112,0.0032053357021354,
2.8105612833617));
#25036=CARTESIAN_POINT('Ctrl Pts',(0.102196604793212,-0.150667825661861,
2.80266404883587));
#25037=CARTESIAN_POINT('Ctrl Pts',(-0.0702903425019912,-0.167940860695529,
2.79476681431002));
#25038=CARTESIAN_POINT('Ctrl Pts',(-0.14944611336054,-0.069697339741445,
2.7890191888177));
#25039=CARTESIAN_POINT('Ctrl Pts',(-0.154458652857569,-0.00947547310228015,
2.78590397483398));
#25040=CARTESIAN_POINT('Ctrl Pts',(-0.154375356381381,-0.000128347871137957,
2.78542117235887));
#25041=CARTESIAN_POINT('Ctrl Pts',(-0.154217143654561,-0.000131209131675806,
2.83957882764113));
#25042=CARTESIAN_POINT('Ctrl Pts',(-0.153918019192818,0.0361710755121499,
2.8377086354254));
#25043=CARTESIAN_POINT('Ctrl Pts',(-0.123049963751881,0.124029060195803,
2.83320603170106));
#25044=CARTESIAN_POINT('Ctrl Pts',(0.0229951363840201,0.180599411232496,
2.82607101646811));
#25045=CARTESIAN_POINT('Ctrl Pts',(0.163793876249876,0.0794763606914083,
2.81817378194228));
#25046=CARTESIAN_POINT('Ctrl Pts',(0.1560922965942,-0.0937023067775016,
2.81027654741644));
#25047=CARTESIAN_POINT('Ctrl Pts',(0.00687287227597422,-0.181927677084725,
2.8023793128906));
#25048=CARTESIAN_POINT('Ctrl Pts',(-0.128932992743455,-0.114906920263654,
2.7954800729655));
#25049=CARTESIAN_POINT('Ctrl Pts',(-0.153937912998098,-0.0316895778160955,
2.79121324454901));
#25050=CARTESIAN_POINT('Ctrl Pts',(-0.154111134012939,9.12056675990824E-5,
2.78957882764113));
#25051=CARTESIAN_POINT('Origin',(0.,0.,3.71042117235887));
#25052=CARTESIAN_POINT('',(-0.154535784933253,3.81877733398595E-5,2.88957882764113));
#25053=CARTESIAN_POINT('',(-0.154054921884602,1.70237768407695E-5,2.88542117235887));
#25054=CARTESIAN_POINT('',(-0.1543,1.43283619370552E-14,3.71042117235887));
#25055=CARTESIAN_POINT('Ctrl Pts',(-0.154054921884602,1.70237768407841E-5,
2.88542117235887));
#25056=CARTESIAN_POINT('Ctrl Pts',(-0.154079346410273,0.0245707720672152,
2.88415957960399));
#25057=CARTESIAN_POINT('Ctrl Pts',(-0.1369997697474,0.100325734672348,2.88026557534049));
#25058=CARTESIAN_POINT('Ctrl Pts',(-0.0186809878927599,0.181096514045709,
2.87373915956839));
#25059=CARTESIAN_POINT('Ctrl Pts',(0.14142638889208,0.114645117640021,2.86584192504255));
#25060=CARTESIAN_POINT('Ctrl Pts',(0.173312464619039,-0.0557468952238434,
2.85794469051671));
#25061=CARTESIAN_POINT('Ctrl Pts',(0.0480683875166603,-0.175597144601074,
2.85004745599088));
#25062=CARTESIAN_POINT('Ctrl Pts',(-0.112431541495112,-0.138186203572753,
2.84253961660493));
#25063=CARTESIAN_POINT('Ctrl Pts',(-0.154066746922155,-0.0432736484708866,
2.8376641887276));
#25064=CARTESIAN_POINT('Ctrl Pts',(-0.154426485097132,0.000114049559789811,
2.83542117235887));
#25065=CARTESIAN_POINT('Ctrl Pts',(-0.154535784933253,3.8187773339879E-5,
2.88957882764113));
#25066=CARTESIAN_POINT('Ctrl Pts',(-0.154542902681706,0.00216158596911697,
2.88946884931902));
#25067=CARTESIAN_POINT('Ctrl Pts',(-0.153545003294962,0.0551032333888324,
2.8867264594883));
#25068=CARTESIAN_POINT('Ctrl Pts',(-0.0931239936920636,0.15643799622185,
2.88135165814895));
#25069=CARTESIAN_POINT('Ctrl Pts',(0.080081970475175,0.163498632518342,
2.87345442362313));
#25070=CARTESIAN_POINT('Ctrl Pts',(0.180683277203119,0.0223266252501708,
2.86555718909729));
#25071=CARTESIAN_POINT('Ctrl Pts',(0.11747183849698,-0.139087354145018,
2.85765995457145));
#25072=CARTESIAN_POINT('Ctrl Pts',(-0.0522430059551858,-0.174400668051551,
2.84976272004562));
#25073=CARTESIAN_POINT('Ctrl Pts',(-0.145618409602951,-0.0806790644135928,
2.84373567773551));
#25074=CARTESIAN_POINT('Ctrl Pts',(-0.154339055420526,-0.0149266411191706,
2.84034104693401));
#25075=CARTESIAN_POINT('Ctrl Pts',(-0.154217143654561,-0.000131209131675806,
2.83957882764113));
#25076=CARTESIAN_POINT('Origin',(0.,0.,3.71042117235887));
#25077=CARTESIAN_POINT('',(-0.154116825055928,9.48496454908493E-5,2.93957882764113));
#25078=CARTESIAN_POINT('',(-0.154366358871002,-0.000130096805920683,2.93542117235887));
#25079=CARTESIAN_POINT('',(-0.1543,1.43283619370552E-14,3.71042117235887));
#25080=CARTESIAN_POINT('Ctrl Pts',(-0.154366358871002,-0.000130096805920679,
2.93542117235887));
#25081=CARTESIAN_POINT('Ctrl Pts',(-0.153995797272422,0.0411865074797718,
2.93328738198899));
#25082=CARTESIAN_POINT('Ctrl Pts',(-0.115714146224304,0.134080683615333,
2.9285211801105));
#25083=CARTESIAN_POINT('Ctrl Pts',(0.0407990816336726,0.177427059877793,
2.9211225667234));
#25084=CARTESIAN_POINT('Ctrl Pts',(0.170870699467283,0.0628341523235889,
2.91322533219756));
#25085=CARTESIAN_POINT('Ctrl Pts',(0.146025941933673,-0.108726036068736,
2.90532809767173));
#25086=CARTESIAN_POINT('Ctrl Pts',(-0.0112102069433731,-0.181712019164164,
2.89743086314589));
#25087=CARTESIAN_POINT('Ctrl Pts',(-0.134787821110527,-0.104611252124613,
2.89079522137494));
#25088=CARTESIAN_POINT('Ctrl Pts',(-0.154028382735806,-0.026662535455284,
2.8867919911126));
#25089=CARTESIAN_POINT('Ctrl Pts',(-0.154054921884602,1.70237768407841E-5,
2.88542117235887));
#25090=CARTESIAN_POINT('Ctrl Pts',(-0.154116825055928,9.48496454908822E-5,
2.93957882764113));
#25091=CARTESIAN_POINT('Ctrl Pts',(-0.154225358468008,0.0191912107511692,
2.93859665170402));
#25092=CARTESIAN_POINT('Ctrl Pts',(-0.1421149984489,0.0893365787084054,
2.93498206425831));
#25093=CARTESIAN_POINT('Ctrl Pts',(-0.0376184643267171,0.178128537842515,
2.92873506530397));
#25094=CARTESIAN_POINT('Ctrl Pts',(0.128588348481182,0.128879639534425,
2.92083783077814));
#25095=CARTESIAN_POINT('Ctrl Pts',(0.178213202383553,-0.0372153106656781,
2.9129405962523));
#25096=CARTESIAN_POINT('Ctrl Pts',(0.0662647529343645,-0.169569771398652,
2.90504336172647));
#25097=CARTESIAN_POINT('Ctrl Pts',(-0.10336559476711,-0.148485092132862,
2.89725610552274));
#25098=CARTESIAN_POINT('Ctrl Pts',(-0.154372534171041,-0.0486635015632469,
2.89210126082763));
#25099=CARTESIAN_POINT('Ctrl Pts',(-0.154535784933253,3.8187773339879E-5,
2.88957882764113));
#25100=CARTESIAN_POINT('Origin',(0.,0.,3.71042117235887));
#25101=CARTESIAN_POINT('',(-0.154208836002914,-0.000129626704909153,2.98957882764113));
#25102=CARTESIAN_POINT('',(-0.154434696759477,0.000111004303427491,2.98542117235887));
#25103=CARTESIAN_POINT('',(-0.1543,1.43283619370552E-14,3.71042117235887));
#25104=CARTESIAN_POINT('Ctrl Pts',(-0.154434696759477,0.000111004303427509,
2.98542117235887));
#25105=CARTESIAN_POINT('Ctrl Pts',(-0.15449350107168,0.00733626390374423,
2.98504759588261));
#25106=CARTESIAN_POINT('Ctrl Pts',(-0.150762340620084,0.0654133961639385,
2.98204160789773));
#25107=CARTESIAN_POINT('Ctrl Pts',(-0.0771442428547834,0.164905101290741,
2.97640320840425));
#25108=CARTESIAN_POINT('Ctrl Pts',(0.0959076962473017,0.15474702077238,
2.96850597387841));
#25109=CARTESIAN_POINT('Ctrl Pts',(0.182006911912947,0.00429076371209153,
2.96060873935257));
#25110=CARTESIAN_POINT('Ctrl Pts',(0.103093336173269,-0.150055625266004,
2.95271150482674));
#25111=CARTESIAN_POINT('Ctrl Pts',(-0.069287674394006,-0.168357194128057,
2.9448142703009));
#25112=CARTESIAN_POINT('Ctrl Pts',(-0.14924717784082,-0.0703180680940833,
2.93905082614495));
#25113=CARTESIAN_POINT('Ctrl Pts',(-0.154452951185252,-0.00978490290509501,
2.9359197934976));
#25114=CARTESIAN_POINT('Ctrl Pts',(-0.154366358871002,-0.000130096805920679,
2.93542117235887));
#25115=CARTESIAN_POINT('Ctrl Pts',(-0.154208836002914,-0.00012962670490916,
2.98957882764113));
#25116=CARTESIAN_POINT('Ctrl Pts',(-0.15391701905173,0.0358705210125992,
2.98772445408903));
#25117=CARTESIAN_POINT('Ctrl Pts',(-0.123464382903156,0.123420397725162,
2.98323766902831));
#25118=CARTESIAN_POINT('Ctrl Pts',(0.0219177299165732,0.180733333857582,
2.97611847245899));
#25119=CARTESIAN_POINT('Ctrl Pts',(0.163317009898163,0.0804517192475515,
2.96822123793315));
#25120=CARTESIAN_POINT('Ctrl Pts',(0.156648310460303,-0.0927697778475837,
2.96032400340732));
#25121=CARTESIAN_POINT('Ctrl Pts',(0.00795766962277319,-0.181883480135435,
2.95242676888148));
#25122=CARTESIAN_POINT('Ctrl Pts',(-0.128557747147415,-0.11552191978543,
2.94551171029275));
#25123=CARTESIAN_POINT('Ctrl Pts',(-0.1539344690334,-0.0319905366812824,
2.94122906321263));
#25124=CARTESIAN_POINT('Ctrl Pts',(-0.154116825055928,9.48496454908822E-5,
2.93957882764113));
#25125=CARTESIAN_POINT('Origin',(0.,0.,3.71042117235887));
#25126=CARTESIAN_POINT('',(-0.154538871978598,3.2832780837988E-5,3.03957882764113));
#25127=CARTESIAN_POINT('',(-0.154056089165245,2.19184202627989E-5,3.03542117235887));
#25128=CARTESIAN_POINT('',(-0.1543,1.43283619370552E-14,3.71042117235887));
#25129=CARTESIAN_POINT('Ctrl Pts',(-0.154056089165245,2.19184202628134E-5,
3.03542117235887));
#25130=CARTESIAN_POINT('Ctrl Pts',(-0.154087155299894,0.0242673368387721,
3.03417539826761));
#25131=CARTESIAN_POINT('Ctrl Pts',(-0.137310014833352,0.0997044362362006,
3.03029721266774));
#25132=CARTESIAN_POINT('Ctrl Pts',(-0.0197606177252597,0.180981890321858,
3.02378661555926));
#25133=CARTESIAN_POINT('Ctrl Pts',(0.140740192743497,0.115486470133437,
3.01588938103343));
#25134=CARTESIAN_POINT('Ctrl Pts',(0.173641826766224,-0.0547123627222005,
3.00799214650759));
#25135=CARTESIAN_POINT('Ctrl Pts',(0.0491147003187017,-0.175307366787479,
3.00009491198175));
#25136=CARTESIAN_POINT('Ctrl Pts',(-0.11194410582055,-0.138777425062269,
2.99257125393218));
#25137=CARTESIAN_POINT('Ctrl Pts',(-0.15407913571938,-0.0435766220328422,
2.98768000739122));
#25138=CARTESIAN_POINT('Ctrl Pts',(-0.154434696759477,0.000111004303427509,
2.98542117235887));
#25139=CARTESIAN_POINT('Ctrl Pts',(-0.154538871978598,3.28327808380407E-5,
3.03957882764113));
#25140=CARTESIAN_POINT('Ctrl Pts',(-0.154544182685759,0.00185071603346938,
3.03948466798264));
#25141=CARTESIAN_POINT('Ctrl Pts',(-0.153694834634547,0.0544858891421056,
3.03675809681555));
#25142=CARTESIAN_POINT('Ctrl Pts',(-0.0940552495850459,0.15587987322763,
3.03139911413983));
#25143=CARTESIAN_POINT('Ctrl Pts',(0.0791055288760802,0.163973290975094,
3.02350187961401));
#25144=CARTESIAN_POINT('Ctrl Pts',(0.180546920428939,0.0234037256776295,
3.01560464508816));
#25145=CARTESIAN_POINT('Ctrl Pts',(0.118299191571216,-0.138384342053441,
3.00770741056233));
#25146=CARTESIAN_POINT('Ctrl Pts',(-0.0512020455023775,-0.174709116500372,
2.99981017603649));
#25147=CARTESIAN_POINT('Ctrl Pts',(-0.145381230907426,-0.0813015016053826,
2.99376731506276));
#25148=CARTESIAN_POINT('Ctrl Pts',(-0.154331273396456,-0.0152341784994835,
2.99035686559764));
#25149=CARTESIAN_POINT('Ctrl Pts',(-0.154208836002914,-0.00012962670490916,
2.98957882764113));
#25150=CARTESIAN_POINT('Origin',(0.,0.,3.71042117235887));
#25151=CARTESIAN_POINT('',(-0.154122750472518,9.83954699399631E-5,3.08957882764113));
#25152=CARTESIAN_POINT('',(-0.154357314101369,-0.000131672715837502,3.08542117235887));
#25153=CARTESIAN_POINT('',(-0.1543,1.43283619370552E-14,3.71042117235887));
#25154=CARTESIAN_POINT('Ctrl Pts',(-0.154357314101369,-0.000131672715837496,
3.08542117235887));
#25155=CARTESIAN_POINT('Ctrl Pts',(-0.153987553769485,0.0408848376338906,
3.08330320065262));
#25156=CARTESIAN_POINT('Ctrl Pts',(-0.11617759776856,0.133482913719063,
3.07855281743775));
#25157=CARTESIAN_POINT('Ctrl Pts',(0.039740276922879,0.17766720864428,3.07117002271427));
#25158=CARTESIAN_POINT('Ctrl Pts',(0.170492952144154,0.0638520156810144,
3.06327278818844));
#25159=CARTESIAN_POINT('Ctrl Pts',(0.146671728755708,-0.107853282848364,
3.0553755536626));
#25160=CARTESIAN_POINT('Ctrl Pts',(-0.0101263751692898,-0.181775639631079,
3.04747831913677));
#25161=CARTESIAN_POINT('Ctrl Pts',(-0.134457266065241,-0.105231153897523,
3.04082685870219));
#25162=CARTESIAN_POINT('Ctrl Pts',(-0.154021510291741,-0.026965000487735,
3.03680780977622));
#25163=CARTESIAN_POINT('Ctrl Pts',(-0.154056089165245,2.19184202628134E-5,
3.03542117235887));
#25164=CARTESIAN_POINT('Ctrl Pts',(-0.154122750472518,9.83954699399839E-5,
3.08957882764113));
#25165=CARTESIAN_POINT('Ctrl Pts',(-0.154233799032612,0.0188853799021587,
3.08861247036765));
#25166=CARTESIAN_POINT('Ctrl Pts',(-0.142381965748736,0.0887139061579003,
3.08501370158555));
#25167=CARTESIAN_POINT('Ctrl Pts',(-0.0386800578824722,0.177901034213339,
3.07878252129485));
#25168=CARTESIAN_POINT('Ctrl Pts',(0.127817493356429,0.129644179368171,
3.07088528676902));
#25169=CARTESIAN_POINT('Ctrl Pts',(0.178431965499368,-0.0361518815554529,
3.06298805224317));
#25170=CARTESIAN_POINT('Ctrl Pts',(0.0672747972491473,-0.169171588947593,
3.05509081771735));
#25171=CARTESIAN_POINT('Ctrl Pts',(-0.102823100152332,-0.149058093692613,
3.04728774284999));
#25172=CARTESIAN_POINT('Ctrl Pts',(-0.154395711813265,-0.0489716517674636,
3.04211707949126));
#25173=CARTESIAN_POINT('Ctrl Pts',(-0.154538871978598,3.28327808380407E-5,
3.03957882764113));
#25174=CARTESIAN_POINT('Origin',(0.,0.,3.71042117235887));
#25175=CARTESIAN_POINT('',(-0.154200664638475,-0.000127870236170058,3.13957882764113));
#25176=CARTESIAN_POINT('',(-0.154442743231392,0.000107782702043065,3.13542117235887));
#25177=CARTESIAN_POINT('',(-0.1543,1.43283619370552E-14,3.71042117235887));
#25178=CARTESIAN_POINT('Ctrl Pts',(-0.154442743231391,0.000107782702043087,
3.13542117235887));
#25179=CARTESIAN_POINT('Ctrl Pts',(-0.154497895338046,0.00702615569019676,
3.13506341454624));
#25180=CARTESIAN_POINT('Ctrl Pts',(-0.150944880930953,0.0647935208243374,
3.13207324522499));
#25181=CARTESIAN_POINT('Ctrl Pts',(-0.0781262761399388,0.164442122383114,
3.12645066439512));
#25182=CARTESIAN_POINT('Ctrl Pts',(0.0949831631341886,0.155316210867962,
3.11855342986929));
#25183=CARTESIAN_POINT('Ctrl Pts',(0.181978087741923,0.00537607841744088,
3.11065619534345));
#25184=CARTESIAN_POINT('Ctrl Pts',(0.10398635378076,-0.149438164016893,
3.10275896081762));
#25185=CARTESIAN_POINT('Ctrl Pts',(-0.0682824508977375,-0.168767394767933,
3.09486172629178));
#25186=CARTESIAN_POINT('Ctrl Pts',(-0.14904624696594,-0.0709390773474446,
3.0890824634722));
#25187=CARTESIAN_POINT('Ctrl Pts',(-0.154447126175577,-0.0100942824218163,
3.08593561216123));
#25188=CARTESIAN_POINT('Ctrl Pts',(-0.154357314101369,-0.000131672715837496,
3.08542117235887));
#25189=CARTESIAN_POINT('Ctrl Pts',(-0.154200664638475,-0.000127870236170063,
3.13957882764113));
#25190=CARTESIAN_POINT('Ctrl Pts',(-0.153916387321455,0.03556997377657,
3.13774027275265));
#25191=CARTESIAN_POINT('Ctrl Pts',(-0.123875930184563,0.122811200111113,
3.13326930635556));
#25192=CARTESIAN_POINT('Ctrl Pts',(0.0208395441149821,0.180860825645154,
3.12616592844986));
#25193=CARTESIAN_POINT('Ctrl Pts',(0.162834335224968,0.0814242232005321,
3.11826869392403));
#25194=CARTESIAN_POINT('Ctrl Pts',(0.157198753896076,-0.0918339622660831,
3.1103714593982));
#25195=CARTESIAN_POINT('Ctrl Pts',(0.00904218304404205,-0.181832790711041,
3.10247422487235));
#25196=CARTESIAN_POINT('Ctrl Pts',(-0.128179738775568,-0.116136573115574,
3.09554334762));
#25197=CARTESIAN_POINT('Ctrl Pts',(-0.153931296515552,-0.0322914212547928,
3.09124488187626));
#25198=CARTESIAN_POINT('Ctrl Pts',(-0.154122750472518,9.83954699399839E-5,
3.08957882764113));
#25199=CARTESIAN_POINT('Origin',(0.,0.,3.71042117235887));
#25200=CARTESIAN_POINT('',(-0.154541524340359,2.74150270591633E-5,3.18957882764113));
#25201=CARTESIAN_POINT('',(-0.154057549710717,2.67855146112065E-5,3.18542117235887));
#25202=CARTESIAN_POINT('',(-0.1543,1.43283619370552E-14,3.71042117235887));
#25203=CARTESIAN_POINT('Ctrl Pts',(-0.154057549710717,2.67855146112127E-5,
3.18542117235887));
#25204=CARTESIAN_POINT('Ctrl Pts',(-0.154095052553054,0.0239637717781011,
3.18419121693124));
#25205=CARTESIAN_POINT('Ctrl Pts',(-0.137617732079011,0.0990829983563936,
3.18032884999499));
#25206=CARTESIAN_POINT('Ctrl Pts',(-0.0208395446762738,0.180860830516292,
3.17383407155014));
#25207=CARTESIAN_POINT('Ctrl Pts',(0.140048991174337,0.116323715159066,
3.1659368370243));
#25208=CARTESIAN_POINT('Ctrl Pts',(0.173965014144346,-0.0536758837012937,
3.15803960249847));
#25209=CARTESIAN_POINT('Ctrl Pts',(0.050159265511441,-0.175011355976434,
3.15014236797263));
#25210=CARTESIAN_POINT('Ctrl Pts',(-0.111453603442084,-0.139367747346172,
3.14260289125943));
#25211=CARTESIAN_POINT('Ctrl Pts',(-0.154092081585972,-0.0438798036810342,
3.13769582605485));
#25212=CARTESIAN_POINT('Ctrl Pts',(-0.154442743231391,0.000107782702043087,
3.13542117235887));
#25213=CARTESIAN_POINT('Ctrl Pts',(-0.154541524340359,2.74150270592019E-5,
3.18957882764113));
#25214=CARTESIAN_POINT('Ctrl Pts',(-0.154545265409953,0.0015398273092893,
3.18950048664627));
#25215=CARTESIAN_POINT('Ctrl Pts',(-0.153842769766794,0.0538687068697594,
3.1867897341428));
#25216=CARTESIAN_POINT('Ctrl Pts',(-0.0949831605760139,0.155316206684809,
3.18144657013072));
#25217=CARTESIAN_POINT('Ctrl Pts',(0.0781262740357409,0.164442117954189,
3.17354933560488));
#25218=CARTESIAN_POINT('Ctrl Pts',(0.180404142828019,0.0244799939226929,
3.16565210107904));
#25219=CARTESIAN_POINT('Ctrl Pts',(0.119122337560023,-0.137676408822293,
3.15775486655321));
#25220=CARTESIAN_POINT('Ctrl Pts',(-0.0501592641604809,-0.175011351262844,
3.14985763202737));
#25221=CARTESIAN_POINT('Ctrl Pts',(-0.145141798308845,-0.081923988470417,
3.14379895239001));
#25222=CARTESIAN_POINT('Ctrl Pts',(-0.15432341073188,-0.0155415899851509,
3.14037268426126));
#25223=CARTESIAN_POINT('Ctrl Pts',(-0.154200664638475,-0.000127870236170063,
3.13957882764113));
#25224=CARTESIAN_POINT('Origin',(0.,0.,3.71042117235887));
#25225=CARTESIAN_POINT('',(-0.154128903346263,0.000101814369117867,3.23957882764113));
#25226=CARTESIAN_POINT('',(-0.15434822268538,-0.000133055250486845,3.23542117235887));
#25227=CARTESIAN_POINT('',(-0.1543,1.43283619370552E-14,3.71042117235887));
#25228=CARTESIAN_POINT('Ctrl Pts',(-0.15434822268538,-0.00013305525048684,
3.23542117235887));
#25229=CARTESIAN_POINT('Ctrl Pts',(-0.153979802923996,0.0405832940781535,
3.23331901931624));
#25230=CARTESIAN_POINT('Ctrl Pts',(-0.116638046803031,0.132884381239301,
3.228584454765));
#25231=CARTESIAN_POINT('Ctrl Pts',(0.0386800589242284,0.177901039004767,
3.22121747870515));
#25232=CARTESIAN_POINT('Ctrl Pts',(0.170109141545278,0.0648676082500797,
3.21332024417931));
#25233=CARTESIAN_POINT('Ctrl Pts',(0.147312299474883,-0.106976694007524,
3.20542300965349));
#25234=CARTESIAN_POINT('Ctrl Pts',(-0.00904218328755787,-0.18183279560836,
3.19752577512764));
#25235=CARTESIAN_POINT('Ctrl Pts',(-0.134124100441736,-0.105850839905797,
3.19085849602944));
#25236=CARTESIAN_POINT('Ctrl Pts',(-0.154014787112897,-0.0272673514852388,
3.18682362843985));
#25237=CARTESIAN_POINT('Ctrl Pts',(-0.154057549710717,2.67855146112127E-5,
3.18542117235887));
#25238=CARTESIAN_POINT('Ctrl Pts',(-0.154128903346263,0.000101814369117853,
3.23957882764113));
#25239=CARTESIAN_POINT('Ctrl Pts',(-0.15424221981892,0.0185794122284465,
3.23862828903127));
#25240=CARTESIAN_POINT('Ctrl Pts',(-0.142646569905461,0.0880912185498955,
3.23504533891281));
#25241=CARTESIAN_POINT('Ctrl Pts',(-0.0397402758525677,0.177667203859151,
3.22882997728572));
#25242=CARTESIAN_POINT('Ctrl Pts',(0.127042092635782,0.130404108641901,
3.22093274275989));
#25243=CARTESIAN_POINT('Ctrl Pts',(0.178644383007786,-0.0350871667669908,
3.21303550823405));
#25244=CARTESIAN_POINT('Ctrl Pts',(0.0682824490586963,-0.1687673902225,
3.20513827370822));
#25245=CARTESIAN_POINT('Ctrl Pts',(-0.102277435139451,-0.149629907004419,
3.19731938017724));
#25246=CARTESIAN_POINT('Ctrl Pts',(-0.154419558113643,-0.0492801999911546,
3.19213289815488));
#25247=CARTESIAN_POINT('Ctrl Pts',(-0.154541524340359,2.74150270592019E-5,
3.18957882764113));
#25248=CARTESIAN_POINT('Origin',(0.,0.,3.71042117235887));
#25249=CARTESIAN_POINT('',(-0.154192638571573,-0.000125942848695916,3.28957882764113));
#25250=CARTESIAN_POINT('',(-0.154450609193756,0.000104390085258889,3.28542117235887));
#25251=CARTESIAN_POINT('',(-0.1543,1.43283619370552E-14,3.71042117235887));
#25252=CARTESIAN_POINT('Ctrl Pts',(-0.154450609193756,0.000104390085258887,
3.28542117235887));
#25253=CARTESIAN_POINT('Ctrl Pts',(-0.154502116257734,0.0067159788236037,
3.28507923320986));
#25254=CARTESIAN_POINT('Ctrl Pts',(-0.151125396911172,0.064173784678776,
3.28210488255223));
#25255=CARTESIAN_POINT('Ctrl Pts',(-0.0791055310066521,0.163973295391393,
3.27649812038601));
#25256=CARTESIAN_POINT('Ctrl Pts',(0.0940552521182287,0.155879877425964,
3.26860088586016));
#25257=CARTESIAN_POINT('Ctrl Pts',(0.181942791852133,0.00646120193221371,
3.26070365133433));
#25258=CARTESIAN_POINT('Ctrl Pts',(0.104875673303493,-0.148815388271832,
3.25280641680849));
#25259=CARTESIAN_POINT('Ctrl Pts',(-0.067274799061048,-0.169171593503912,
3.24490918228266));
#25260=CARTESIAN_POINT('Ctrl Pts',(-0.148843209204449,-0.0715602003700874,
3.23911410079945));
#25261=CARTESIAN_POINT('Ctrl Pts',(-0.154441154880871,-0.0104035676716175,
3.23595143082485));
#25262=CARTESIAN_POINT('Ctrl Pts',(-0.15434822268538,-0.00013305525048684,
3.23542117235887));
#25263=CARTESIAN_POINT('Ctrl Pts',(-0.154192638571573,-0.000125942848695916,
3.28957882764113));
#25264=CARTESIAN_POINT('Ctrl Pts',(-0.153916116413885,0.0352694274746551,
3.28775609141628));
#25265=CARTESIAN_POINT('Ctrl Pts',(-0.124284613860796,0.122201478629219,
3.28330094368282));
#25266=CARTESIAN_POINT('Ctrl Pts',(0.0197606171930289,0.18098188544746,
3.27621338444074));
#25267=CARTESIAN_POINT('Ctrl Pts',(0.162345869645737,0.0823938314495476,
3.26831614991491));
#25268=CARTESIAN_POINT('Ctrl Pts',(0.157743606844976,-0.0908948807772195,
3.26041891538907));
#25269=CARTESIAN_POINT('Ctrl Pts',(0.0101263748965706,-0.181775634735301,
3.25252168086324));
#25270=CARTESIAN_POINT('Ctrl Pts',(-0.127798960265965,-0.1167508316284,
3.24557498494725));
#25271=CARTESIAN_POINT('Ctrl Pts',(-0.153928402385683,-0.0325922506078629,
3.24126070053988));
#25272=CARTESIAN_POINT('Ctrl Pts',(-0.154128903346263,0.000101814369117853,
3.23957882764113));
#25273=CARTESIAN_POINT('Origin',(0.,0.,3.71042117235887));
#25274=CARTESIAN_POINT('',(-0.154543726005254,2.19441315424396E-5,3.33957882764113));
#25275=CARTESIAN_POINT('',(-0.154059302102979,3.16189515402649E-5,3.33542117235887));
#25276=CARTESIAN_POINT('',(-0.1543,1.43283619370552E-14,3.71042117235887));
#25277=CARTESIAN_POINT('Ctrl Pts',(-0.154059302102979,3.16189515402656E-5,
3.33542117235887));
#25278=CARTESIAN_POINT('Ctrl Pts',(-0.15410303154311,0.0236600756904899,
3.33420703559487));
#25279=CARTESIAN_POINT('Ctrl Pts',(-0.137922930779561,0.0984614290803482,
3.33036048732225));
#25280=CARTESIAN_POINT('Ctrl Pts',(-0.0219177305069036,0.180733338725286,
3.32388152754101));
#25281=CARTESIAN_POINT('Ctrl Pts',(0.139352809018331,0.117156823343995,
3.31598429301518));
#25282=CARTESIAN_POINT('Ctrl Pts',(0.174282014774141,-0.0526374957955154,
3.30808705848934));
#25283=CARTESIAN_POINT('Ctrl Pts',(0.0512020468814229,-0.174709121205821,
3.3001898239635));
#25284=CARTESIAN_POINT('Ctrl Pts',(-0.110960029365619,-0.139957157472604,
3.29263452858669));
#25285=CARTESIAN_POINT('Ctrl Pts',(-0.154105590184654,-0.0441832011483282,
3.28771164471847));
#25286=CARTESIAN_POINT('Ctrl Pts',(-0.154450609193756,0.000104390085258887,
3.28542117235887));
#25287=CARTESIAN_POINT('Ctrl Pts',(-0.154543726005254,2.19441315424298E-5,
3.33957882764113));
#25288=CARTESIAN_POINT('Ctrl Pts',(-0.154546150302478,0.00122892294348618,
3.33951630530989));
#25289=CARTESIAN_POINT('Ctrl Pts',(-0.153988815888461,0.0532516871969489,
3.33682137147005));
#25290=CARTESIAN_POINT('Ctrl Pts',(-0.0959076936642258,0.154747016604558,
3.33149402612159));
#25291=CARTESIAN_POINT('Ctrl Pts',(0.0771442407770374,0.164905096849345,
3.32359679159575));
#25292=CARTESIAN_POINT('Ctrl Pts',(0.180254949482897,0.0255553915814562,
3.31569955706992));
#25293=CARTESIAN_POINT('Ctrl Pts',(0.119941247180243,-0.13696357938087,
3.30780232254408));
#25294=CARTESIAN_POINT('Ctrl Pts',(-0.0491146989958762,-0.175307362065916,
3.29990508801825));
#25295=CARTESIAN_POINT('Ctrl Pts',(-0.144900102757682,-0.0825465196247692,
3.29383058971726));
#25296=CARTESIAN_POINT('Ctrl Pts',(-0.154315472118983,-0.0158488741865795,
3.29038850292489));
#25297=CARTESIAN_POINT('Ctrl Pts',(-0.154192638571573,-0.000125942848695916,
3.28957882764113));
#25298=CARTESIAN_POINT('Origin',(0.,0.,3.71042117235887));
#25299=CARTESIAN_POINT('',(-0.15413527741405,0.000105101588974824,3.38957882764113));
#25300=CARTESIAN_POINT('',(-0.15433909720242,-0.000134243687139869,3.38542117235887));
#25301=CARTESIAN_POINT('',(-0.1543,1.43283619370552E-14,3.71042117235887));
#25302=CARTESIAN_POINT('Ctrl Pts',(-0.15433909720242,-0.000134243687139867,
3.38542117235887));
#25303=CARTESIAN_POINT('Ctrl Pts',(-0.153972537455045,0.0402818685502336,
3.38333483797987));
#25304=CARTESIAN_POINT('Ctrl Pts',(-0.117095500692927,0.132285100657941,
3.37861609209226));
#25305=CARTESIAN_POINT('Ctrl Pts',(0.0376184653398806,0.178128542640067,
3.37126493469602));
#25306=CARTESIAN_POINT('Ctrl Pts',(0.169719281325138,0.0658808939206553,
3.36336770017019));
#25307=CARTESIAN_POINT('Ctrl Pts',(0.14794763130091,-0.10609630073556,3.35547046564435));
#25308=CARTESIAN_POINT('Ctrl Pts',(-0.00795766983708003,-0.181883485034118,
3.34757323111852));
#25309=CARTESIAN_POINT('Ctrl Pts',(-0.133788315045723,-0.106470301039161,
3.34089013335669));
#25310=CARTESIAN_POINT('Ctrl Pts',(-0.154008220246,-0.0275695907640756,
3.33683944710348));
#25311=CARTESIAN_POINT('Ctrl Pts',(-0.154059302102979,3.16189515402656E-5,
3.33542117235887));
#25312=CARTESIAN_POINT('Ctrl Pts',(-0.15413527741405,0.000105101588974825,
3.38957882764113));
#25313=CARTESIAN_POINT('Ctrl Pts',(-0.154250615308729,0.0182733082008614,
3.3886441076949));
#25314=CARTESIAN_POINT('Ctrl Pts',(-0.142908820182152,0.0874685218643051,
3.38507697624006));
#25315=CARTESIAN_POINT('Ctrl Pts',(-0.0407990805348497,0.177427055099143,
3.3788774332766));
#25316=CARTESIAN_POINT('Ctrl Pts',(0.126262173896246,0.131159400329288,
3.37098019875077));
#25317=CARTESIAN_POINT('Ctrl Pts',(0.178850447353964,-0.0340212041663437,
3.36308296422493));
#25318=CARTESIAN_POINT('Ctrl Pts',(0.0692876725278909,-0.168357189593675,
3.3551857296991));
#25319=CARTESIAN_POINT('Ctrl Pts',(-0.101728594599068,-0.150200514568663,
3.3473510175045));
#25320=CARTESIAN_POINT('Ctrl Pts',(-0.15444407880598,-0.0495891584122831,
3.3421487168185));
#25321=CARTESIAN_POINT('Ctrl Pts',(-0.154543726005254,2.19441315424298E-5,
3.33957882764113));
#25322=CARTESIAN_POINT('Origin',(0.,0.,3.71042117235887));
#25323=CARTESIAN_POINT('',(-0.154184766718537,-0.000123847547745311,3.43957882764113));
#25324=CARTESIAN_POINT('',(-0.154458280286029,0.000100830356962909,3.43542117235887));
#25325=CARTESIAN_POINT('',(-0.1543,1.43283619370552E-14,3.71042117235887));
#25326=CARTESIAN_POINT('Ctrl Pts',(-0.154458280286029,0.000100830356962935,
3.43542117235887));
#25327=CARTESIAN_POINT('Ctrl Pts',(-0.154506161619621,0.00640573612334919,
3.43509505187348));
#25328=CARTESIAN_POINT('Ctrl Pts',(-0.151303896650316,0.0635541898545394,
3.43213651987949));
#25329=CARTESIAN_POINT('Ctrl Pts',(-0.0800819726320239,0.163498636922,3.42654557637688));
#25330=CARTESIAN_POINT('Ctrl Pts',(0.0931239962001525,0.156438000435139,
3.41864834185104));
#25331=CARTESIAN_POINT('Ctrl Pts',(0.181901025498224,0.00754609564814438,
3.41075110732521));
#25332=CARTESIAN_POINT('Ctrl Pts',(0.10576126311461,-0.148187320169658,
3.40285387279937));
#25333=CARTESIAN_POINT('Ctrl Pts',(-0.0662647547190597,-0.169569775965683,
3.39495663827354));
#25334=CARTESIAN_POINT('Ctrl Pts',(-0.148638055997427,-0.0721814340714305,
3.3891457381267));
#25335=CARTESIAN_POINT('Ctrl Pts',(-0.154435040545295,-0.0107127563084332,
3.38596724948848));
#25336=CARTESIAN_POINT('Ctrl Pts',(-0.15433909720242,-0.000134243687139867,
3.38542117235887));
#25337=CARTESIAN_POINT('Ctrl Pts',(-0.154184766718538,-0.000123847547745311,
3.43957882764113));
#25338=CARTESIAN_POINT('Ctrl Pts',(-0.153916198856604,0.0349688764624186,
3.4377719100799));
#25339=CARTESIAN_POINT('Ctrl Pts',(-0.124690442079412,0.121591245361209,
3.43333258101007));
#25340=CARTESIAN_POINT('Ctrl Pts',(0.0186809873893989,0.181096509168673,
3.42626084043161));
#25341=CARTESIAN_POINT('Ctrl Pts',(0.161851630600137,0.0833605094034181,
3.41836360590578));
#25342=CARTESIAN_POINT('Ctrl Pts',(0.158282849894819,-0.0899525667211824,
3.41046637137994));
#25343=CARTESIAN_POINT('Ctrl Pts',(0.0112102066414966,-0.181712014270169,
3.40256913685411));
#25344=CARTESIAN_POINT('Ctrl Pts',(-0.127415402859048,-0.117364684067358,
3.3956066222745));
#25345=CARTESIAN_POINT('Ctrl Pts',(-0.153925794165715,-0.032893029234098,
3.39127651920351));
#25346=CARTESIAN_POINT('Ctrl Pts',(-0.15413527741405,0.000105101588974825,
3.38957882764113));
#25347=CARTESIAN_POINT('Origin',(0.,0.,3.71042117235887));
#25348=CARTESIAN_POINT('',(-0.154545466983052,1.64397697926255E-5,3.48957882764113));
#25349=CARTESIAN_POINT('',(-0.154061344734167,3.6410572125671E-5,3.48542117235887));
#25350=CARTESIAN_POINT('',(-0.1543,1.43283619370552E-14,3.71042117235887));
#25351=CARTESIAN_POINT('Ctrl Pts',(-0.154061344734167,3.64105721256669E-5,
3.48542117235887));
#25352=CARTESIAN_POINT('Ctrl Pts',(-0.154111085743468,0.0233562467547802,
3.48422285425849));
#25353=CARTESIAN_POINT('Ctrl Pts',(-0.13822562008929,0.0978397409961887,
3.48039212464949));
#25354=CARTESIAN_POINT('Ctrl Pts',(-0.0229951370022999,0.180599416102118,
3.47392898353189));
#25355=CARTESIAN_POINT('Ctrl Pts',(0.138651671100891,0.117985766817156,
3.46603174900605));
#25356=CARTESIAN_POINT('Ctrl Pts',(0.174592817347261,-0.0515972368462645,
3.45813451448022));
#25357=CARTESIAN_POINT('Ctrl Pts',(0.0522430073621133,-0.174400672749591,
3.45023727995438));
#25358=CARTESIAN_POINT('Ctrl Pts',(-0.110463377019167,-0.140545639944236,
3.44266616591394));
#25359=CARTESIAN_POINT('Ctrl Pts',(-0.15411966834722,-0.0444868242763973,
3.4377274633821));
#25360=CARTESIAN_POINT('Ctrl Pts',(-0.154458280286029,0.000100830356962935,
3.43542117235887));
#25361=CARTESIAN_POINT('Ctrl Pts',(-0.154545466983052,1.64397697926493E-5,
3.48957882764113));
#25362=CARTESIAN_POINT('Ctrl Pts',(-0.154546843102601,0.000918015954509084,
3.48953212397352));
#25363=CARTESIAN_POINT('Ctrl Pts',(-0.154132992535152,0.0526348504359433,
3.4868530087973));
#25364=CARTESIAN_POINT('Ctrl Pts',(-0.0968288031440013,0.15417230277993,
3.48154148211247));
#25365=CARTESIAN_POINT('Ctrl Pts',(0.0761594573579975,0.165362221823523,
3.47364424758663));
#25366=CARTESIAN_POINT('Ctrl Pts',(0.180099349163956,0.0266298748857393,
3.46574701306079));
#25367=CARTESIAN_POINT('Ctrl Pts',(0.120755889508211,-0.136245876208876,
3.45784977853496));
#25368=CARTESIAN_POINT('Ctrl Pts',(-0.0480683862207756,-0.175597139874519,
3.44995254400912));
#25369=CARTESIAN_POINT('Ctrl Pts',(-0.144656135320296,-0.0831690899066176,
3.44386222704451));
#25370=CARTESIAN_POINT('Ctrl Pts',(-0.154307462490191,-0.0161560295849065,
3.44040432158851));
#25371=CARTESIAN_POINT('Ctrl Pts',(-0.154184766718538,-0.000123847547745311,
3.43957882764113));
#25372=CARTESIAN_POINT('Origin',(0.,0.,3.71042117235887));
#25373=CARTESIAN_POINT('',(-0.154141660315178,0.000107924336747972,3.53957882764113));
#25374=CARTESIAN_POINT('',(-0.154329957770701,-0.000135440264844456,3.53542117235887));
#25375=CARTESIAN_POINT('',(-0.1543,1.43283619370552E-14,3.71042117235887));
#25376=CARTESIAN_POINT('Ctrl Pts',(-0.154329957770701,-0.000135440264844458,
3.53542117235887));
#25377=CARTESIAN_POINT('Ctrl Pts',(-0.153965757190248,0.0399803656323286,
3.5333506566435));
#25378=CARTESIAN_POINT('Ctrl Pts',(-0.117549955642843,0.13168538088825,
3.52864772941951));
#25379=CARTESIAN_POINT('Ctrl Pts',(0.0365555273815534,0.178349539831362,
3.52131239068689));
#25380=CARTESIAN_POINT('Ctrl Pts',(0.169323388748115,0.0668919258489962,
3.51341515616108));
#25381=CARTESIAN_POINT('Ctrl Pts',(0.148577699872602,-0.105212180693424,
3.50551792163523));
#25382=CARTESIAN_POINT('Ctrl Pts',(-0.00687287246844015,-0.181927682017732,
3.4976206871094));
#25383=CARTESIAN_POINT('Ctrl Pts',(-0.133449900938225,-0.107089534990244,
3.49092177068394));
#25384=CARTESIAN_POINT('Ctrl Pts',(-0.154001816923033,-0.0278717244546827,
3.4868552657671));
#25385=CARTESIAN_POINT('Ctrl Pts',(-0.154061344734167,3.64105721256669E-5,
3.48542117235887));
#25386=CARTESIAN_POINT('Ctrl Pts',(-0.154141660315178,0.000107924336747963,
3.53957882764113));
#25387=CARTESIAN_POINT('Ctrl Pts',(-0.154258987201045,0.017967079764623,
3.53865992635852));
#25388=CARTESIAN_POINT('Ctrl Pts',(-0.14316956514131,0.0868471600938436,
3.53510861356731));
#25389=CARTESIAN_POINT('Ctrl Pts',(-0.0418557834629445,0.177179558878914,
3.52892488926748));
#25390=CARTESIAN_POINT('Ctrl Pts',(0.125477426630257,0.13191056683484,3.52102765474164));
#25391=CARTESIAN_POINT('Ctrl Pts',(0.179050327003836,-0.0329543119327003,
3.51313042021581));
#25392=CARTESIAN_POINT('Ctrl Pts',(0.0702903405429243,-0.167940855985405,
3.50523318568997));
#25393=CARTESIAN_POINT('Ctrl Pts',(-0.101176526834898,-0.15076997316947,
3.49738265483174));
#25394=CARTESIAN_POINT('Ctrl Pts',(-0.154469279323916,-0.0498985397050101,
3.49216453548213));
#25395=CARTESIAN_POINT('Ctrl Pts',(-0.154545466983052,1.64397697926493E-5,
3.48957882764113));
#25396=CARTESIAN_POINT('Origin',(0.,0.,3.71042117235887));
#25397=CARTESIAN_POINT('',(-0.154140927489633,-0.000180264065019253,3.58957882764113));
#25398=CARTESIAN_POINT('',(-0.15446591465964,9.2330361050462E-5,3.58542117235887));
#25399=CARTESIAN_POINT('',(-0.1543,1.43283619370552E-14,3.71042117235887));
#25400=CARTESIAN_POINT('',(-0.0398513841857247,-0.149064942821851,3.6));
#25401=CARTESIAN_POINT('Ctrl Pts',(-0.0398513841857247,-0.149064942821851,
3.6));
#25402=CARTESIAN_POINT('Ctrl Pts',(-0.0891618565331957,-0.135882161272422,
3.59736758849139));
#25403=CARTESIAN_POINT('Ctrl Pts',(-0.14437796139003,-0.0838321271698221,
3.59389386437176));
#25404=CARTESIAN_POINT('Ctrl Pts',(-0.154259564981832,-0.0165262407662603,
3.59042014025214));
#25405=CARTESIAN_POINT('Ctrl Pts',(-0.154140927489633,-0.000180264065019272,
3.58957882764113));
#25406=CARTESIAN_POINT('',(0.0399440158046003,-0.149318575284508,3.6));
#25407=CARTESIAN_POINT('Origin',(0.,0.,3.6));
#25408=CARTESIAN_POINT('Ctrl Pts',(0.0399441988940755,-0.14931907659749,
3.6));
#25409=CARTESIAN_POINT('Ctrl Pts',(-0.00742263582378978,-0.161856507480607,
3.59746250047314));
#25410=CARTESIAN_POINT('Ctrl Pts',(-0.110807703402812,-0.13923343552822,
3.59260289125943));
#25411=CARTESIAN_POINT('Ctrl Pts',(-0.154134073844742,-0.0447846479172299,
3.58774328204572));
#25412=CARTESIAN_POINT('Ctrl Pts',(-0.15446591465964,9.23303610504333E-5,
3.58542117235887));
#25413=CARTESIAN_POINT('Origin',(-1.70916393953233E-17,-6.81365885416763E-18,
2.7));
#25414=CARTESIAN_POINT('Ctrl Pts',(-0.0958116152722464,0.0825211298936403,
2.7));
#25415=CARTESIAN_POINT('Ctrl Pts',(-0.100666302508711,0.0779874972024075,
2.7));
#25416=CARTESIAN_POINT('Ctrl Pts',(-0.10511524090547,0.0730607151536329,
2.7));
#25417=CARTESIAN_POINT('Ctrl Pts',(-0.109154515912936,0.0678088625732328,
2.7));
#25418=CARTESIAN_POINT('Ctrl Pts',(-0.111628556611506,0.0645921226872924,
2.7));
#25419=CARTESIAN_POINT('Ctrl Pts',(-0.113949938179476,0.0612512837881844,
2.7));
#25420=CARTESIAN_POINT('Ctrl Pts',(-0.116112529388643,0.0578058814506189,
2.7));
#25421=CARTESIAN_POINT('Ctrl Pts',(-0.120278296492253,0.0511690544554421,
2.7));
#25422=CARTESIAN_POINT('Ctrl Pts',(-0.123843133570631,0.0441670378484578,
2.7));
#25423=CARTESIAN_POINT('Ctrl Pts',(-0.126794163478656,0.0368991818833284,
2.7));
#25424=CARTESIAN_POINT('Ctrl Pts',(-0.128540684647383,0.0325978143303114,
2.7));
#25425=CARTESIAN_POINT('Ctrl Pts',(-0.130072629552482,0.0281986906446855,
2.7));
#25426=CARTESIAN_POINT('Ctrl Pts',(-0.13137784724267,0.0237479033105473,
2.7));
#25427=CARTESIAN_POINT('Ctrl Pts',(-0.134168070532741,0.0142332525574809,
2.7));
#25428=CARTESIAN_POINT('Ctrl Pts',(-0.135935427906691,0.00446386180413974,
2.7));
#25429=CARTESIAN_POINT('Ctrl Pts',(-0.136643098733652,-0.00537896296213896,
2.7));
#25430=CARTESIAN_POINT('Ctrl Pts',(-0.136956933956429,-0.00974402223206864,
2.7));
#25431=CARTESIAN_POINT('Ctrl Pts',(-0.137061776691848,-0.0141238933117977,
2.7));
#25432=CARTESIAN_POINT('Ctrl Pts',(-0.136951314304003,-0.0185038366743994,
2.7));
#25433=CARTESIAN_POINT('Ctrl Pts',(-0.136873618225507,-0.0215845633357163,
2.7));
#25434=CARTESIAN_POINT('Ctrl Pts',(-0.13668911286562,-0.0246638039330577,
2.7));
#25435=CARTESIAN_POINT('Ctrl Pts',(-0.136397287648127,-0.0277243541204411,
2.7));
#25436=CARTESIAN_POINT('Ctrl Pts',(-0.136038403631432,-0.031488191097877,
2.7));
#25437=CARTESIAN_POINT('Ctrl Pts',(-0.135517191903042,-0.0352286565107813,
2.7));
#25438=CARTESIAN_POINT('Ctrl Pts',(-0.134831588718299,-0.0389361603135121,
2.7));
#25439=CARTESIAN_POINT('Ctrl Pts',(-0.133471069242182,-0.0462933769129071,
2.7));
#25440=CARTESIAN_POINT('Ctrl Pts',(-0.131464409754198,-0.0535208830833808,
2.7));
#25441=CARTESIAN_POINT('Ctrl Pts',(-0.128873836850864,-0.0605679807942907,
2.7));
#25442=CARTESIAN_POINT('Ctrl Pts',(-0.127324936193114,-0.064781432678084,
2.7));
#25443=CARTESIAN_POINT('Ctrl Pts',(-0.125566934259419,-0.0689304108686299,
2.7));
#25444=CARTESIAN_POINT('Ctrl Pts',(-0.123610254975486,-0.0730036509543968,
2.7));
#25445=CARTESIAN_POINT('Ctrl Pts',(-0.122225010943685,-0.0758873281953399,
2.7));
#25446=CARTESIAN_POINT('Ctrl Pts',(-0.120744058613202,-0.0787247786003408,
2.7));
#25447=CARTESIAN_POINT('Ctrl Pts',(-0.11917349881759,-0.0815104554030709,
2.7));
#25448=CARTESIAN_POINT('Ctrl Pts',(-0.115042560220701,-0.0888374351557691,
2.7));
#25449=CARTESIAN_POINT('Ctrl Pts',(-0.11029123440495,-0.095810889712998,
2.7));
#25450=CARTESIAN_POINT('Ctrl Pts',(-0.104997440961948,-0.102362839712403,
2.7));
#25451=CARTESIAN_POINT('Ctrl Pts',(-0.101348653506344,-0.106878821158406,
2.7));
#25452=CARTESIAN_POINT('Ctrl Pts',(-0.0974416313653614,-0.11119454456931,
2.7));
#25453=CARTESIAN_POINT('Ctrl Pts',(-0.09329635857045,-0.115285413781573,
2.7));
#25454=CARTESIAN_POINT('Ctrl Pts',(-0.0904535089763086,-0.118090953116413,
2.7));
#25455=CARTESIAN_POINT('Ctrl Pts',(-0.0874964288334564,-0.12079189694507,
2.7));
#25456=CARTESIAN_POINT('Ctrl Pts',(-0.0844493327259437,-0.123365242468763,
2.7));
#25457=CARTESIAN_POINT('Ctrl Pts',(-0.0762097423121146,-0.130323773594913,
2.7));
#25458=CARTESIAN_POINT('Ctrl Pts',(-0.0672905965515622,-0.136377649112853,
2.7));
#25459=CARTESIAN_POINT('Ctrl Pts',(-0.0578267373609757,-0.141381851878944,
2.7));
#25460=CARTESIAN_POINT('Ctrl Pts',(-0.0536817029967175,-0.143573620798307,
2.7));
#25461=CARTESIAN_POINT('Ctrl Pts',(-0.0494316342727489,-0.145563646977507,
2.7));
#25462=CARTESIAN_POINT('Ctrl Pts',(-0.0450857388735961,-0.147337358046063,
2.7));
#25463=CARTESIAN_POINT('Ctrl Pts',(-0.043386269574786,-0.148030970576765,
2.7));
#25464=CARTESIAN_POINT('Ctrl Pts',(-0.0416721350945774,-0.148691483593437,
2.7));
#25465=CARTESIAN_POINT('Ctrl Pts',(-0.0399441884684126,-0.149319082708151,
2.7));
#25466=CARTESIAN_POINT('Ctrl Pts',(0.0398513841857358,-0.149064942821848,
2.7));
#25467=CARTESIAN_POINT('Ctrl Pts',(0.0462200530662091,-0.146737857425647,
2.7));
#25468=CARTESIAN_POINT('Ctrl Pts',(0.0524055534681357,-0.143963403134301,
2.7));
#25469=CARTESIAN_POINT('Ctrl Pts',(0.0583783483111506,-0.140779078044469,
2.7));
#25470=CARTESIAN_POINT('Ctrl Pts',(0.062793202477668,-0.138425350642158,
2.7));
#25471=CARTESIAN_POINT('Ctrl Pts',(0.067091772966825,-0.135847508755531,
2.7));
#25472=CARTESIAN_POINT('Ctrl Pts',(0.0712602009478766,-0.133058650089746,
2.7));
#25473=CARTESIAN_POINT('Ctrl Pts',(0.0751200675142575,-0.130476232360243,
2.7));
#25474=CARTESIAN_POINT('Ctrl Pts',(0.078861342939135,-0.127717307612303,
2.7));
#25475=CARTESIAN_POINT('Ctrl Pts',(0.0824683178131891,-0.124797523957272,
2.7));
#25476=CARTESIAN_POINT('Ctrl Pts',(0.0880430571667216,-0.12028486905563,
2.7));
#25477=CARTESIAN_POINT('Ctrl Pts',(0.093301870580488,-0.115385246850429,
2.7));
#25478=CARTESIAN_POINT('Ctrl Pts',(0.098201122907525,-0.11013722292202,
2.7));
#25479=CARTESIAN_POINT('Ctrl Pts',(0.100467267721939,-0.107709754113023,
2.7));
#25480=CARTESIAN_POINT('Ctrl Pts',(0.102654039344122,-0.10520989028497,
2.7));
#25481=CARTESIAN_POINT('Ctrl Pts',(0.104752062819345,-0.102648267464436,
2.7));
#25482=CARTESIAN_POINT('Ctrl Pts',(0.111288676944248,-0.0946672605266598,
2.7));
#25483=CARTESIAN_POINT('Ctrl Pts',(0.11698432795861,-0.0860702972477514,
2.7));
#25484=CARTESIAN_POINT('Ctrl Pts',(0.121705201609602,-0.0769745632194894,
2.7));
#25485=CARTESIAN_POINT('Ctrl Pts',(0.12379312017453,-0.0729517586830322,
2.7));
#25486=CARTESIAN_POINT('Ctrl Pts',(0.125689731189231,-0.0688311600363216,
2.7));
#25487=CARTESIAN_POINT('Ctrl Pts',(0.127380076370131,-0.0646223264534606,
2.7));
#25488=CARTESIAN_POINT('Ctrl Pts',(0.128615050131834,-0.0615473337827676,
2.7));
#25489=CARTESIAN_POINT('Ctrl Pts',(0.129739752069541,-0.0584245102417657,
2.7));
#25490=CARTESIAN_POINT('Ctrl Pts',(0.130743760465559,-0.0552728510655911,
2.7));
#25491=CARTESIAN_POINT('Ctrl Pts',(0.131931576408969,-0.0515442059342363,
2.7));
#25492=CARTESIAN_POINT('Ctrl Pts',(0.132952645794869,-0.0477702728539015,
2.7));
#25493=CARTESIAN_POINT('Ctrl Pts',(0.13379905511372,-0.0439575955102323,
2.7));
#25494=CARTESIAN_POINT('Ctrl Pts',(0.135238114697535,-0.0374753064460584,
2.7));
#25495=CARTESIAN_POINT('Ctrl Pts',(0.136172820012768,-0.0308808878255892,
2.7));
#25496=CARTESIAN_POINT('Ctrl Pts',(0.136617245503396,-0.0242291498972301,
2.7));
#25497=CARTESIAN_POINT('Ctrl Pts',(0.136949796542121,-0.0192518423303904,
2.7));
#25498=CARTESIAN_POINT('Ctrl Pts',(0.13700760567975,-0.0142424066500717,
2.7));
#25499=CARTESIAN_POINT('Ctrl Pts',(0.136793131026844,-0.00922497436481165,
2.7));
#25500=CARTESIAN_POINT('Ctrl Pts',(0.136645101058571,-0.00576195282855203,
2.7));
#25501=CARTESIAN_POINT('Ctrl Pts',(0.1363675285007,-0.00230375513318918,
2.7));
#25502=CARTESIAN_POINT('Ctrl Pts',(0.13596351343207,0.00113554936727295,
2.7));
#25503=CARTESIAN_POINT('Ctrl Pts',(0.13510375104742,0.00845454528710606,
2.7));
#25504=CARTESIAN_POINT('Ctrl Pts',(0.133671961121794,0.0156977511556185,
2.7));
#25505=CARTESIAN_POINT('Ctrl Pts',(0.131684102868306,0.0227886248739312,
2.7));
#25506=CARTESIAN_POINT('Ctrl Pts',(0.130343128964387,0.0275720024591066,
2.7));
#25507=CARTESIAN_POINT('Ctrl Pts',(0.128748781223598,0.0322859803615266,
2.7));
#25508=CARTESIAN_POINT('Ctrl Pts',(0.126902487239724,0.0369045444632721,
2.7));
#25509=CARTESIAN_POINT('Ctrl Pts',(0.125403567336896,0.0406541410687207,
2.7));
#25510=CARTESIAN_POINT('Ctrl Pts',(0.123736334503949,0.0443441630809861,
2.7));
#25511=CARTESIAN_POINT('Ctrl Pts',(0.121913684068145,0.047935992310073,
2.7));
#25512=CARTESIAN_POINT('Ctrl Pts',(0.117743460752234,0.0561540958496606,
2.7));
#25513=CARTESIAN_POINT('Ctrl Pts',(0.112753744605352,0.0638862445298334,
2.7));
#25514=CARTESIAN_POINT('Ctrl Pts',(0.106960788703284,0.0709645017846505,
2.7));
#25515=CARTESIAN_POINT('Ctrl Pts',(0.104535029275377,0.0739284720891533,
2.7));
#25516=CARTESIAN_POINT('Ctrl Pts',(0.101968022916162,0.0767773427076814,
2.7));
#25517=CARTESIAN_POINT('Ctrl Pts',(0.0992594073891335,0.0794964656217155,
2.7));
#25518=CARTESIAN_POINT('Ctrl Pts',(0.0981919726164135,0.0805680412369242,
2.7));
#25519=CARTESIAN_POINT('Ctrl Pts',(0.0971025353237707,0.0816194476022307,
2.7));
#25520=CARTESIAN_POINT('Ctrl Pts',(0.0959918005672169,0.0826503307119895,
2.7));
#25521=CARTESIAN_POINT('Origin',(0.,0.,3.71042117235887));
#25522=CARTESIAN_POINT('Ctrl Pts',(-0.15446591465964,9.23303610504368E-5,
3.58542117235887));
#25523=CARTESIAN_POINT('Ctrl Pts',(-0.154510258305412,0.00608920819750747,
3.58511087053711));
#25524=CARTESIAN_POINT('Ctrl Pts',(-0.151481073290489,0.0629168758661166,
3.58216815720674));
#25525=CARTESIAN_POINT('Ctrl Pts',(-0.0810549264538156,0.163034932450524,
3.57659303236775));
#25526=CARTESIAN_POINT('Ctrl Pts',(0.0921890963056651,0.156981846810788,
3.56869579784192));
#25527=CARTESIAN_POINT('Ctrl Pts',(0.181852962765875,0.00863524897295638,
3.56079856331608));
#25528=CARTESIAN_POINT('Ctrl Pts',(0.10664300202618,-0.147556335146073,
3.55290132879024));
#25529=CARTESIAN_POINT('Ctrl Pts',(-0.0652523071804818,-0.169960705131912,
3.54500409426442));
#25530=CARTESIAN_POINT('Ctrl Pts',(-0.1484307843993,-0.072802923531341,
3.53917737545395));
#25531=CARTESIAN_POINT('Ctrl Pts',(-0.154428794390259,-0.0110220529132785,
3.53598306815211));
#25532=CARTESIAN_POINT('Ctrl Pts',(-0.154329957770701,-0.000135440264844458,
3.53542117235887));
#25533=CARTESIAN_POINT('Ctrl Pts',(-0.154140927489633,-0.000180264065019272,
3.58957882764113));
#25534=CARTESIAN_POINT('Ctrl Pts',(-0.153888356116389,0.0346192390763322,
3.58778772874353));
#25535=CARTESIAN_POINT('Ctrl Pts',(-0.125147291545086,0.121067307783401,
3.58336421833732));
#25536=CARTESIAN_POINT('Ctrl Pts',(0.0176337902165689,0.181151815132919,
3.5763082964225));
#25537=CARTESIAN_POINT('Ctrl Pts',(0.161334465098627,0.0843516096779105,
3.56841106189666));
#25538=CARTESIAN_POINT('Ctrl Pts',(0.158825384561566,-0.0890212772063117,
3.56051382737082));
#25539=CARTESIAN_POINT('Ctrl Pts',(0.0122890037691484,-0.181634540286447,
3.55261659284499));
#25540=CARTESIAN_POINT('Ctrl Pts',(-0.127027468209772,-0.117980653400407,
3.54563825960175));
#25541=CARTESIAN_POINT('Ctrl Pts',(-0.153922876401689,-0.0331947231106458,
3.54129233786714));
#25542=CARTESIAN_POINT('Ctrl Pts',(-0.154141660315178,0.000107924336747963,
3.53957882764113));
#25543=CARTESIAN_POINT('Ctrl Pts',(0.0958116152722374,0.0825211298936506,
3.6));
#25544=CARTESIAN_POINT('Ctrl Pts',(0.12310948837823,0.0508267830136165,
3.59736758849139));
#25545=CARTESIAN_POINT('Ctrl Pts',(0.143341746937054,-0.0412253317476725,
3.59210276547417));
#25546=CARTESIAN_POINT('Ctrl Pts',(0.0436608358730345,-0.142764465257081,
3.58420553094833));
#25547=CARTESIAN_POINT('Ctrl Pts',(-0.0955856094744946,-0.114504131671876,
3.57630829642249));
#25548=CARTESIAN_POINT('Ctrl Pts',(-0.148178789486409,0.0173870346414916,
3.56841106189666));
#25549=CARTESIAN_POINT('Ctrl Pts',(-0.066425116332372,0.133608342244775,
3.56051382737082));
#25550=CARTESIAN_POINT('Ctrl Pts',(0.0755496515090821,0.128647793449282,
3.55261659284499));
#25551=CARTESIAN_POINT('Ctrl Pts',(0.149029858339241,0.0070766508919659,
3.54471935831915));
#25552=CARTESIAN_POINT('Ctrl Pts',(0.0873947349721999,-0.120923516391581,
3.53682212379332));
#25553=CARTESIAN_POINT('Ctrl Pts',(-0.0534747520607383,-0.13928406457505,
3.52892488926748));
#25554=CARTESIAN_POINT('Ctrl Pts',(-0.145862599457632,-0.0313691495625942,
3.52102765474165));
#25555=CARTESIAN_POINT('Ctrl Pts',(-0.106007076394109,0.104987796417131,
3.5131304202158));
#25556=CARTESIAN_POINT('Ctrl Pts',(0.029957527138026,0.146158777133349,
3.50523318568998));
#25557=CARTESIAN_POINT('Ctrl Pts',(0.138761779048601,0.0548184317796861,
3.49733595116414));
#25558=CARTESIAN_POINT('Ctrl Pts',(0.121760532397217,-0.0862221662260755,
3.4894387166383));
#25559=CARTESIAN_POINT('Ctrl Pts',(-0.0056323702114988,-0.149091091323021,
3.48154148211246));
#25560=CARTESIAN_POINT('Ctrl Pts',(-0.127918803859021,-0.0767897408219312,
3.47364424758663));
#25561=CARTESIAN_POINT('Ctrl Pts',(-0.134230305961673,0.0651314716709306,
3.46574701306079));
#25562=CARTESIAN_POINT('Ctrl Pts',(-0.0188446861564537,0.148002567505592,
3.45784977853496));
#25563=CARTESIAN_POINT('Ctrl Pts',(0.113626077839972,0.0966902152561852,
3.44995254400912));
#25564=CARTESIAN_POINT('Ctrl Pts',(0.143080115058725,-0.0422843201504222,
3.44205530948329));
#25565=CARTESIAN_POINT('Ctrl Pts',(0.0428135339010967,-0.142922651128878,
3.43415807495745));
#25566=CARTESIAN_POINT('Ctrl Pts',(-0.0962690497602299,-0.113983126411312,
3.42626084043161));
#25567=CARTESIAN_POINT('Ctrl Pts',(-0.148071296290933,0.0182968362857149,
3.41836360590578));
#25568=CARTESIAN_POINT('Ctrl Pts',(-0.0656277734239754,0.133988351515145,
3.41046637137994));
#25569=CARTESIAN_POINT('Ctrl Pts',(0.076315808940436,0.128202107291143,
3.40256913685411));
#25570=CARTESIAN_POINT('Ctrl Pts',(0.149069246106613,0.0061840816248079,
3.39467190232827));
#25571=CARTESIAN_POINT('Ctrl Pts',(0.086672143362556,-0.121440613321149,
3.38677466780244));
#25572=CARTESIAN_POINT('Ctrl Pts',(-0.0543044603643882,-0.138963695209725,
3.37887743327661));
#25573=CARTESIAN_POINT('Ctrl Pts',(-0.14604705151224,-0.0304982252781714,
3.37098019875076));
#25574=CARTESIAN_POINT('Ctrl Pts',(-0.105379112789235,0.105617827984774,
3.36308296422493));
#25575=CARTESIAN_POINT('Ctrl Pts',(0.0308286127169663,0.145977668287988,
3.35518572969909));
#25576=CARTESIAN_POINT('Ctrl Pts',(0.139086215966064,0.0539898835791761,
3.34728849517326));
#25577=CARTESIAN_POINT('Ctrl Pts',(0.121244186506805,-0.0869467091899644,
3.33939126064743));
#25578=CARTESIAN_POINT('Ctrl Pts',(-0.00652136974010873,-0.149054871565549,
3.33149402612159));
#25579=CARTESIAN_POINT('Ctrl Pts',(-0.12837446138172,-0.0760255264081264,
3.32359679159575));
#25580=CARTESIAN_POINT('Ctrl Pts',(-0.133839510420159,0.0659307853068325,
3.31569955706992));
#25581=CARTESIAN_POINT('Ctrl Pts',(-0.0179617435035512,0.148112318093405,
3.30780232254408));
#25582=CARTESIAN_POINT('Ctrl Pts',(0.114200665588904,0.0960108899018034,
3.29990508801825));
#25583=CARTESIAN_POINT('Ctrl Pts',(0.142825410033637,-0.0431368201123976,
3.29200785349241));
#25584=CARTESIAN_POINT('Ctrl Pts',(0.0419604590288785,-0.143175426937629,
3.28411061896658));
#25585=CARTESIAN_POINT('Ctrl Pts',(-0.0969470717891682,-0.113407002747589,
3.27621338444074));
#25586=CARTESIAN_POINT('Ctrl Pts',(-0.147959550895179,0.0191795281376522,
3.26831614991491));
#25587=CARTESIAN_POINT('Ctrl Pts',(-0.0648275722345507,0.134377337668448,
3.26041891538907));
#25588=CARTESIAN_POINT('Ctrl Pts',(0.0770789801059626,0.127744721325426,
3.25252168086324));
#25589=CARTESIAN_POINT('Ctrl Pts',(0.149103473944927,0.00529500313887513,
3.24462444633739));
#25590=CARTESIAN_POINT('Ctrl Pts',(0.085946395912033,-0.121955319811881,
3.23672721181157));
#25591=CARTESIAN_POINT('Ctrl Pts',(-0.0551321992305218,-0.138637381714645,
3.22882997728572));
#25592=CARTESIAN_POINT('Ctrl Pts',(-0.146226329520922,-0.0296267371731131,
3.22093274275989));
#25593=CARTESIAN_POINT('Ctrl Pts',(-0.104747391252292,0.106244374093527,
3.21303550823405));
#25594=CARTESIAN_POINT('Ctrl Pts',(0.0316985965714106,0.145791227363271,
3.20513827370822));
#25595=CARTESIAN_POINT('Ctrl Pts',(0.139405709322103,0.0531594884201076,
3.19724103918239));
#25596=CARTESIAN_POINT('Ctrl Pts',(0.12072352734024,-0.0876681980379225,
3.18934380465655));
#25597=CARTESIAN_POINT('Ctrl Pts',(-0.00741013659566878,-0.149013331203351,
3.18144657013072));
#25598=CARTESIAN_POINT('Ctrl Pts',(-0.128825553891948,-0.0752586185437851,
3.17354933560487));
#25599=CARTESIAN_POINT('Ctrl Pts',(-0.133443954917441,0.0667277595658497,
3.16565210107904));
#25600=CARTESIAN_POINT('Ctrl Pts',(-0.0170781621796165,0.148216798566333,
3.15775486655321));
#25601=CARTESIAN_POINT('Ctrl Pts',(0.114771192054407,0.0953281515350871,
3.14985763202737));
#25602=CARTESIAN_POINT('Ctrl Pts',(0.14256562565491,-0.0439877867403021,
3.14196039750153));
#25603=CARTESIAN_POINT('Ctrl Pts',(0.0411058919243144,-0.143423110584706,
3.1340631629757));
#25604=CARTESIAN_POINT('Ctrl Pts',(-0.0976216460800827,-0.112826846172802,
3.12616592844987));
#25605=CARTESIAN_POINT('Ctrl Pts',(-0.147842543583951,0.0200615380096788,
3.11826869392402));
#25606=CARTESIAN_POINT('Ctrl Pts',(-0.0640250655728793,0.134761544882338,
3.11037145939819));
#25607=CARTESIAN_POINT('Ctrl Pts',(0.0778394100992752,0.127282792380129,
3.10247422487235));
#25608=CARTESIAN_POINT('Ctrl Pts',(0.14913239918967,0.00440573633107837,
3.09457699034652));
#25609=CARTESIAN_POINT('Ctrl Pts',(0.0852175919350427,-0.122465689176514,
3.08667975582068));
#25610=CARTESIAN_POINT('Ctrl Pts',(-0.0559579774207319,-0.138306137838011,
3.07878252129485));
#25611=CARTESIAN_POINT('Ctrl Pts',(-0.14640040725691,-0.028754195445133,
3.07088528676901));
#25612=CARTESIAN_POINT('Ctrl Pts',(-0.104111944565534,0.106867141813886,
3.06298805224318));
#25613=CARTESIAN_POINT('Ctrl Pts',(0.0325674531231242,0.145599601640112,
3.05509081771734));
#25614=CARTESIAN_POINT('Ctrl Pts',(0.139720244968427,0.0523272027405333,
3.04719358319151));
#25615=CARTESIAN_POINT('Ctrl Pts',(0.120198574861694,-0.0883865691262194,
3.03929634866567));
#25616=CARTESIAN_POINT('Ctrl Pts',(-0.00829863992324496,-0.148966491453986,
3.03139911413983));
#25617=CARTESIAN_POINT('Ctrl Pts',(-0.129272064956395,-0.0744890342439453,
3.023501879614));
#25618=CARTESIAN_POINT('Ctrl Pts',(-0.133043653723939,0.0675223607738245,
3.01560464508816));
#25619=CARTESIAN_POINT('Ctrl Pts',(-0.0161939735020032,0.148316007979255,
3.00770741056233));
#25620=CARTESIAN_POINT('Ctrl Pts',(0.115337636891868,0.0946420229965858,
2.9998101760365));
#25621=CARTESIAN_POINT('Ctrl Pts',(0.142300771189819,-0.0448371890228274,
2.99191294151066));
#25622=CARTESIAN_POINT('Ctrl Pts',(0.040249862963706,-0.14366569365053,
2.98401570698482));
#25623=CARTESIAN_POINT('Ctrl Pts',(-0.0982927486352741,-0.112242677117094,
2.97611847245899));
#25624=CARTESIAN_POINT('Ctrl Pts',(-0.14772027852239,0.0209428344297273,
2.96822123793315));
#25625=CARTESIAN_POINT('Ctrl Pts',(-0.0632202819765869,0.135140959547726,
2.96032400340732));
#25626=CARTESIAN_POINT('Ctrl Pts',(0.0785970718760291,0.126816336854618,
2.95242676888148));
#25627=CARTESIAN_POINT('Ctrl Pts',(0.149156020812652,0.00351631284117927,
2.94452953435565));
#25628=CARTESIAN_POINT('Ctrl Pts',(0.0844857573500313,-0.122971703272108,
2.93663229982981));
#25629=CARTESIAN_POINT('Ctrl Pts',(-0.0567817655678681,-0.137969975356402,
2.92873506530398));
#25630=CARTESIAN_POINT('Ctrl Pts',(-0.146569278528953,-0.0278806311257436,
2.92083783077813));
#25631=CARTESIAN_POINT('Ctrl Pts',(-0.103472795328523,0.107486108997575,
2.91294059625231));
#25632=CARTESIAN_POINT('Ctrl Pts',(0.0334351514749053,0.145402797936144,
2.90504336172646));
#25633=CARTESIAN_POINT('Ctrl Pts',(0.140029811715087,0.0514930561329736,
2.89714612720063));
#25634=CARTESIAN_POINT('Ctrl Pts',(0.119669347747977,-0.0891017968949556,
2.88924889267479));
#25635=CARTESIAN_POINT('Ctrl Pts',(-0.00918684813991898,-0.148914354007184,
2.88135165814896));
#25636=CARTESIAN_POINT('Ctrl Pts',(-0.129713978666681,-0.073716800831252,
2.87345442362312));
#25637=CARTESIAN_POINT('Ctrl Pts',(-0.132638621131497,0.0683145605832212,
2.86555718909729));
#25638=CARTESIAN_POINT('Ctrl Pts',(-0.0153092088077737,0.148409942975243,
2.85765995457145));
#25639=CARTESIAN_POINT('Ctrl Pts',(0.11589997974986,0.0939525283576191,
2.84976272004561));
#25640=CARTESIAN_POINT('Ctrl Pts',(0.14203085645546,-0.0456849961183085,
2.84186548551979));
#25641=CARTESIAN_POINT('Ctrl Pts',(0.0393924018242494,-0.143903168728488,
2.83396825099394));
#25642=CARTESIAN_POINT('Ctrl Pts',(-0.0989603541143928,-0.111654514006987,
2.82607101646811));
#25643=CARTESIAN_POINT('Ctrl Pts',(-0.14759276289462,0.0218233815372009,
2.81817378194227));
#25644=CARTESIAN_POINT('Ctrl Pts',(-0.0624132446091692,0.135515576866934,
2.81027654741644));
#25645=CARTESIAN_POINT('Ctrl Pts',(0.0793519279903814,0.126345354605138,
2.8023793128906));
#25646=CARTESIAN_POINT('Ctrl Pts',(0.149174358180394,0.00262679649731067,
2.79448207836477));
#25647=CARTESIAN_POINT('Ctrl Pts',(0.0837508793007237,-0.12347340605925,
2.78658484383893));
#25648=CARTESIAN_POINT('Ctrl Pts',(-0.0576034595552612,-0.137628787005506,
2.7786876093131));
#25649=CARTESIAN_POINT('Ctrl Pts',(-0.146733081304572,-0.0270063046901533,
2.77079037478726));
#25650=CARTESIAN_POINT('Ctrl Pts',(-0.102829689230287,0.108101695072837,
2.76289314026143));
#25651=CARTESIAN_POINT('Ctrl Pts',(0.0343011276704797,0.145199973805224,
2.75499590573559));
#25652=CARTESIAN_POINT('Ctrl Pts',(0.140335424370929,0.0506587128142576,
2.74709867120975));
#25653=CARTESIAN_POINT('Ctrl Pts',(0.11913389087728,-0.0898170012241629,
2.73920143668392));
#25654=CARTESIAN_POINT('Ctrl Pts',(-0.0100709312277202,-0.14885086814231,
2.73130420215808));
#25655=CARTESIAN_POINT('Ctrl Pts',(-0.130158589013459,-0.0729535941759648,
2.72340696763225));
#25656=CARTESIAN_POINT('Ctrl Pts',(-0.132214800612389,0.0691267612890124,
2.71550973310641));
#25657=CARTESIAN_POINT('Ctrl Pts',(-0.0144510241825876,0.148455288920992,
2.70761249858058));
#25658=CARTESIAN_POINT('Ctrl Pts',(0.116510849855331,0.0933444320528056,
2.69971526405474));
#25659=CARTESIAN_POINT('Ctrl Pts',(0.141650318794474,-0.0467072968399595,
2.6918180295289));
#25660=CARTESIAN_POINT('Ctrl Pts',(0.073068805953493,-0.111356443894342,
2.68655320651168));
#25661=CARTESIAN_POINT('Ctrl Pts',(0.0326585063531192,-0.122159831625552,
2.68392079500307));
#25662=CARTESIAN_POINT('Ctrl Pts',(0.102845629995664,0.088579422941069,
3.60535973499898));
#25663=CARTESIAN_POINT('Ctrl Pts',(0.132147577876935,0.0545582339347427,
3.60272732349037));
#25664=CARTESIAN_POINT('Ctrl Pts',(0.153865188751202,-0.0442518916242316,
3.59746250047314));
#25665=CARTESIAN_POINT('Ctrl Pts',(0.046866198411756,-0.153245525906639,
3.58956526594731));
#25666=CARTESIAN_POINT('Ctrl Pts',(-0.102603031970513,-0.122910458459966,
3.58166803142147));
#25667=CARTESIAN_POINT('Ctrl Pts',(-0.159057343031147,0.0186635046949134,
3.57377079689563));
#25668=CARTESIAN_POINT('Ctrl Pts',(-0.0713017197061865,0.143417205646691,
3.5658735623698));
#25669=CARTESIAN_POINT('Ctrl Pts',(0.0810961331079431,0.138092477903117,
3.55797632784396));
#25670=CARTESIAN_POINT('Ctrl Pts',(0.159970893148119,0.00759618358562943,
3.55007909331813));
#25671=CARTESIAN_POINT('Ctrl Pts',(0.0938108239901933,-0.129801122643079,
3.54218185879229));
#25672=CARTESIAN_POINT('Ctrl Pts',(-0.0574006037673195,-0.149509611427338,
3.53428462426646));
#25673=CARTESIAN_POINT('Ctrl Pts',(-0.156571109790821,-0.0336721173108959,
3.52638738974062));
#25674=CARTESIAN_POINT('Ctrl Pts',(-0.113789591426601,0.112695480957047,
3.51849015521479));
#25675=CARTESIAN_POINT('Ctrl Pts',(0.0321568605525351,0.15688903136602,
3.51059292068895));
#25676=CARTESIAN_POINT('Ctrl Pts',(0.148948982281772,0.0588429298027895,
3.50269568616312));
#25677=CARTESIAN_POINT('Ctrl Pts',(0.130699588222345,-0.092552171048525,
3.49479845163728));
#25678=CARTESIAN_POINT('Ctrl Pts',(-0.00604587096381251,-0.160036621554591,
3.48690121711144));
#25679=CARTESIAN_POINT('Ctrl Pts',(-0.137309969504135,-0.0824272636422575,
3.47900398258561));
#25680=CARTESIAN_POINT('Ctrl Pts',(-0.144084830862247,0.0699131020545748,
3.47110674805977));
#25681=CARTESIAN_POINT('Ctrl Pts',(-0.0202281697717358,0.158868183704434,
3.46320951353394));
#25682=CARTESIAN_POINT('Ctrl Pts',(0.121967942260279,0.103788732443176,
3.4553122790081));
#25683=CARTESIAN_POINT('Ctrl Pts',(0.153584349154903,-0.045388625715703,
3.44741504448227));
#25684=CARTESIAN_POINT('Ctrl Pts',(0.0459566917214356,-0.153415325002449,
3.43951780995643));
#25685=CARTESIAN_POINT('Ctrl Pts',(-0.103336647060408,-0.122351203571073,
3.43162057543059));
#25686=CARTESIAN_POINT('Ctrl Pts',(-0.158941958217129,0.0196400994742142,
3.42372334090476));
#25687=CARTESIAN_POINT('Ctrl Pts',(-0.0704458398266582,0.14382511331743,
3.41582610637892));
#25688=CARTESIAN_POINT('Ctrl Pts',(0.0819185380270082,0.137614071672475,
3.40792887185309));
#25689=CARTESIAN_POINT('Ctrl Pts',(0.160013172570483,0.00663808629925336,
3.40003163732726));
#25690=CARTESIAN_POINT('Ctrl Pts',(0.0930351832799072,-0.130356182270652,
3.39213440280141));
#25691=CARTESIAN_POINT('Ctrl Pts',(-0.0582912251492787,-0.149165722128378,
3.38423716827558));
#25692=CARTESIAN_POINT('Ctrl Pts',(-0.15676910340262,-0.0327372540747895,
3.37633993374974));
#25693=CARTESIAN_POINT('Ctrl Pts',(-0.113115525840982,0.11337176632503,
3.36844269922391));
#25694=CARTESIAN_POINT('Ctrl Pts',(0.0330918969246043,0.156694626405347,
3.36054546469807));
#25695=CARTESIAN_POINT('Ctrl Pts',(0.149297237752422,0.0579535536930025,
3.35264823017224));
#25696=CARTESIAN_POINT('Ctrl Pts',(0.130145334771507,-0.0933299063718294,
3.3447509956464));
#25697=CARTESIAN_POINT('Ctrl Pts',(-0.00700013643909911,-0.159997742721738,
3.33685376112057));
#25698=CARTESIAN_POINT('Ctrl Pts',(-0.137799079147585,-0.0816069443874761,
3.32895652659473));
#25699=CARTESIAN_POINT('Ctrl Pts',(-0.143665345045706,0.0707710973426707,
3.3210592920689));
#25700=CARTESIAN_POINT('Ctrl Pts',(-0.019280405838002,0.158985991637365,
3.31316205754306));
#25701=CARTESIAN_POINT('Ctrl Pts',(0.122584713398713,0.103059534382534,
3.30526482301722));
#25702=CARTESIAN_POINT('Ctrl Pts',(0.153310944947138,-0.0463037120067701,
3.29736758849139));
#25703=CARTESIAN_POINT('Ctrl Pts',(0.04504098831306,-0.15368665836036,3.28947035396555));
#25704=CARTESIAN_POINT('Ctrl Pts',(-0.1040644461119,-0.121732783758583,
3.28157311943972));
#25705=CARTESIAN_POINT('Ctrl Pts',(-0.158822009027328,0.0205875941944168,
3.27367588491388));
#25706=CARTESIAN_POINT('Ctrl Pts',(-0.0695868918252512,0.14424265690943,
3.26577865038805));
#25707=CARTESIAN_POINT('Ctrl Pts',(0.0827377374433846,0.137123106692272,
3.25788141586221));
#25708=CARTESIAN_POINT('Ctrl Pts',(0.160049913247329,0.00568373606998795,
3.24998418133638));
#25709=CARTESIAN_POINT('Ctrl Pts',(0.0922561550425197,-0.130908675965198,
3.24208694681054));
#25710=CARTESIAN_POINT('Ctrl Pts',(-0.0591797325073638,-0.148815452311067,
3.2341897122847));
#25711=CARTESIAN_POINT('Ctrl Pts',(-0.156961543115644,-0.0318017856251262,
3.22629247775887));
#25712=CARTESIAN_POINT('Ctrl Pts',(-0.112437426434515,0.114044310348977,
3.21839524323303));
#25713=CARTESIAN_POINT('Ctrl Pts',(0.0340257506890165,0.156494497910436,
3.21049800870719));
#25714=CARTESIAN_POINT('Ctrl Pts',(0.149640186729828,0.0570621950300983,
3.20260077418136));
#25715=CARTESIAN_POINT('Ctrl Pts',(0.129586451385121,-0.094104363361123,
3.19470353965552));
#25716=CARTESIAN_POINT('Ctrl Pts',(-0.00795415215963184,-0.159953152671687,
3.18680630512969));
#25717=CARTESIAN_POINT('Ctrl Pts',(-0.138283288637936,-0.0807837339423469,
3.17890907060385));
#25718=CARTESIAN_POINT('Ctrl Pts',(-0.143240749815163,0.0716265815084065,
3.17101183607802));
#25719=CARTESIAN_POINT('Ctrl Pts',(-0.0183319563451689,0.159098142549652,
3.16311460155218));
#25720=CARTESIAN_POINT('Ctrl Pts',(0.123197125094384,0.10232667274308,3.15521736702635));
#25721=CARTESIAN_POINT('Ctrl Pts',(0.153032088484722,-0.047217152393966,
3.14732013250051));
#25722=CARTESIAN_POINT('Ctrl Pts',(0.0441236831200233,-0.153952525715282,
3.13942289797468));
#25723=CARTESIAN_POINT('Ctrl Pts',(-0.104788544309502,-0.121110034958652,
3.13152566344884));
#25724=CARTESIAN_POINT('Ctrl Pts',(-0.158696411618254,0.021534356867118,
3.123628428923));
#25725=CARTESIAN_POINT('Ctrl Pts',(-0.0687254690952325,0.14465507071593,
3.11573119439717));
#25726=CARTESIAN_POINT('Ctrl Pts',(0.0835539944442463,0.136627265209407,
3.10783395987133));
#25727=CARTESIAN_POINT('Ctrl Pts',(0.160080962040421,0.00472918369319909,
3.0999367253455));
#25728=CARTESIAN_POINT('Ctrl Pts',(0.091473845883615,-0.131456514123307,
3.09203949081966));
#25729=CARTESIAN_POINT('Ctrl Pts',(-0.0600661352464005,-0.148459890147985,
3.08414225629383));
#25730=CARTESIAN_POINT('Ctrl Pts',(-0.157148400777682,-0.0308651862007597,
3.07624502176799));
#25731=CARTESIAN_POINT('Ctrl Pts',(-0.111755328396166,0.114712798593949,
3.06834778724216));
#25732=CARTESIAN_POINT('Ctrl Pts',(0.0349583943897092,0.156288803974834,
3.06045055271632));
#25733=CARTESIAN_POINT('Ctrl Pts',(0.149977814027003,0.0561688070540271,
3.05255331819049));
#25734=CARTESIAN_POINT('Ctrl Pts',(0.129022959493032,-0.0948754737002677,
3.04465608366465));
#25735=CARTESIAN_POINT('Ctrl Pts',(-0.00890788500525998,-0.159902874179684,
3.03675884913881));
#25736=CARTESIAN_POINT('Ctrl Pts',(-0.138762580335427,-0.0799576505710677,
3.02886161461298));
#25737=CARTESIAN_POINT('Ctrl Pts',(-0.142811060488699,0.072479518405434,
3.02096438008714));
#25738=CARTESIAN_POINT('Ctrl Pts',(-0.0173828549097553,0.159204635426789,
3.01306714556131));
#25739=CARTESIAN_POINT('Ctrl Pts',(0.123805155509077,0.101590172042203,
3.00516991103547));
#25740=CARTESIAN_POINT('Ctrl Pts',(0.152747789715287,-0.0481289135892851,
2.99727267650964));
#25741=CARTESIAN_POINT('Ctrl Pts',(0.0432048087487045,-0.154212918029513,
2.9893754419838));
#25742=CARTESIAN_POINT('Ctrl Pts',(-0.105508915893722,-0.120482979101306,
2.98147820745797));
#25743=CARTESIAN_POINT('Ctrl Pts',(-0.158565170460834,0.0224803537097271,
2.97358097293213));
#25744=CARTESIAN_POINT('Ctrl Pts',(-0.067861602269319,0.145062340128731,
2.9656837384063));
#25745=CARTESIAN_POINT('Ctrl Pts',(0.0843672799997867,0.136126564827205,
2.95778650388046));
#25746=CARTESIAN_POINT('Ctrl Pts',(0.160106317846084,0.0037744631314833,
2.94988926935462));
#25747=CARTESIAN_POINT('Ctrl Pts',(0.0906882836244439,-0.131999677270073,
2.94199203482879));
#25748=CARTESIAN_POINT('Ctrl Pts',(-0.0609504018432475,-0.148099048280287,
2.93409480030295));
#25749=CARTESIAN_POINT('Ctrl Pts',(-0.157329669742954,-0.0299274891113821,
2.92619756577712));
#25750=CARTESIAN_POINT('Ctrl Pts',(-0.111069255984644,0.115377207285653,
2.91830033125128));
#25751=CARTESIAN_POINT('Ctrl Pts',(0.0358897948611611,0.156077551916693,
2.91040309672545));
#25752=CARTESIAN_POINT('Ctrl Pts',(0.150310107632486,0.0552734215298454,
2.90250586219961));
#25753=CARTESIAN_POINT('Ctrl Pts',(0.128454879143209,-0.0956432099528824,
2.89460862767377));
#25754=CARTESIAN_POINT('Ctrl Pts',(-0.00986130107440376,-0.159846909059511,
2.88671139314794));
#25755=CARTESIAN_POINT('Ctrl Pts',(-0.139236937163761,-0.079128723602177,
2.8788141586221));
#25756=CARTESIAN_POINT('Ctrl Pts',(-0.142376292407395,0.0733298776050816,
2.87091692409627));
#25757=CARTESIAN_POINT('Ctrl Pts',(-0.0164331351694357,0.159305466665398,
2.86301968957043));
#25758=CARTESIAN_POINT('Ctrl Pts',(0.124408782797267,0.10085005811842,2.85512245504459));
#25759=CARTESIAN_POINT('Ctrl Pts',(0.152458059176653,-0.0490389624868201,
2.84722522051876));
#25760=CARTESIAN_POINT('Ctrl Pts',(0.0422843970550532,-0.154467827352683,
2.83932798599292));
#25761=CARTESIAN_POINT('Ctrl Pts',(-0.106225533663848,-0.11985163596585,
2.83143075146709));
#25762=CARTESIAN_POINT('Ctrl Pts',(-0.158428293266612,0.0234255462289395,
2.82353351694125));
#25763=CARTESIAN_POINT('Ctrl Pts',(-0.0669953162115558,0.145464459997932,
2.81563628241542));
#25764=CARTESIAN_POINT('Ctrl Pts',(0.085177553915074,0.13562100539136,2.80773904788958));
#25765=CARTESIAN_POINT('Ctrl Pts',(0.160126001452633,0.00281964289891892,
2.79984181336375));
#25766=CARTESIAN_POINT('Ctrl Pts',(0.0898994544648863,-0.132538212593453,
2.79194457883791));
#25767=CARTESIAN_POINT('Ctrl Pts',(-0.0618324205375044,-0.147732811568847,
2.78404734431207));
#25768=CARTESIAN_POINT('Ctrl Pts',(-0.157505498107873,-0.028988973955003,
2.77615010978624));
#25769=CARTESIAN_POINT('Ctrl Pts',(-0.110378936218723,0.11603798664468,
2.7682528752604));
#25770=CARTESIAN_POINT('Ctrl Pts',(0.0368193467442185,0.155859837441643,
2.76035564073457));
#25771=CARTESIAN_POINT('Ctrl Pts',(0.150638156857367,0.0543778248529476,
2.75245840620873));
#25772=CARTESIAN_POINT('Ctrl Pts',(0.127880111678472,-0.0964109210451539,
2.7445611716829));
#25773=CARTESIAN_POINT('Ctrl Pts',(-0.0108102891681236,-0.159778762376561,
2.73666393715706));
#25774=CARTESIAN_POINT('Ctrl Pts',(-0.139714188602295,-0.0783094860905571,
2.72876670263123));
#25775=CARTESIAN_POINT('Ctrl Pts',(-0.141921357082812,0.0742017060679738,
2.72086946810539));
#25776=CARTESIAN_POINT('Ctrl Pts',(-0.0155119468753121,0.159354141686116,
2.71297223357956));
#25777=CARTESIAN_POINT('Ctrl Pts',(0.125064499963334,0.100197318391729,
2.70507499905372));
#25778=CARTESIAN_POINT('Ctrl Pts',(0.152049584323474,-0.050136315469175,
2.69717776452788));
#25779=CARTESIAN_POINT('Ctrl Pts',(0.0784331561467309,-0.119531683020366,
2.69191294151066));
#25780=CARTESIAN_POINT('Ctrl Pts',(0.0350561322973247,-0.131128202024318,
2.68928053000205));
#25781=CARTESIAN_POINT('Ctrl Pts',(0.10987964471909,0.0946377159884874,
3.61071946999795));
#25782=CARTESIAN_POINT('Ctrl Pts',(0.14118566737564,0.0582896848558689,
3.60808705848934));
#25783=CARTESIAN_POINT('Ctrl Pts',(0.16438863056535,-0.0472784515007908,
3.60282223547212));
#25784=CARTESIAN_POINT('Ctrl Pts',(0.0500715609504776,-0.163726586556196,
3.59492500094628));
#25785=CARTESIAN_POINT('Ctrl Pts',(-0.109620454466532,-0.131316785248055,
3.58702776642045));
#25786=CARTESIAN_POINT('Ctrl Pts',(-0.169935896575886,0.0199399747483351,
3.57913053189461));
#25787=CARTESIAN_POINT('Ctrl Pts',(-0.0761783230800011,0.153226069048607,
3.57123329736878));
#25788=CARTESIAN_POINT('Ctrl Pts',(0.0866426147068042,0.147537162356952,
3.56333606284294));
#25789=CARTESIAN_POINT('Ctrl Pts',(0.170911927956997,0.00811571627929297,
3.55543882831711));
#25790=CARTESIAN_POINT('Ctrl Pts',(0.100226913008187,-0.138678728894576,
3.54754159379127));
#25791=CARTESIAN_POINT('Ctrl Pts',(-0.0613264554739007,-0.159735158279625,
3.53964435926544));
#25792=CARTESIAN_POINT('Ctrl Pts',(-0.167279620124009,-0.0359750850591977,
3.53174712473959));
#25793=CARTESIAN_POINT('Ctrl Pts',(-0.121572106459094,0.120403165496963,
3.52384989021377));
#25794=CARTESIAN_POINT('Ctrl Pts',(0.0343561939670442,0.167619285598691,
3.51595265568792));
#25795=CARTESIAN_POINT('Ctrl Pts',(0.159136185514944,0.0628674278258929,
3.5080554211621));
#25796=CARTESIAN_POINT('Ctrl Pts',(0.139638644047474,-0.0988821758709744,
3.50015818663625));
#25797=CARTESIAN_POINT('Ctrl Pts',(-0.00645937171612636,-0.170982151786161,
3.49226095211042));
#25798=CARTESIAN_POINT('Ctrl Pts',(-0.146701135149248,-0.0880647864625838,
3.48436371758458));
#25799=CARTESIAN_POINT('Ctrl Pts',(-0.15393935576282,0.074694732438219,
3.47646648305875));
#25800=CARTESIAN_POINT('Ctrl Pts',(-0.0216116533870178,0.169733799903276,
3.46856924853291));
#25801=CARTESIAN_POINT('Ctrl Pts',(0.130309806680585,0.110887249630166,
3.46067201400708));
#25802=CARTESIAN_POINT('Ctrl Pts',(0.164088583251082,-0.0484929312809838,
3.45277477948124));
#25803=CARTESIAN_POINT('Ctrl Pts',(0.0490998495417746,-0.16390799887602,
3.4448775449554));
#25804=CARTESIAN_POINT('Ctrl Pts',(-0.110404244360585,-0.130719280730833,
3.43698031042957));
#25805=CARTESIAN_POINT('Ctrl Pts',(-0.169812620143325,0.0209833626627134,
3.42908307590373));
#25806=CARTESIAN_POINT('Ctrl Pts',(-0.075263906229341,0.153661875119715,
3.4211858413779));
#25807=CARTESIAN_POINT('Ctrl Pts',(0.0875212671135803,0.147026036053807,
3.41328860685206));
#25808=CARTESIAN_POINT('Ctrl Pts',(0.170957099034354,0.00709209097369881,
3.40539137232623));
#25809=CARTESIAN_POINT('Ctrl Pts',(0.0993982231972585,-0.139271751220155,
3.39749413780039));
#25810=CARTESIAN_POINT('Ctrl Pts',(-0.0622779899341693,-0.15936774904703,
3.38959690327456));
#25811=CARTESIAN_POINT('Ctrl Pts',(-0.167491155293001,-0.0349762828714076,
3.38169966874872));
#25812=CARTESIAN_POINT('Ctrl Pts',(-0.120851938892729,0.121125704665286,
3.37380243422289));
#25813=CARTESIAN_POINT('Ctrl Pts',(0.0353551811322426,0.167411584522707,
3.36590519969705));
#25814=CARTESIAN_POINT('Ctrl Pts',(0.15950825953878,0.0619172238068289,
3.35800796517121));
#25815=CARTESIAN_POINT('Ctrl Pts',(0.139046483036208,-0.0997131035536944,
3.35011073064538));
#25816=CARTESIAN_POINT('Ctrl Pts',(-0.00747890313808957,-0.170940613877928,
3.34221349611955));
#25817=CARTESIAN_POINT('Ctrl Pts',(-0.14722369691345,-0.0871883623668259,
3.33431626159371));
#25818=CARTESIAN_POINT('Ctrl Pts',(-0.153491179671254,0.0756114093785092,
3.32641902706787));
#25819=CARTESIAN_POINT('Ctrl Pts',(-0.0205990681724529,0.169859665181325,
3.31852179254204));
#25820=CARTESIAN_POINT('Ctrl Pts',(0.130968761208522,0.110108178863265,
3.3106245580162));
#25821=CARTESIAN_POINT('Ctrl Pts',(0.16379647986064,-0.0494706039011429,
3.30272732349037));
#25822=CARTESIAN_POINT('Ctrl Pts',(0.0481215175972415,-0.16419788978309,
3.29483008896453));
#25823=CARTESIAN_POINT('Ctrl Pts',(-0.111181820434632,-0.130058564769576,
3.2869328544387));
#25824=CARTESIAN_POINT('Ctrl Pts',(-0.169684467159477,0.0219956602511813,
3.27903561991286));
#25825=CARTESIAN_POINT('Ctrl Pts',(-0.0743462114159517,0.154107976150411,
3.27113838538702));
#25826=CARTESIAN_POINT('Ctrl Pts',(0.0883964947808067,0.146501492059118,
3.26324115086119));
#25827=CARTESIAN_POINT('Ctrl Pts',(0.170996352549731,0.00607246900110077,
3.25534391633535));
#25828=CARTESIAN_POINT('Ctrl Pts',(0.0985659141730064,-0.139862032118515,
3.24744668180952));
#25829=CARTESIAN_POINT('Ctrl Pts',(-0.0632272657842059,-0.15899352290749,
3.23954944728368));
#25830=CARTESIAN_POINT('Ctrl Pts',(-0.167696756710366,-0.0339768340771394,
3.23165221275785));
#25831=CARTESIAN_POINT('Ctrl Pts',(-0.120127461616738,0.121844246604426,
3.22375497823201));
#25832=CARTESIAN_POINT('Ctrl Pts',(0.0363529048066224,0.167197768457601,
3.21585774370617));
#25833=CARTESIAN_POINT('Ctrl Pts',(0.159874664137553,0.0609649016400891,
3.20796050918034));
#25834=CARTESIAN_POINT('Ctrl Pts',(0.138449375430002,-0.100540528684324,
3.2000632746545));
#25835=CARTESIAN_POINT('Ctrl Pts',(-0.00849816772359493,-0.170892974140023,
3.19216604012867));
#25836=CARTESIAN_POINT('Ctrl Pts',(-0.147741023383925,-0.0863088493409087,
3.18426880560283));
#25837=CARTESIAN_POINT('Ctrl Pts',(-0.153037544712885,0.0765254034509632,
3.176371571077));
#25838=CARTESIAN_POINT('Ctrl Pts',(-0.0195857505107214,0.169979486532972,
3.16847433655116));
#25839=CARTESIAN_POINT('Ctrl Pts',(0.131623058134361,0.109325193951073,
3.16057710202532));
#25840=CARTESIAN_POINT('Ctrl Pts',(0.163498551314534,-0.0504465180476298,
3.15267986749949));
#25841=CARTESIAN_POINT('Ctrl Pts',(0.0471414743157323,-0.164481940845858,
3.14478263297365));
#25842=CARTESIAN_POINT('Ctrl Pts',(-0.111955442538922,-0.129393223744503,
3.13688539844782));
#25843=CARTESIAN_POINT('Ctrl Pts',(-0.169550279652557,0.0230071757245571,
3.12898816392198));
#25844=CARTESIAN_POINT('Ctrl Pts',(-0.0734258726175858,0.154548596549523,
3.12109092939615));
#25845=CARTESIAN_POINT('Ctrl Pts',(0.0892685787892176,0.145971738038684,
3.11319369487031));
#25846=CARTESIAN_POINT('Ctrl Pts',(0.171029524891172,0.00505263105532012,
3.10529646034447));
#25847=CARTESIAN_POINT('Ctrl Pts',(0.0977300998321875,-0.140447339070101,
3.09739922581864));
#25848=CARTESIAN_POINT('Ctrl Pts',(-0.0641742930720691,-0.158613642457959,
3.0895019912928));
#25849=CARTESIAN_POINT('Ctrl Pts',(-0.167896394298454,-0.0329761769563863,
3.08160475676697));
#25850=CARTESIAN_POINT('Ctrl Pts',(-0.119398712226798,0.122558455374011,
3.07370752224113));
#25851=CARTESIAN_POINT('Ctrl Pts',(0.0373493356562941,0.166978006309557,
3.0658102877153));
#25852=CARTESIAN_POINT('Ctrl Pts',(0.160235383085578,0.0600104113675208,
3.05791305318946));
#25853=CARTESIAN_POINT('Ctrl Pts',(0.13784734412437,-0.101364378274316,
3.05001581866363));
#25854=CARTESIAN_POINT('Ctrl Pts',(-0.00951713008727486,-0.170839256905381,
3.04211858413779));
#25855=CARTESIAN_POINT('Ctrl Pts',(-0.148253095714458,-0.0854262668981903,
3.03422134961195));
#25856=CARTESIAN_POINT('Ctrl Pts',(-0.152578467253459,0.0774366760370435,
3.02632411508612));
#25857=CARTESIAN_POINT('Ctrl Pts',(-0.0185717363175075,0.170093262874324,
3.01842688056029));
#25858=CARTESIAN_POINT('Ctrl Pts',(0.132272674126287,0.10853832108782,3.01052964603445));
#25859=CARTESIAN_POINT('Ctrl Pts',(0.163194808240755,-0.051420638155743,
3.00263241150862));
#25860=CARTESIAN_POINT('Ctrl Pts',(0.0461597545337032,-0.164760142408496,
2.99473517698277));
#25861=CARTESIAN_POINT('Ctrl Pts',(-0.112725083152171,-0.128723281085519,
2.98683794245694));
#25862=CARTESIAN_POINT('Ctrl Pts',(-0.169410062399277,0.024017872989727,
2.9789407079311));
#25863=CARTESIAN_POINT('Ctrl Pts',(-0.0725029225620513,0.154983720709736,
2.97104347340527));
#25864=CARTESIAN_POINT('Ctrl Pts',(0.0901374881235442,0.145436792799793,
2.96314623887944));
#25865=CARTESIAN_POINT('Ctrl Pts',(0.171056614879515,0.00403261342178739,
2.95524900435359));
#25866=CARTESIAN_POINT('Ctrl Pts',(0.0968908098988563,-0.141027651268038,
2.94735176982777));
#25867=CARTESIAN_POINT('Ctrl Pts',(-0.0651190381186268,-0.158228121204172,
2.93945453530192));
#25868=CARTESIAN_POINT('Ctrl Pts',(-0.168090060956955,-0.0319743470970206,
2.93155730077609));
#25869=CARTESIAN_POINT('Ctrl Pts',(-0.118665716640764,0.123268305573731,
2.92366006625025));
#25870=CARTESIAN_POINT('Ctrl Pts',(0.0383444382474168,0.166752305897243,
2.91576283172442));
#25871=CARTESIAN_POINT('Ctrl Pts',(0.160590403549885,0.0590537869267172,
2.90786559719859));
#25872=CARTESIAN_POINT('Ctrl Pts',(0.137240410538441,-0.102184623010809,
2.89996836267275));
#25873=CARTESIAN_POINT('Ctrl Pts',(-0.0105357540088883,-0.170779464111837,
2.89207112814692));
#25874=CARTESIAN_POINT('Ctrl Pts',(-0.14875989566084,-0.0845406463731019,
2.88417389362107));
#25875=CARTESIAN_POINT('Ctrl Pts',(-0.152113963683294,0.0783451946269418,
2.87627665909525));
#25876=CARTESIAN_POINT('Ctrl Pts',(-0.0175570615310977,0.170200990355554,
2.86837942456941));
#25877=CARTESIAN_POINT('Ctrl Pts',(0.132917585844673,0.10774758787922,2.86048219004357));
#25878=CARTESIAN_POINT('Ctrl Pts',(0.162885261897846,-0.0523929288553319,
2.85258495551774));
#25879=CARTESIAN_POINT('Ctrl Pts',(0.0451763922858567,-0.165032485976878,
2.8446877209919));
#25880=CARTESIAN_POINT('Ctrl Pts',(-0.113490713213303,-0.128048757924713,
2.83679048646607));
#25881=CARTESIAN_POINT('Ctrl Pts',(-0.169263823638604,0.0250277109206782,
2.82889325194023));
#25882=CARTESIAN_POINT('Ctrl Pts',(-0.0715773878139425,0.15541334312893,
2.82099601741439));
#25883=CARTESIAN_POINT('Ctrl Pts',(0.0910031798397666,0.144896656177581,
2.81309878288856));
#25884=CARTESIAN_POINT('Ctrl Pts',(0.171077644724872,0.00301248930052715,
2.80520154836272));
#25885=CARTESIAN_POINT('Ctrl Pts',(0.0960480296290492,-0.141603019127657,
2.79730431383689));
#25886=CARTESIAN_POINT('Ctrl Pts',(-0.0660613815197478,-0.157836836132188,
2.78940707931105));
#25887=CARTESIAN_POINT('Ctrl Pts',(-0.168277914911174,-0.0309716432198527,
2.78150984478522));
#25888=CARTESIAN_POINT('Ctrl Pts',(-0.11792818320716,0.123974278216523,
2.77361261025938));
#25889=CARTESIAN_POINT('Ctrl Pts',(0.0393375658179575,0.166519701078062,
2.76571537573355));
#25890=CARTESIAN_POINT('Ctrl Pts',(0.160940889343806,0.0580969368916377,
2.75781814120771));
#25891=CARTESIAN_POINT('Ctrl Pts',(0.136626332479664,-0.103004840866145,
2.74992090668187));
#25892=CARTESIAN_POINT('Ctrl Pts',(-0.011549647108527,-0.170706656610813,
2.74202367215604));
#25893=CARTESIAN_POINT('Ctrl Pts',(-0.149269788191131,-0.0836653780051494,
2.7341264376302));
#25894=CARTESIAN_POINT('Ctrl Pts',(-0.151627913553235,0.0792766508469352,
2.72622920310437));
#25895=CARTESIAN_POINT('Ctrl Pts',(-0.0165728695680367,0.170252994451239,
2.71833196857853));
#25896=CARTESIAN_POINT('Ctrl Pts',(0.133618150071337,0.107050204730652,
2.7104347340527));
#25897=CARTESIAN_POINT('Ctrl Pts',(0.162448849852474,-0.0535653340983903,
2.70253749952686));
#25898=CARTESIAN_POINT('Ctrl Pts',(0.0837975063399687,-0.127706922146391,
2.69727267650963));
#25899=CARTESIAN_POINT('Ctrl Pts',(0.0374537582415302,-0.140096572423083,
2.69464026500102));
#25900=CARTESIAN_POINT('Ctrl Pts',(0.116913659442517,0.100696009035906,
3.61607920499693));
#25901=CARTESIAN_POINT('Ctrl Pts',(0.150223756874345,0.0620211357769951,
3.61344679348832));
#25902=CARTESIAN_POINT('Ctrl Pts',(0.174912072379498,-0.0503050113773498,
3.60818197047109));
#25903=CARTESIAN_POINT('Ctrl Pts',(0.0532769234891989,-0.174207647205754,
3.60028473594526));
#25904=CARTESIAN_POINT('Ctrl Pts',(-0.11663787696255,-0.139723112036145,
3.59238750141943));
#25905=CARTESIAN_POINT('Ctrl Pts',(-0.180814450120624,0.0212164448017569,
3.58449026689359));
#25906=CARTESIAN_POINT('Ctrl Pts',(-0.0810549264538156,0.163034932450524,
3.57659303236775));
#25907=CARTESIAN_POINT('Ctrl Pts',(0.0921890963056651,0.156981846810788,
3.56869579784192));
#25908=CARTESIAN_POINT('Ctrl Pts',(0.181852962765875,0.00863524897295638,
3.56079856331608));
#25909=CARTESIAN_POINT('Ctrl Pts',(0.10664300202618,-0.147556335146073,
3.55290132879024));
#25910=CARTESIAN_POINT('Ctrl Pts',(-0.0652523071804818,-0.169960705131912,
3.54500409426442));
#25911=CARTESIAN_POINT('Ctrl Pts',(-0.177988130457198,-0.0382780528074994,
3.53710685973857));
#25912=CARTESIAN_POINT('Ctrl Pts',(-0.129354621491586,0.128110850036879,
3.52920962521275));
#25913=CARTESIAN_POINT('Ctrl Pts',(0.0365555273815534,0.178349539831362,
3.52131239068689));
#25914=CARTESIAN_POINT('Ctrl Pts',(0.169323388748115,0.0668919258489962,
3.51341515616108));
#25915=CARTESIAN_POINT('Ctrl Pts',(0.148577699872602,-0.105212180693424,
3.50551792163523));
#25916=CARTESIAN_POINT('Ctrl Pts',(-0.00687287246844015,-0.181927682017732,
3.4976206871094));
#25917=CARTESIAN_POINT('Ctrl Pts',(-0.156092300794361,-0.0937023092829102,
3.48972345258356));
#25918=CARTESIAN_POINT('Ctrl Pts',(-0.163793880663394,0.0794763628218631,
3.48182621805772));
#25919=CARTESIAN_POINT('Ctrl Pts',(-0.0229951370022999,0.180599416102118,
3.47392898353189));
#25920=CARTESIAN_POINT('Ctrl Pts',(0.138651671100891,0.117985766817156,
3.46603174900605));
#25921=CARTESIAN_POINT('Ctrl Pts',(0.174592817347261,-0.0515972368462645,
3.45813451448022));
#25922=CARTESIAN_POINT('Ctrl Pts',(0.0522430073621133,-0.174400672749591,
3.45023727995438));
#25923=CARTESIAN_POINT('Ctrl Pts',(-0.117471841660763,-0.139087357890593,
3.44234004542855));
#25924=CARTESIAN_POINT('Ctrl Pts',(-0.180683282069521,0.0223266258512126,
3.43444281090271));
#25925=CARTESIAN_POINT('Ctrl Pts',(-0.0800819726320239,0.163498636922,3.42654557637688));
#25926=CARTESIAN_POINT('Ctrl Pts',(0.0931239962001525,0.156438000435139,
3.41864834185104));
#25927=CARTESIAN_POINT('Ctrl Pts',(0.181901025498224,0.00754609564814438,
3.41075110732521));
#25928=CARTESIAN_POINT('Ctrl Pts',(0.10576126311461,-0.148187320169658,
3.40285387279937));
#25929=CARTESIAN_POINT('Ctrl Pts',(-0.0662647547190597,-0.169569775965683,
3.39495663827354));
#25930=CARTESIAN_POINT('Ctrl Pts',(-0.178213207183381,-0.0372153116680257,
3.3870594037477));
#25931=CARTESIAN_POINT('Ctrl Pts',(-0.128588351944475,0.128879643005541,
3.37916216922186));
#25932=CARTESIAN_POINT('Ctrl Pts',(0.0376184653398806,0.178128542640067,
3.37126493469602));
#25933=CARTESIAN_POINT('Ctrl Pts',(0.169719281325138,0.0658808939206553,
3.36336770017019));
#25934=CARTESIAN_POINT('Ctrl Pts',(0.14794763130091,-0.10609630073556,3.35547046564435));
#25935=CARTESIAN_POINT('Ctrl Pts',(-0.00795766983708003,-0.181883485034118,
3.34757323111852));
#25936=CARTESIAN_POINT('Ctrl Pts',(-0.156648314679315,-0.0927697803461756,
3.33967599659268));
#25937=CARTESIAN_POINT('Ctrl Pts',(-0.163317014296801,0.0804517214143475,
3.33177876206685));
#25938=CARTESIAN_POINT('Ctrl Pts',(-0.0219177305069036,0.180733338725286,
3.32388152754101));
#25939=CARTESIAN_POINT('Ctrl Pts',(0.139352809018331,0.117156823343995,
3.31598429301518));
#25940=CARTESIAN_POINT('Ctrl Pts',(0.174282014774141,-0.0526374957955154,
3.30808705848934));
#25941=CARTESIAN_POINT('Ctrl Pts',(0.0512020468814229,-0.174709121205821,
3.3001898239635));
#25942=CARTESIAN_POINT('Ctrl Pts',(-0.118299194757364,-0.13838434578057,
3.29229258943767));
#25943=CARTESIAN_POINT('Ctrl Pts',(-0.180546925291626,0.0234037263079457,
3.28439535491183));
#25944=CARTESIAN_POINT('Ctrl Pts',(-0.0791055310066521,0.163973295391393,
3.27649812038601));
#25945=CARTESIAN_POINT('Ctrl Pts',(0.0940552521182287,0.155879877425964,
3.26860088586016));
#25946=CARTESIAN_POINT('Ctrl Pts',(0.181942791852133,0.00646120193221371,
3.26070365133433));
#25947=CARTESIAN_POINT('Ctrl Pts',(0.104875673303493,-0.148815388271832,
3.25280641680849));
#25948=CARTESIAN_POINT('Ctrl Pts',(-0.067274799061048,-0.169171593503912,
3.24490918228266));
#25949=CARTESIAN_POINT('Ctrl Pts',(-0.178431970305088,-0.0361518825291525,
3.23701194775682));
#25950=CARTESIAN_POINT('Ctrl Pts',(-0.127817496798961,0.129644182859876,
3.22911471323099));
#25951=CARTESIAN_POINT('Ctrl Pts',(0.0386800589242284,0.177901039004767,
3.22121747870515));
#25952=CARTESIAN_POINT('Ctrl Pts',(0.170109141545278,0.0648676082500797,
3.21332024417931));
#25953=CARTESIAN_POINT('Ctrl Pts',(0.147312299474883,-0.106976694007524,
3.20542300965349));
#25954=CARTESIAN_POINT('Ctrl Pts',(-0.00904218328755787,-0.18183279560836,
3.19752577512764));
#25955=CARTESIAN_POINT('Ctrl Pts',(-0.157198758129913,-0.0918339647394704,
3.18962854060181));
#25956=CARTESIAN_POINT('Ctrl Pts',(-0.162834339610607,0.0814242253935201,
3.18173130607597));
#25957=CARTESIAN_POINT('Ctrl Pts',(-0.0208395446762738,0.180860830516292,
3.17383407155014));
#25958=CARTESIAN_POINT('Ctrl Pts',(0.140048991174337,0.116323715159066,
3.1659368370243));
#25959=CARTESIAN_POINT('Ctrl Pts',(0.173965014144346,-0.0536758837012937,
3.15803960249847));
#25960=CARTESIAN_POINT('Ctrl Pts',(0.050159265511441,-0.175011355976434,
3.15014236797263));
#25961=CARTESIAN_POINT('Ctrl Pts',(-0.119122340768341,-0.137676412530354,
3.14224513344679));
#25962=CARTESIAN_POINT('Ctrl Pts',(-0.180404147686861,0.0244799945819963,
3.13434789892096));
#25963=CARTESIAN_POINT('Ctrl Pts',(-0.0781262761399388,0.164442122383114,
3.12645066439512));
#25964=CARTESIAN_POINT('Ctrl Pts',(0.0949831631341886,0.155316210867962,
3.11855342986929));
#25965=CARTESIAN_POINT('Ctrl Pts',(0.181978087741923,0.00537607841744088,
3.11065619534345));
#25966=CARTESIAN_POINT('Ctrl Pts',(0.10398635378076,-0.149438164016893,
3.10275896081762));
#25967=CARTESIAN_POINT('Ctrl Pts',(-0.0682824508977375,-0.168767394767933,
3.09486172629178));
#25968=CARTESIAN_POINT('Ctrl Pts',(-0.178644387819226,-0.0350871677120128,
3.08696449176594));
#25969=CARTESIAN_POINT('Ctrl Pts',(-0.127042096057429,0.130404112154074,
3.07906725724011));
#25970=CARTESIAN_POINT('Ctrl Pts',(0.039740276922879,0.17766720864428,3.07117002271427));
#25971=CARTESIAN_POINT('Ctrl Pts',(0.170492952144154,0.0638520156810144,
3.06327278818844));
#25972=CARTESIAN_POINT('Ctrl Pts',(0.146671728755708,-0.107853282848364,
3.0553755536626));
#25973=CARTESIAN_POINT('Ctrl Pts',(-0.0101263751692898,-0.181775639631079,
3.04747831913677));
#25974=CARTESIAN_POINT('Ctrl Pts',(-0.15774361109349,-0.0908948832253125,
3.03958108461093));
#25975=CARTESIAN_POINT('Ctrl Pts',(-0.162345874018219,0.0823938336686527,
3.0316838500851));
#25976=CARTESIAN_POINT('Ctrl Pts',(-0.0197606177252597,0.180981890321858,
3.02378661555926));
#25977=CARTESIAN_POINT('Ctrl Pts',(0.140740192743497,0.115486470133437,
3.01588938103343));
#25978=CARTESIAN_POINT('Ctrl Pts',(0.173641826766224,-0.0547123627222005,
3.00799214650759));
#25979=CARTESIAN_POINT('Ctrl Pts',(0.0491147003187017,-0.175307366787479,
3.00009491198175));
#25980=CARTESIAN_POINT('Ctrl Pts',(-0.119941250410619,-0.136963583069732,
2.99219767745592));
#25981=CARTESIAN_POINT('Ctrl Pts',(-0.180254954337721,0.0255553922697266,
2.98430044293008));
#25982=CARTESIAN_POINT('Ctrl Pts',(-0.0771442428547834,0.164905101290741,
2.97640320840425));
#25983=CARTESIAN_POINT('Ctrl Pts',(0.0959076962473017,0.15474702077238,
2.96850597387841));
#25984=CARTESIAN_POINT('Ctrl Pts',(0.182006911912947,0.00429076371209153,
2.96060873935257));
#25985=CARTESIAN_POINT('Ctrl Pts',(0.103093336173269,-0.150055625266004,
2.95271150482674));
#25986=CARTESIAN_POINT('Ctrl Pts',(-0.069287674394006,-0.168357194128057,
2.9448142703009));
#25987=CARTESIAN_POINT('Ctrl Pts',(-0.178850452170956,-0.0340212050826592,
2.93691703577507));
#25988=CARTESIAN_POINT('Ctrl Pts',(-0.126262177296885,0.131159403861809,
2.92901980124923));
#25989=CARTESIAN_POINT('Ctrl Pts',(0.0407990816336726,0.177427059877793,
2.9211225667234));
#25990=CARTESIAN_POINT('Ctrl Pts',(0.170870699467283,0.0628341523235889,
2.91322533219756));
#25991=CARTESIAN_POINT('Ctrl Pts',(0.146025941933673,-0.108726036068736,
2.90532809767173));
#25992=CARTESIAN_POINT('Ctrl Pts',(-0.0112102069433731,-0.181712019164164,
2.89743086314589));
#25993=CARTESIAN_POINT('Ctrl Pts',(-0.158282854157919,-0.0899525691440268,
2.88953362862006));
#25994=CARTESIAN_POINT('Ctrl Pts',(-0.161851634959193,0.0833605116488022,
2.88163639409422));
#25995=CARTESIAN_POINT('Ctrl Pts',(-0.0186809878927599,0.181096514045709,
2.87373915956839));
#25996=CARTESIAN_POINT('Ctrl Pts',(0.14142638889208,0.114645117640021,2.86584192504255));
#25997=CARTESIAN_POINT('Ctrl Pts',(0.173312464619039,-0.0557468952238434,
2.85794469051671));
#25998=CARTESIAN_POINT('Ctrl Pts',(0.0480683875166603,-0.175597144601074,
2.85004745599088));
#25999=CARTESIAN_POINT('Ctrl Pts',(-0.120755892762759,-0.136245879883575,
2.84215022146504));
#26000=CARTESIAN_POINT('Ctrl Pts',(-0.180099354010596,0.0266298756124168,
2.83425298693921));
#26001=CARTESIAN_POINT('Ctrl Pts',(-0.0761594594163292,0.165362226259928,
2.82635575241337));
#26002=CARTESIAN_POINT('Ctrl Pts',(0.0968288057644592,0.154172306963803,
2.81845851788754));
#26003=CARTESIAN_POINT('Ctrl Pts',(0.182029287997112,0.0032053357021354,
2.8105612833617));
#26004=CARTESIAN_POINT('Ctrl Pts',(0.102196604793212,-0.150667825661861,
2.80266404883587));
#26005=CARTESIAN_POINT('Ctrl Pts',(-0.0702903425019912,-0.167940860695529,
2.79476681431002));
#26006=CARTESIAN_POINT('Ctrl Pts',(-0.179050331714475,-0.0329543124847025,
2.7868695797842));
#26007=CARTESIAN_POINT('Ctrl Pts',(-0.125477430195597,0.131910569788365,
2.77897234525835));
#26008=CARTESIAN_POINT('Ctrl Pts',(0.0418557848916964,0.17717956471448,
2.77107511073252));
#26009=CARTESIAN_POINT('Ctrl Pts',(0.171243621830244,0.0618160489303277,
2.76317787620668));
#26010=CARTESIAN_POINT('Ctrl Pts',(0.145372553280857,-0.109598760687136,
2.75528064168085));
#26011=CARTESIAN_POINT('Ctrl Pts',(-0.0122890050489303,-0.181634550845065,
2.74738340715501));
#26012=CARTESIAN_POINT('Ctrl Pts',(-0.158825387779967,-0.0890212699197419,
2.73948617262918));
#26013=CARTESIAN_POINT('Ctrl Pts',(-0.161334470023658,0.0843515956258966,
2.73158893810334));
#26014=CARTESIAN_POINT('Ctrl Pts',(-0.0176337922607613,0.181151847216363,
2.72369170357751));
#26015=CARTESIAN_POINT('Ctrl Pts',(0.14217180017934,0.113903091069576,2.71579446905167));
#26016=CARTESIAN_POINT('Ctrl Pts',(0.172848115381474,-0.0569943527276058,
2.70789723452584));
#26017=CARTESIAN_POINT('Ctrl Pts',(0.0891618565332066,-0.135882161272415,
2.70263241150861));
#26018=CARTESIAN_POINT('Ctrl Pts',(0.0398513841857358,-0.149064942821848,
2.7));
#26019=CARTESIAN_POINT('Ctrl Pts',(0.0958116152722374,0.0825211298936506,
3.6));
#26020=CARTESIAN_POINT('Ctrl Pts',(0.102493614798766,0.0762810303731869,
3.6));
#26021=CARTESIAN_POINT('Ctrl Pts',(0.108396094096263,0.0693090539021388,
3.6));
#26022=CARTESIAN_POINT('Ctrl Pts',(0.113512571306729,0.0617846659987563,
3.6));
#26023=CARTESIAN_POINT('Ctrl Pts',(0.117461600031764,0.0559771498608983,
3.6));
#26024=CARTESIAN_POINT('Ctrl Pts',(0.120942091267611,0.0498392138898472,
3.6));
#26025=CARTESIAN_POINT('Ctrl Pts',(0.123938893544148,0.0434377969520944,
3.6));
#26026=CARTESIAN_POINT('Ctrl Pts',(0.125176287448039,0.0407946214723323,
3.6));
#26027=CARTESIAN_POINT('Ctrl Pts',(0.126329312445263,0.0381097373250835,
3.6));
#26028=CARTESIAN_POINT('Ctrl Pts',(0.12739426777321,0.0353959223183902,
3.6));
#26029=CARTESIAN_POINT('Ctrl Pts',(0.130992400282108,0.0262268372474364,
3.6));
#26030=CARTESIAN_POINT('Ctrl Pts',(0.13360037697833,0.0167048680256365,
3.6));
#26031=CARTESIAN_POINT('Ctrl Pts',(0.135185783736742,0.0070125550480467,
3.6));
#26032=CARTESIAN_POINT('Ctrl Pts',(0.135855615028331,0.00291757154566029,
3.6));
#26033=CARTESIAN_POINT('Ctrl Pts',(0.13634239472836,-0.00120821237992505,
3.6));
#26034=CARTESIAN_POINT('Ctrl Pts',(0.136641151680689,-0.0053522141362822,
3.6));
#26035=CARTESIAN_POINT('Ctrl Pts',(0.136866179264237,-0.00847352962091436,
3.6));
#26036=CARTESIAN_POINT('Ctrl Pts',(0.136984148876184,-0.0116047424016575,
3.6));
#26037=CARTESIAN_POINT('Ctrl Pts',(0.136993305813875,-0.0147266162095009,
3.6));
#26038=CARTESIAN_POINT('Ctrl Pts',(0.1370171880242,-0.0228687756739225,
3.6));
#26039=CARTESIAN_POINT('Ctrl Pts',(0.1363045911537,-0.0309705737407376,
3.6));
#26040=CARTESIAN_POINT('Ctrl Pts',(0.134831565375878,-0.0389361856515032,
3.6));
#26041=CARTESIAN_POINT('Ctrl Pts',(0.133932184221546,-0.043799726631656,
3.6));
#26042=CARTESIAN_POINT('Ctrl Pts',(0.132748938308619,-0.0486126850413777,
3.6));
#26043=CARTESIAN_POINT('Ctrl Pts',(0.131298540463925,-0.0533602760289537,
3.6));
#26044=CARTESIAN_POINT('Ctrl Pts',(0.130441077796828,-0.0561670107778959,
3.6));
#26045=CARTESIAN_POINT('Ctrl Pts',(0.129489770756279,-0.058951963571448,
3.6));
#26046=CARTESIAN_POINT('Ctrl Pts',(0.128448797183808,-0.061708664264176,
3.6));
#26047=CARTESIAN_POINT('Ctrl Pts',(0.124844109667278,-0.0712545786242284,
3.6));
#26048=CARTESIAN_POINT('Ctrl Pts',(0.120197621014249,-0.0803872939153616,
3.6));
#26049=CARTESIAN_POINT('Ctrl Pts',(0.114666430721154,-0.0889848980033025,
3.6));
#26050=CARTESIAN_POINT('Ctrl Pts',(0.111763941762871,-0.0934964858552134,
3.6));
#26051=CARTESIAN_POINT('Ctrl Pts',(0.108616890563154,-0.0978607268708147,
3.6));
#26052=CARTESIAN_POINT('Ctrl Pts',(0.105242483611131,-0.102058774522217,
3.6));
#26053=CARTESIAN_POINT('Ctrl Pts',(0.103051571759935,-0.104784454169668,
3.6));
#26054=CARTESIAN_POINT('Ctrl Pts',(0.100763130867069,-0.107441777418394,
3.6));
#26055=CARTESIAN_POINT('Ctrl Pts',(0.098386472215756,-0.110019467506635,
3.6));
#26056=CARTESIAN_POINT('Ctrl Pts',(0.0926299038901994,-0.116262959438837,
3.6));
#26057=CARTESIAN_POINT('Ctrl Pts',(0.0863771877690887,-0.12201951201926,
3.6));
#26058=CARTESIAN_POINT('Ctrl Pts',(0.0796980248685607,-0.127218319244159,
3.6));
#26059=CARTESIAN_POINT('Ctrl Pts',(0.0749983795646852,-0.130876345006388,
3.6));
#26060=CARTESIAN_POINT('Ctrl Pts',(0.0700820293375014,-0.134260491890013,
3.6));
#26061=CARTESIAN_POINT('Ctrl Pts',(0.064997448628775,-0.137327043702736,
3.6));
#26062=CARTESIAN_POINT('Ctrl Pts',(0.0586168958330981,-0.141175206779031,
3.6));
#26063=CARTESIAN_POINT('Ctrl Pts',(0.0519659322704503,-0.144529310638398,
3.6));
#26064=CARTESIAN_POINT('Ctrl Pts',(0.0450857487477646,-0.147337352418514,
3.6));
#26065=CARTESIAN_POINT('Ctrl Pts',(0.0433856322299594,-0.148031228998597,
3.6));
#26066=CARTESIAN_POINT('Ctrl Pts',(0.0416714833555574,-0.148691718060548,
3.6));
#26067=CARTESIAN_POINT('Ctrl Pts',(0.0399441988940855,-0.149319076597487,
3.6));
#26068=CARTESIAN_POINT('Ctrl Pts',(-0.126474550616365,-0.00011099430647141,
3.51934196736194));
#26069=CARTESIAN_POINT('Ctrl Pts',(-0.126555547962724,-0.00903265450993761,
3.51990386315518));
#26070=CARTESIAN_POINT('Ctrl Pts',(-0.125690900286005,-0.0179387227435883,
3.52046575894841));
#26071=CARTESIAN_POINT('Ctrl Pts',(-0.123822037714229,-0.0266288110680491,
3.52102765474165));
#26072=CARTESIAN_POINT('Ctrl Pts',(-0.115066650325334,-0.0673407879000796,
3.52366006625026));
#26073=CARTESIAN_POINT('Ctrl Pts',(-0.0842707011930362,-0.103312426237565,
3.52629247775887));
#26074=CARTESIAN_POINT('Ctrl Pts',(-0.0453944787880641,-0.118238154042396,
3.52892488926748));
#26075=CARTESIAN_POINT('Ctrl Pts',(-0.00651825638309213,-0.133163881847227,
3.53155730077609));
#26076=CARTESIAN_POINT('Ctrl Pts',(0.0404382392945539,-0.127043699119404,
3.5341897122847));
#26077=CARTESIAN_POINT('Ctrl Pts',(0.0741890076945504,-0.102650246541568,
3.53682212379332));
#26078=CARTESIAN_POINT('Ctrl Pts',(0.107939776094547,-0.0782567939637322,
3.53945453530193));
#26079=CARTESIAN_POINT('Ctrl Pts',(0.128484817216894,-0.0355900715358833,
3.54208694681054));
#26080=CARTESIAN_POINT('Ctrl Pts',(0.126510636639707,0.00600514677092718,
3.54471935831915));
#26081=CARTESIAN_POINT('Ctrl Pts',(0.124536456062521,0.0476003650777378,
3.54735176982776));
#26082=CARTESIAN_POINT('Ctrl Pts',(0.100043053785802,0.0881240792635097,
3.54998418133637));
#26083=CARTESIAN_POINT('Ctrl Pts',(0.0641338913405327,0.109212694488978,
3.55261659284499));
#26084=CARTESIAN_POINT('Ctrl Pts',(0.028224728895264,0.130301309714446,
3.5552490043536));
#26085=CARTESIAN_POINT('Ctrl Pts',(-0.019100193718554,0.13195482597961,
3.55788141586221));
#26086=CARTESIAN_POINT('Ctrl Pts',(-0.0563882672178024,0.113411366178312,
3.56051382737082));
#26087=CARTESIAN_POINT('Ctrl Pts',(-0.0936763407170509,0.0948679063770136,
3.56314623887943));
#26088=CARTESIAN_POINT('Ctrl Pts',(-0.12092756510173,0.0561274705092526,
3.56577865038805));
#26089=CARTESIAN_POINT('Ctrl Pts',(-0.125787647292084,0.0147753915231441,
3.56841106189666));
#26090=CARTESIAN_POINT('Ctrl Pts',(-0.126360541139662,0.00990091600857084,
3.56872136371842));
#26091=CARTESIAN_POINT('Ctrl Pts',(-0.126622308248343,0.0049901515008091,
3.56903166554018));
#26092=CARTESIAN_POINT('Ctrl Pts',(-0.126585968300139,7.56654190205153E-5,
3.56934196736194));
#26093=CARTESIAN_POINT('Ctrl Pts',(-0.0398513841857247,-0.149064942821851,
3.6));
#26094=CARTESIAN_POINT('Ctrl Pts',(-0.0891618565331957,-0.135882161272422,
3.59736758849139));
#26095=CARTESIAN_POINT('Ctrl Pts',(-0.17284812802765,-0.0569944292149041,
3.59210276547417));
#26096=CARTESIAN_POINT('Ctrl Pts',(-0.142171789002704,0.113903133580536,
3.58420553094833));
#26097=CARTESIAN_POINT('Ctrl Pts',(0.0176337902165689,0.181151815132919,
3.5763082964225));
#26098=CARTESIAN_POINT('Ctrl Pts',(0.161334465098627,0.0843516096779105,
3.56841106189666));
#26099=CARTESIAN_POINT('Ctrl Pts',(0.158825384561566,-0.0890212772063117,
3.56051382737082));
#26100=CARTESIAN_POINT('Ctrl Pts',(0.0122890037691484,-0.181634540286447,
3.55261659284499));
#26101=CARTESIAN_POINT('Ctrl Pts',(-0.145372548664834,-0.109598761010981,
3.54471935831915));
#26102=CARTESIAN_POINT('Ctrl Pts',(-0.171243617690229,0.0618160491398297,
3.53682212379332));
#26103=CARTESIAN_POINT('Ctrl Pts',(-0.0418557834629445,0.177179558878914,
3.52892488926748));
#26104=CARTESIAN_POINT('Ctrl Pts',(0.125477426630257,0.13191056683484,3.52102765474164));
#26105=CARTESIAN_POINT('Ctrl Pts',(0.179050327003836,-0.0329543119327003,
3.51313042021581));
#26106=CARTESIAN_POINT('Ctrl Pts',(0.0702903405429243,-0.167940855985405,
3.50523318568997));
#26107=CARTESIAN_POINT('Ctrl Pts',(-0.102196602002365,-0.150667821707605,
3.49733595116413));
#26108=CARTESIAN_POINT('Ctrl Pts',(-0.182029283116568,0.00320533567306586,
3.4894387166383));
#26109=CARTESIAN_POINT('Ctrl Pts',(-0.0968288031440013,0.15417230277993,
3.48154148211247));
#26110=CARTESIAN_POINT('Ctrl Pts',(0.0761594573579975,0.165362221823523,
3.47364424758663));
#26111=CARTESIAN_POINT('Ctrl Pts',(0.180099349163956,0.0266298748857393,
3.46574701306079));
#26112=CARTESIAN_POINT('Ctrl Pts',(0.120755889508211,-0.136245876208876,
3.45784977853496));
#26113=CARTESIAN_POINT('Ctrl Pts',(-0.0480683862207756,-0.175597139874519,
3.44995254400912));
#26114=CARTESIAN_POINT('Ctrl Pts',(-0.173312459951882,-0.0557468937208932,
3.44205530948329));
#26115=CARTESIAN_POINT('Ctrl Pts',(-0.141426385082663,0.114645114551432,
3.43415807495745));
#26116=CARTESIAN_POINT('Ctrl Pts',(0.0186809873893989,0.181096509168673,
3.42626084043161));
#26117=CARTESIAN_POINT('Ctrl Pts',(0.161851630600137,0.0833605094034181,
3.41836360590578));
#26118=CARTESIAN_POINT('Ctrl Pts',(0.158282849894819,-0.0899525667211824,
3.41046637137994));
#26119=CARTESIAN_POINT('Ctrl Pts',(0.0112102066414966,-0.181712014270169,
3.40256913685411));
#26120=CARTESIAN_POINT('Ctrl Pts',(-0.146025938000753,-0.108726033140384,
3.39467190232827));
#26121=CARTESIAN_POINT('Ctrl Pts',(-0.170870694865204,0.0628341506312357,
3.38677466780244));
#26122=CARTESIAN_POINT('Ctrl Pts',(-0.0407990805348497,0.177427055099143,
3.3788774332766));
#26123=CARTESIAN_POINT('Ctrl Pts',(0.126262173896246,0.131159400329288,
3.37098019875077));
#26124=CARTESIAN_POINT('Ctrl Pts',(0.178850447353964,-0.0340212041663437,
3.36308296422493));
#26125=CARTESIAN_POINT('Ctrl Pts',(0.0692876725278909,-0.168357189593675,
3.3551857296991));
#26126=CARTESIAN_POINT('Ctrl Pts',(-0.103093333396635,-0.150055621224551,
3.34728849517326));
#26127=CARTESIAN_POINT('Ctrl Pts',(-0.18200690701094,0.00429076359651101,
3.33939126064742));
#26128=CARTESIAN_POINT('Ctrl Pts',(-0.0959076936642258,0.154747016604558,
3.33149402612159));
#26129=CARTESIAN_POINT('Ctrl Pts',(0.0771442407770374,0.164905096849345,
3.32359679159575));
#26130=CARTESIAN_POINT('Ctrl Pts',(0.180254949482897,0.0255553915814562,
3.31569955706992));
#26131=CARTESIAN_POINT('Ctrl Pts',(0.119941247180243,-0.13696357938087,
3.30780232254408));
#26132=CARTESIAN_POINT('Ctrl Pts',(-0.0491146989958762,-0.175307362065916,
3.29990508801825));
#26133=CARTESIAN_POINT('Ctrl Pts',(-0.173641822089509,-0.0547123612486432,
3.29200785349241));
#26134=CARTESIAN_POINT('Ctrl Pts',(-0.14074018895294,0.115486467023018,
3.28411061896658));
#26135=CARTESIAN_POINT('Ctrl Pts',(0.0197606171930289,0.18098188544746,
3.27621338444074));
#26136=CARTESIAN_POINT('Ctrl Pts',(0.162345869645737,0.0823938314495476,
3.26831614991491));
#26137=CARTESIAN_POINT('Ctrl Pts',(0.157743606844976,-0.0908948807772195,
3.26041891538907));
#26138=CARTESIAN_POINT('Ctrl Pts',(0.0101263748965706,-0.181775634735301,
3.25252168086324));
#26139=CARTESIAN_POINT('Ctrl Pts',(-0.146671724805377,-0.107853279943556,
3.2446244463374));
#26140=CARTESIAN_POINT('Ctrl Pts',(-0.170492947552259,0.0638520139612676,
3.23672721181156));
#26141=CARTESIAN_POINT('Ctrl Pts',(-0.0397402758525677,0.177667203859151,
3.22882997728572));
#26142=CARTESIAN_POINT('Ctrl Pts',(0.127042092635782,0.130404108641901,
3.22093274275989));
#26143=CARTESIAN_POINT('Ctrl Pts',(0.178644383007786,-0.0350871667669908,
3.21303550823405));
#26144=CARTESIAN_POINT('Ctrl Pts',(0.0682824490586963,-0.1687673902225,
3.20513827370822));
#26145=CARTESIAN_POINT('Ctrl Pts',(-0.103986350980073,-0.149438159992073,
3.19724103918238));
#26146=CARTESIAN_POINT('Ctrl Pts',(-0.181978082840693,0.00537607827262928,
3.18934380465655));
#26147=CARTESIAN_POINT('Ctrl Pts',(-0.0949831605760139,0.155316206684809,
3.18144657013072));
#26148=CARTESIAN_POINT('Ctrl Pts',(0.0781262740357409,0.164442117954189,
3.17354933560488));
#26149=CARTESIAN_POINT('Ctrl Pts',(0.180404142828019,0.0244799939226929,
3.16565210107904));
#26150=CARTESIAN_POINT('Ctrl Pts',(0.119122337560023,-0.137676408822293,
3.15775486655321));
#26151=CARTESIAN_POINT('Ctrl Pts',(-0.0501592641604809,-0.175011351262844,
3.14985763202737));
#26152=CARTESIAN_POINT('Ctrl Pts',(-0.173965009458927,-0.0536758822556528,
3.14196039750153));
#26153=CARTESIAN_POINT('Ctrl Pts',(-0.140048987402398,0.116323712026096,
3.1340631629757));
#26154=CARTESIAN_POINT('Ctrl Pts',(0.0208395441149821,0.180860825645154,
3.12616592844986));
#26155=CARTESIAN_POINT('Ctrl Pts',(0.162834335224968,0.0814242232005321,
3.11826869392403));
#26156=CARTESIAN_POINT('Ctrl Pts',(0.157198753896076,-0.0918339622660831,
3.1103714593982));
#26157=CARTESIAN_POINT('Ctrl Pts',(0.00904218304404205,-0.181832790711041,
3.10247422487235));
#26158=CARTESIAN_POINT('Ctrl Pts',(-0.147312295507299,-0.106976691126326,
3.09457699034652));
#26159=CARTESIAN_POINT('Ctrl Pts',(-0.170109136963721,0.0648676065029794,
3.08667975582068));
#26160=CARTESIAN_POINT('Ctrl Pts',(-0.0386800578824722,0.177901034213339,
3.07878252129485));
#26161=CARTESIAN_POINT('Ctrl Pts',(0.127817493356429,0.129644179368171,
3.07088528676902));
#26162=CARTESIAN_POINT('Ctrl Pts',(0.178431965499368,-0.0361518815554529,
3.06298805224317));
#26163=CARTESIAN_POINT('Ctrl Pts',(0.0672747972491473,-0.169171588947593,
3.05509081771735));
#26164=CARTESIAN_POINT('Ctrl Pts',(-0.104875670478854,-0.148815384263785,
3.0471935831915));
#26165=CARTESIAN_POINT('Ctrl Pts',(-0.181942786951853,0.00646120175817659,
3.03929634866568));
#26166=CARTESIAN_POINT('Ctrl Pts',(-0.0940552495850459,0.15587987322763,
3.03139911413983));
#26167=CARTESIAN_POINT('Ctrl Pts',(0.0791055288760802,0.163973290975094,
3.02350187961401));
#26168=CARTESIAN_POINT('Ctrl Pts',(0.180546920428939,0.0234037256776295,
3.01560464508816));
#26169=CARTESIAN_POINT('Ctrl Pts',(0.118299191571216,-0.138384342053441,
3.00770741056233));
#26170=CARTESIAN_POINT('Ctrl Pts',(-0.0512020455023775,-0.174709116500372,
2.99981017603649));
#26171=CARTESIAN_POINT('Ctrl Pts',(-0.174282010080185,-0.0526374943778417,
2.99191294151066));
#26172=CARTESIAN_POINT('Ctrl Pts',(-0.139352805265142,0.117156820188587,
2.98401570698483));
#26173=CARTESIAN_POINT('Ctrl Pts',(0.0219177299165732,0.180733333857582,
2.97611847245899));
#26174=CARTESIAN_POINT('Ctrl Pts',(0.163317009898163,0.0804517192475515,
2.96822123793315));
#26175=CARTESIAN_POINT('Ctrl Pts',(0.156648310460303,-0.0927697778475837,
2.96032400340732));
#26176=CARTESIAN_POINT('Ctrl Pts',(0.00795766962277319,-0.181883480135435,
2.95242676888148));
#26177=CARTESIAN_POINT('Ctrl Pts',(-0.147947627316214,-0.106096297878073,
2.94452953435564));
#26178=CARTESIAN_POINT('Ctrl Pts',(-0.169719276754081,0.0658808921462626,
2.93663229982981));
#26179=CARTESIAN_POINT('Ctrl Pts',(-0.0376184643267171,0.178128537842515,
2.92873506530397));
#26180=CARTESIAN_POINT('Ctrl Pts',(0.128588348481182,0.128879639534425,
2.92083783077814));
#26181=CARTESIAN_POINT('Ctrl Pts',(0.178213202383553,-0.0372153106656781,
2.9129405962523));
#26182=CARTESIAN_POINT('Ctrl Pts',(0.0662647529343645,-0.169569771398652,
2.90504336172647));
#26183=CARTESIAN_POINT('Ctrl Pts',(-0.105761260266122,-0.148187316178505,
2.89714612720063));
#26184=CARTESIAN_POINT('Ctrl Pts',(-0.181901020599063,0.00754609544484455,
2.8892488926748));
#26185=CARTESIAN_POINT('Ctrl Pts',(-0.0931239936920636,0.15643799622185,
2.88135165814895));
#26186=CARTESIAN_POINT('Ctrl Pts',(0.080081970475175,0.163498632518342,
2.87345442362313));
#26187=CARTESIAN_POINT('Ctrl Pts',(0.180683277203119,0.0223266252501708,
2.86555718909729));
#26188=CARTESIAN_POINT('Ctrl Pts',(0.11747183849698,-0.139087354145018,
2.85765995457145));
#26189=CARTESIAN_POINT('Ctrl Pts',(-0.0522430059551858,-0.174400668051551,
2.84976272004562));
#26190=CARTESIAN_POINT('Ctrl Pts',(-0.174592812644639,-0.0515972354582594,
2.84186548551978));
#26191=CARTESIAN_POINT('Ctrl Pts',(-0.138651667367148,0.117985763642445,
2.83396825099395));
#26192=CARTESIAN_POINT('Ctrl Pts',(0.0229951363840201,0.180599411232496,
2.82607101646811));
#26193=CARTESIAN_POINT('Ctrl Pts',(0.163793876249876,0.0794763606914083,
2.81817378194228));
#26194=CARTESIAN_POINT('Ctrl Pts',(0.1560922965942,-0.0937023067775016,
2.81027654741644));
#26195=CARTESIAN_POINT('Ctrl Pts',(0.00687287227597422,-0.181927677084725,
2.8023793128906));
#26196=CARTESIAN_POINT('Ctrl Pts',(-0.148577695856893,-0.105212177919503,
2.79448207836477));
#26197=CARTESIAN_POINT('Ctrl Pts',(-0.169323384214447,0.0668919241546485,
2.78658484383893));
#26198=CARTESIAN_POINT('Ctrl Pts',(-0.0365555263461618,0.178349534836247,
2.7786876093131));
#26199=CARTESIAN_POINT('Ctrl Pts',(0.129354617910885,0.128110846926664,
2.77079037478726));
#26200=CARTESIAN_POINT('Ctrl Pts',(0.177988125847537,-0.0382780523762908,
2.76289314026143));
#26201=CARTESIAN_POINT('Ctrl Pts',(0.0652523050728403,-0.169960699505811,
2.75499590573559));
#26202=CARTESIAN_POINT('Ctrl Pts',(-0.106642998487829,-0.147556332986489,
2.74709867120975));
#26203=CARTESIAN_POINT('Ctrl Pts',(-0.181852959134814,0.00863525184135577,
2.73920143668392));
#26204=CARTESIAN_POINT('Ctrl Pts',(-0.0921890914137533,0.156981837366664,
2.73130420215808));
#26205=CARTESIAN_POINT('Ctrl Pts',(0.081054919689294,0.163034936656946,
2.72340696763225));
#26206=CARTESIAN_POINT('Ctrl Pts',(0.180814453969382,0.0212164304176998,
2.71550973310641));
#26207=CARTESIAN_POINT('Ctrl Pts',(0.116637857196403,-0.139723086682139,
2.70761249858058));
#26208=CARTESIAN_POINT('Ctrl Pts',(-0.0532768903028442,-0.174207676028794,
2.69971526405474));
#26209=CARTESIAN_POINT('Ctrl Pts',(-0.17491212592378,-0.0503049553127666,
2.69181802952891));
#26210=CARTESIAN_POINT('Ctrl Pts',(-0.150223756874352,0.0620211357769783,
2.68655320651168));
#26211=CARTESIAN_POINT('Ctrl Pts',(-0.116913659442528,0.100696009035893,
2.68392079500307));
#26212=CARTESIAN_POINT('Ctrl Pts',(-0.0374537582415199,-0.140096572423086,
3.60535973499898));
#26213=CARTESIAN_POINT('Ctrl Pts',(-0.0837975063399586,-0.127706922146397,
3.60272732349037));
#26214=CARTESIAN_POINT('Ctrl Pts',(-0.162448861737804,-0.0535654059838928,
3.59746250047314));
#26215=CARTESIAN_POINT('Ctrl Pts',(-0.133618139567134,0.107050244683975,
3.5895652659473));
#26216=CARTESIAN_POINT('Ctrl Pts',(0.0165728676468313,0.170252964298069,
3.58166803142147));
#26217=CARTESIAN_POINT('Ctrl Pts',(0.151627908924514,0.0792766640535213,
3.57377079689563));
#26218=CARTESIAN_POINT('Ctrl Pts',(0.149269785166362,-0.0836653848533289,
3.5658735623698));
#26219=CARTESIAN_POINT('Ctrl Pts',(0.0115496459057422,-0.170706646687446,
3.55797632784397));
#26220=CARTESIAN_POINT('Ctrl Pts',(-0.136626328141362,-0.103004841170506,
3.55007909331813));
#26221=CARTESIAN_POINT('Ctrl Pts',(-0.160940885452871,0.0580969370885353,
3.54218185879229));
#26222=CARTESIAN_POINT('Ctrl Pts',(-0.0393375644751653,0.166519695593587,
3.53428462426645));
#26223=CARTESIAN_POINT('Ctrl Pts',(0.117928179856326,0.123974275440694,
3.52638738974062));
#26224=CARTESIAN_POINT('Ctrl Pts',(0.168277910483947,-0.0309716427010613,
3.51849015521478));
#26225=CARTESIAN_POINT('Ctrl Pts',(0.0660613796785464,-0.157836831705444,
3.51059292068895));
#26226=CARTESIAN_POINT('Ctrl Pts',(-0.0960480270061105,-0.141603015411306,
3.50269568616311));
#26227=CARTESIAN_POINT('Ctrl Pts',(-0.171077640137963,0.00301248927320663,
3.49479845163728));
#26228=CARTESIAN_POINT('Ctrl Pts',(-0.0910031773769663,0.144896652245428,
3.48690121711144));
#26229=CARTESIAN_POINT('Ctrl Pts',(0.0715773858794485,0.155413338959437,
3.47900398258561));
#26230=CARTESIAN_POINT('Ctrl Pts',(0.169263819083558,0.0250277102377205,
3.47110674805977));
#26231=CARTESIAN_POINT('Ctrl Pts',(0.113490710154562,-0.128048754471099,
3.46320951353393));
#26232=CARTESIAN_POINT('Ctrl Pts',(-0.0451763910679377,-0.165032481534694,
3.4553122790081));
#26233=CARTESIAN_POINT('Ctrl Pts',(-0.162885257511484,-0.0523929274428053,
3.44741504448226));
#26234=CARTESIAN_POINT('Ctrl Pts',(-0.132917582264447,0.107747584976454,
3.43951780995643));
#26235=CARTESIAN_POINT('Ctrl Pts',(0.0175570610580211,0.17020098577194,
3.43162057543059));
#26236=CARTESIAN_POINT('Ctrl Pts',(0.152113959586497,0.0783451925166497,
3.42372334090476));
#26237=CARTESIAN_POINT('Ctrl Pts',(0.148759891654226,-0.0845406440960262,
3.41582610637892));
#26238=CARTESIAN_POINT('Ctrl Pts',(0.0105357537251741,-0.170779459512285,
3.40792887185309));
#26239=CARTESIAN_POINT('Ctrl Pts',(-0.137240406842142,-0.102184620258639,
3.40003163732725));
#26240=CARTESIAN_POINT('Ctrl Pts',(-0.160590399224686,0.059053785336183,
3.39213440280142));
#26241=CARTESIAN_POINT('Ctrl Pts',(-0.0383444372147038,0.166752301406097,
3.38423716827558));
#26242=CARTESIAN_POINT('Ctrl Pts',(0.118665713444722,0.123268302253741,
3.37633993374974));
#26243=CARTESIAN_POINT('Ctrl Pts',(0.168090056429774,-0.0319743462358346,
3.36844269922391));
#26244=CARTESIAN_POINT('Ctrl Pts',(0.065119036364785,-0.158228116942597,
3.36054546469807));
#26245=CARTESIAN_POINT('Ctrl Pts',(-0.0968908072892766,-0.141027647469737,
3.35264823017224));
#26246=CARTESIAN_POINT('Ctrl Pts',(-0.171056610272434,0.00403261331316083,
3.3447509956464));
#26247=CARTESIAN_POINT('Ctrl Pts',(-0.090137485695877,0.145436788882724,
3.33685376112057));
#26248=CARTESIAN_POINT('Ctrl Pts',(0.0725029206093111,0.154983716535553,
3.32895652659473));
#26249=CARTESIAN_POINT('Ctrl Pts',(0.16941005783654,0.0240178723428656,
3.3210592920689));
#26250=CARTESIAN_POINT('Ctrl Pts',(0.112725080116148,-0.128723277618595,
3.31316205754306));
#26251=CARTESIAN_POINT('Ctrl Pts',(-0.0461597532904643,-0.164760137971002,
3.30526482301723));
#26252=CARTESIAN_POINT('Ctrl Pts',(-0.163194803845412,-0.0514206367708408,
3.29736758849139));
#26253=CARTESIAN_POINT('Ctrl Pts',(-0.132272670563786,0.108538318164536,
3.28947035396555));
#26254=CARTESIAN_POINT('Ctrl Pts',(0.0185717358172978,0.17009325829319,
3.28157311943971));
#26255=CARTESIAN_POINT('Ctrl Pts',(0.152578463144044,0.0774366739514488,
3.27367588491388));
#26256=CARTESIAN_POINT('Ctrl Pts',(0.148253091721553,-0.0854262645973846,
3.26577865038804));
#26257=CARTESIAN_POINT('Ctrl Pts',(0.00951712983096357,-0.170839252304153,
3.25788141586221));
#26258=CARTESIAN_POINT('Ctrl Pts',(-0.137847340411707,-0.101364375544273,
3.24998418133637));
#26259=CARTESIAN_POINT('Ctrl Pts',(-0.160235378769951,0.060010409751241,
3.24208694681054));
#26260=CARTESIAN_POINT('Ctrl Pts',(-0.0373493346503772,0.166978001812321,
3.2341897122847));
#26261=CARTESIAN_POINT('Ctrl Pts',(0.119398709011011,0.122558452073145,
3.22629247775887));
#26262=CARTESIAN_POINT('Ctrl Pts',(0.16789638977649,-0.0329761760682205,
3.21839524323303));
#26263=CARTESIAN_POINT('Ctrl Pts',(0.0641742913436723,-0.158613638185999,
3.2104980087072));
#26264=CARTESIAN_POINT('Ctrl Pts',(-0.0977300972000018,-0.14044733528743,
3.20260077418136));
#26265=CARTESIAN_POINT('Ctrl Pts',(-0.17102952028482,0.00505263091922082,
3.19470353965552));
#26266=CARTESIAN_POINT('Ctrl Pts',(-0.0892685763849535,0.145971734107207,
3.18680630512969));
#26267=CARTESIAN_POINT('Ctrl Pts',(0.0734258706399851,0.15454859238706,
3.17890907060385));
#26268=CARTESIAN_POINT('Ctrl Pts',(0.169550275086044,0.0230071751049201,
3.17101183607802));
#26269=CARTESIAN_POINT('Ctrl Pts',(0.11195543952363,-0.129393220259535,
3.16311460155218));
#26270=CARTESIAN_POINT('Ctrl Pts',(-0.0471414730460515,-0.164481936415857,
3.15521736702635));
#26271=CARTESIAN_POINT('Ctrl Pts',(-0.163498546911009,-0.0504465166889647,
3.14732013250051));
#26272=CARTESIAN_POINT('Ctrl Pts',(-0.131623054589357,0.109325191006596,
3.13942289797468));
#26273=CARTESIAN_POINT('Ctrl Pts',(0.0195857499831994,0.169979481954902,
3.13152566344884));
#26274=CARTESIAN_POINT('Ctrl Pts',(0.153037540591104,0.0765254013899147,
3.123628428923));
#26275=CARTESIAN_POINT('Ctrl Pts',(0.147741019404812,-0.0863088470163307,
3.11573119439717));
#26276=CARTESIAN_POINT('Ctrl Pts',(0.00849816749472986,-0.170892969537348,
3.10783395987133));
#26277=CARTESIAN_POINT('Ctrl Pts',(-0.138449371701125,-0.100540525976471,
3.09993672534551));
#26278=CARTESIAN_POINT('Ctrl Pts',(-0.159874659831641,0.0609648999981013,
3.09203949081965));
#26279=CARTESIAN_POINT('Ctrl Pts',(-0.0363529038275426,0.167197763954447,
3.08414225629384));
#26280=CARTESIAN_POINT('Ctrl Pts',(0.120127458381323,0.121844243322797,
3.07624502176798));
#26281=CARTESIAN_POINT('Ctrl Pts',(0.167696752193779,-0.0339768331620215,
3.06834778724216));
#26282=CARTESIAN_POINT('Ctrl Pts',(0.0632272640813166,-0.158993518625298,
3.06045055271632));
#26283=CARTESIAN_POINT('Ctrl Pts',(-0.0985659115183093,-0.139862028351609,
3.05255331819049));
#26284=CARTESIAN_POINT('Ctrl Pts',(-0.170996347944273,0.0060724688375345,
3.04465608366465));
#26285=CARTESIAN_POINT('Ctrl Pts',(-0.0883964924000305,0.146501488113373,
3.03675884913881));
#26286=CARTESIAN_POINT('Ctrl Pts',(0.0743462094135637,0.154107971999816,
3.02886161461298));
#26287=CARTESIAN_POINT('Ctrl Pts',(0.16968446258935,0.0219956596587875,
3.02096438008714));
#26288=CARTESIAN_POINT('Ctrl Pts',(0.111181817440176,-0.130058561266688,
3.01306714556131));
#26289=CARTESIAN_POINT('Ctrl Pts',(-0.048121516301165,-0.16419788536074,
3.00516991103547));
#26290=CARTESIAN_POINT('Ctrl Pts',(-0.163796475449092,-0.0494706025687624,
2.99727267650963));
#26291=CARTESIAN_POINT('Ctrl Pts',(-0.13096875768114,0.110108175897699,
2.9893754419838));
#26292=CARTESIAN_POINT('Ctrl Pts',(0.020599067617639,0.169859660606483,
2.98147820745796));
#26293=CARTESIAN_POINT('Ctrl Pts',(0.153491175537256,0.0756114073420768,
2.97358097293213));
#26294=CARTESIAN_POINT('Ctrl Pts',(0.147223692948271,-0.0871883600185597,
2.96568373840629));
#26295=CARTESIAN_POINT('Ctrl Pts',(0.00747890293667656,-0.17094060927397,
2.95778650388045));
#26296=CARTESIAN_POINT('Ctrl Pts',(-0.139046479291249,-0.0997131008681262,
2.94988926935462));
#26297=CARTESIAN_POINT('Ctrl Pts',(-0.159508255242737,0.0619172221391909,
2.94199203482878));
#26298=CARTESIAN_POINT('Ctrl Pts',(-0.0353551801800353,0.167411580013796,
2.93409480030295));
#26299=CARTESIAN_POINT('Ctrl Pts',(0.120851935637802,0.121125701403006,
2.92619756577711));
#26300=CARTESIAN_POINT('Ctrl Pts',(0.167491150781951,-0.0349762819293654,
2.91830033125128));
#26301=CARTESIAN_POINT('Ctrl Pts',(0.0622779882568489,-0.159367744754771,
2.91040309672545));
#26302=CARTESIAN_POINT('Ctrl Pts',(-0.0993982205201476,-0.139271747469127,
2.9025058621996));
#26303=CARTESIAN_POINT('Ctrl Pts',(-0.170957094429947,0.0070920907826306,
2.89460862767378));
#26304=CARTESIAN_POINT('Ctrl Pts',(-0.0875212647563887,0.147026032094007,
2.88671139314793));
#26305=CARTESIAN_POINT('Ctrl Pts',(0.0752639042022573,0.153661870981,2.8788141586221));
#26306=CARTESIAN_POINT('Ctrl Pts',(0.169812615569706,0.0209833620978328,
2.87091692409627));
#26307=CARTESIAN_POINT('Ctrl Pts',(0.110404241387148,-0.130719277210608,
2.86301968957043));
#26308=CARTESIAN_POINT('Ctrl Pts',(-0.0490998482194935,-0.163907994460633,
2.8551224550446));
#26309=CARTESIAN_POINT('Ctrl Pts',(-0.164088578831389,-0.0484929299764868,
2.84722522051876));
#26310=CARTESIAN_POINT('Ctrl Pts',(-0.130309803171479,0.110887246646458,
2.83932798599293));
#26311=CARTESIAN_POINT('Ctrl Pts',(0.0216116528059362,0.16973379532663,
2.83143075146709));
#26312=CARTESIAN_POINT('Ctrl Pts',(0.153939351614839,0.0746947304359413,
2.82353351694125));
#26313=CARTESIAN_POINT('Ctrl Pts',(0.146701131201786,-0.0880647841079112,
2.81563628241542));
#26314=CARTESIAN_POINT('Ctrl Pts',(0.00645937153523989,-0.170982147149946,
2.80773904788958));
#26315=CARTESIAN_POINT('Ctrl Pts',(-0.139638640273367,-0.0988821732639446,
2.79984181336375));
#26316=CARTESIAN_POINT('Ctrl Pts',(-0.15913618125404,0.0628674262334842,
2.79194457883791));
#26317=CARTESIAN_POINT('Ctrl Pts',(-0.0343561929939461,0.167619280904103,
2.78404734431207));
#26318=CARTESIAN_POINT('Ctrl Pts',(0.121572103093823,0.120403162573872,
2.77615010978624));
#26319=CARTESIAN_POINT('Ctrl Pts',(0.167279615791685,-0.0359750846539325,
2.7682528752604));
#26320=CARTESIAN_POINT('Ctrl Pts',(0.0613264534930637,-0.159735152992013,
2.76035564073457));
#26321=CARTESIAN_POINT('Ctrl Pts',(-0.100226909682718,-0.138678726864922,
2.75245840620873));
#26322=CARTESIAN_POINT('Ctrl Pts',(-0.170911924544395,0.00811571897511738,
2.74456117168289));
#26323=CARTESIAN_POINT('Ctrl Pts',(-0.0866426101092102,0.147537153481027,
2.73666393715706));
#26324=CARTESIAN_POINT('Ctrl Pts',(0.0761783167224614,0.153226073001953,
2.72876670263122));
#26325=CARTESIAN_POINT('Ctrl Pts',(0.169935900193086,0.0199399612296831,
2.72086946810539));
#26326=CARTESIAN_POINT('Ctrl Pts',(0.109620435889599,-0.131316761419452,
2.71297223357956));
#26327=CARTESIAN_POINT('Ctrl Pts',(-0.0500715297607526,-0.163726613645121,
2.70507499905371));
#26328=CARTESIAN_POINT('Ctrl Pts',(-0.164388680888184,-0.0472783988092873,
2.69717776452789));
#26329=CARTESIAN_POINT('Ctrl Pts',(-0.141185667375647,0.0582896848558531,
2.69191294151066));
#26330=CARTESIAN_POINT('Ctrl Pts',(-0.1098796447191,0.0946377159884756,
2.68928053000205));
#26331=CARTESIAN_POINT('Ctrl Pts',(-0.035056132297315,-0.13112820202432,
3.61071946999795));
#26332=CARTESIAN_POINT('Ctrl Pts',(-0.0784331561467214,-0.119531683020372,
3.60808705848934));
#26333=CARTESIAN_POINT('Ctrl Pts',(-0.152049595447957,-0.0501363827528818,
3.60282223547212));
#26334=CARTESIAN_POINT('Ctrl Pts',(-0.125064490131564,0.100197355787414,
3.59492500094628));
#26335=CARTESIAN_POINT('Ctrl Pts',(0.015511945077094,0.15935411346322,3.58702776642045));
#26336=CARTESIAN_POINT('Ctrl Pts',(0.141921352750402,0.074201718429132,
3.57913053189461));
#26337=CARTESIAN_POINT('Ctrl Pts',(0.139714185771159,-0.078309492500346,
3.57123329736877));
#26338=CARTESIAN_POINT('Ctrl Pts',(0.0108102880423358,-0.159778753088445,
3.56333606284294));
#26339=CARTESIAN_POINT('Ctrl Pts',(-0.127880107617888,-0.0964109213300309,
3.5554388283171));
#26340=CARTESIAN_POINT('Ctrl Pts',(-0.150638153215513,0.0543778250372407,
3.54754159379127));
#26341=CARTESIAN_POINT('Ctrl Pts',(-0.0368193454873861,0.155859832308261,
3.53964435926543));
#26342=CARTESIAN_POINT('Ctrl Pts',(0.110378933082395,0.116037984046548,
3.5317471247396));
#26343=CARTESIAN_POINT('Ctrl Pts',(0.157505493964057,-0.0289889734694223,
3.52384989021376));
#26344=CARTESIAN_POINT('Ctrl Pts',(0.0618324188141689,-0.147732807425485,
3.51595265568793));
#26345=CARTESIAN_POINT('Ctrl Pts',(-0.089899452009857,-0.132538209115007,
3.50805542116209));
#26346=CARTESIAN_POINT('Ctrl Pts',(-0.160125997159357,0.00281964287334723,
3.50015818663625));
#26347=CARTESIAN_POINT('Ctrl Pts',(-0.0851775516099315,0.135621001710926,
3.49226095211042));
#26348=CARTESIAN_POINT('Ctrl Pts',(0.0669953144008998,0.145464456095352,
3.48436371758458));
#26349=CARTESIAN_POINT('Ctrl Pts',(0.15842828900316,0.0234255455897019,
3.47646648305875));
#26350=CARTESIAN_POINT('Ctrl Pts',(0.106225530800914,-0.119851632733321,
3.46856924853291));
#26351=CARTESIAN_POINT('Ctrl Pts',(-0.0422843959151,-0.154467823194868,
3.46067201400708));
#26352=CARTESIAN_POINT('Ctrl Pts',(-0.152458055071087,-0.0490389611647173,
3.45277477948124));
#26353=CARTESIAN_POINT('Ctrl Pts',(-0.124408779446231,0.100850055401476,
3.44487754495541));
#26354=CARTESIAN_POINT('Ctrl Pts',(0.0164331347266433,0.159305462375208,
3.43698031042957));
#26355=CARTESIAN_POINT('Ctrl Pts',(0.142376288572858,0.0733298756298809,
3.42908307590374));
#26356=CARTESIAN_POINT('Ctrl Pts',(0.139236933413632,-0.0791287214708696,
3.4211858413779));
#26357=CARTESIAN_POINT('Ctrl Pts',(0.00986130080885162,-0.159846904754402,
3.41328860685207));
#26358=CARTESIAN_POINT('Ctrl Pts',(-0.128454875683531,-0.0956432073768941,
3.40539137232623));
#26359=CARTESIAN_POINT('Ctrl Pts',(-0.150310103584168,0.0552734200411303,
3.3974941378004));
#26360=CARTESIAN_POINT('Ctrl Pts',(-0.0358897938945578,0.15607754771305,
3.38959690327456));
#26361=CARTESIAN_POINT('Ctrl Pts',(0.111069252993198,0.115377204178194,
3.38169966874872));
#26362=CARTESIAN_POINT('Ctrl Pts',(0.157329665505583,-0.0299274883053255,
3.37380243422289));
#26363=CARTESIAN_POINT('Ctrl Pts',(0.060950400201679,-0.14809904429152,
3.36590519969705));
#26364=CARTESIAN_POINT('Ctrl Pts',(-0.090688281181918,-0.131999673714922,
3.35800796517121));
#26365=CARTESIAN_POINT('Ctrl Pts',(-0.160106313533927,0.00377446302981049,
3.35011073064538));
#26366=CARTESIAN_POINT('Ctrl Pts',(-0.0843672777275282,0.13612656116089,
3.34221349611954));
#26367=CARTESIAN_POINT('Ctrl Pts',(0.0678616004415848,0.145062336221761,
3.33431626159371));
#26368=CARTESIAN_POINT('Ctrl Pts',(0.158565166190183,0.0224803531042752,
3.32641902706787));
#26369=CARTESIAN_POINT('Ctrl Pts',(0.105508913052052,-0.12048297585632,
3.31852179254204));
#26370=CARTESIAN_POINT('Ctrl Pts',(-0.0432048075850524,-0.154212913876088,
3.3106245580162));
#26371=CARTESIAN_POINT('Ctrl Pts',(-0.152747785601314,-0.0481289122930385,
3.30272732349037));
#26372=CARTESIAN_POINT('Ctrl Pts',(-0.123805152174632,0.101590169306055,
3.29483008896453));
#26373=CARTESIAN_POINT('Ctrl Pts',(0.0173828544415669,0.159204631138919,
3.28693285443869));
#26374=CARTESIAN_POINT('Ctrl Pts',(0.142811056642351,0.0724795164533502,
3.27903561991286));
#26375=CARTESIAN_POINT('Ctrl Pts',(0.13876257659813,-0.0799576484175498,
3.27113838538702));
#26376=CARTESIAN_POINT('Ctrl Pts',(0.00890788476535658,-0.159902869873006,
3.26324115086119));
#26377=CARTESIAN_POINT('Ctrl Pts',(-0.129022956018037,-0.0948754711449903,
3.25534391633535));
#26378=CARTESIAN_POINT('Ctrl Pts',(-0.149977809987643,0.0561688055412144,
3.24744668180951));
#26379=CARTESIAN_POINT('Ctrl Pts',(-0.0349583934481866,0.156288799765492,
3.23954944728368));
#26380=CARTESIAN_POINT('Ctrl Pts',(0.111755325386239,0.11471279550439,3.23165221275784));
#26381=CARTESIAN_POINT('Ctrl Pts',(0.157148396545194,-0.0308651853694504,
3.22375497823201));
#26382=CARTESIAN_POINT('Ctrl Pts',(0.0600661336286481,-0.148459886149497,
3.21585774370617));
#26383=CARTESIAN_POINT('Ctrl Pts',(-0.0914738434199304,-0.131456510582787,
3.20796050918034));
#26384=CARTESIAN_POINT('Ctrl Pts',(-0.160080957728948,0.00472918356581254,
3.2000632746545));
#26385=CARTESIAN_POINT('Ctrl Pts',(-0.0835539921938928,0.136627261529605,
3.19216604012867));
#26386=CARTESIAN_POINT('Ctrl Pts',(0.0687254672442293,0.144655066819931,
3.18426880560283));
#26387=CARTESIAN_POINT('Ctrl Pts',(0.158696407344068,0.0215343562871474,
3.176371571077));
#26388=CARTESIAN_POINT('Ctrl Pts',(0.104788541487236,-0.121110031696776,
3.16847433655116));
#26389=CARTESIAN_POINT('Ctrl Pts',(-0.0441236819316221,-0.15395252156887,
3.16057710202533));
#26390=CARTESIAN_POINT('Ctrl Pts',(-0.153032084363091,-0.0472171511222767,
3.15267986749949));
#26391=CARTESIAN_POINT('Ctrl Pts',(-0.123197121776316,0.102326669987095,
3.14478263297366));
#26392=CARTESIAN_POINT('Ctrl Pts',(0.0183319558514166,0.159098138264651,
3.13688539844782));
#26393=CARTESIAN_POINT('Ctrl Pts',(0.143240745957241,0.0716265795792973,
3.12898816392198));
#26394=CARTESIAN_POINT('Ctrl Pts',(0.138283284913549,-0.0807837317665782,
3.12109092939615));
#26395=CARTESIAN_POINT('Ctrl Pts',(0.00795415194541781,-0.159953148363655,
3.11319369487031));
#26396=CARTESIAN_POINT('Ctrl Pts',(-0.12958644789495,-0.0941043608266151,
3.10529646034448));
#26397=CARTESIAN_POINT('Ctrl Pts',(-0.149640182699562,0.0570621934932236,
3.09739922581864));
#26398=CARTESIAN_POINT('Ctrl Pts',(-0.0340257497726133,0.156494493695554,
3.08950199129281));
#26399=CARTESIAN_POINT('Ctrl Pts',(0.112437423406217,0.114044307277423,
3.08160475676696));
#26400=CARTESIAN_POINT('Ctrl Pts',(0.156961538888189,-0.0318017847685902,
3.07370752224114));
#26401=CARTESIAN_POINT('Ctrl Pts',(0.0591797309134862,-0.148815448303003,
3.06581028771529));
#26402=CARTESIAN_POINT('Ctrl Pts',(-0.0922561525577649,-0.130908672439433,
3.05791305318946));
#26403=CARTESIAN_POINT('Ctrl Pts',(-0.160049908936692,0.00568373591689232,
3.05001581866362));
#26404=CARTESIAN_POINT('Ctrl Pts',(-0.0827377352150154,0.137123102999116,
3.04211858413779));
#26405=CARTESIAN_POINT('Ctrl Pts',(0.0695868899510474,0.144242653024537,
3.03422134961195));
#26406=CARTESIAN_POINT('Ctrl Pts',(0.15882200474976,0.0205875936399453,
3.02632411508612));
#26407=CARTESIAN_POINT('Ctrl Pts',(0.104064443309136,-0.121732780479934,
3.01842688056028));
#26408=CARTESIAN_POINT('Ctrl Pts',(-0.0450409870999527,-0.153686654221109,
3.01052964603445));
#26409=CARTESIAN_POINT('Ctrl Pts',(-0.153310940817998,-0.0463037107596828,
3.00263241150861));
#26410=CARTESIAN_POINT('Ctrl Pts',(-0.122584710097139,0.103059531606811,
2.99473517698278));
#26411=CARTESIAN_POINT('Ctrl Pts',(0.019280405318705,0.158985987355384,
2.98683794245694));
#26412=CARTESIAN_POINT('Ctrl Pts',(0.143665341176349,0.0707710954366019,
2.97894070793111));
#26413=CARTESIAN_POINT('Ctrl Pts',(0.13779907543624,-0.0816069421895357,
2.97104347340527));
#26414=CARTESIAN_POINT('Ctrl Pts',(0.00700013625057968,-0.159997738412506,
2.96314623887943));
#26415=CARTESIAN_POINT('Ctrl Pts',(-0.130145331266283,-0.0933299038581796,
2.9552490043536));
#26416=CARTESIAN_POINT('Ctrl Pts',(-0.149297233731393,0.0579535521321195,
2.94735176982776));
#26417=CARTESIAN_POINT('Ctrl Pts',(-0.0330918960333533,0.156694622185077,
2.93945453530193));
#26418=CARTESIAN_POINT('Ctrl Pts',(0.113115522794421,0.113371763271587,
2.93155730077609));
#26419=CARTESIAN_POINT('Ctrl Pts',(0.156769099180348,-0.0327372531930529,
2.92366006625026));
#26420=CARTESIAN_POINT('Ctrl Pts',(0.0582912235793329,-0.14916571811089,
2.91576283172442));
#26421=CARTESIAN_POINT('Ctrl Pts',(-0.0930351807741731,-0.130356178759748,
2.90786559719858));
#26422=CARTESIAN_POINT('Ctrl Pts',(-0.160013168260831,0.00663808612041647,
2.89996836267275));
#26423=CARTESIAN_POINT('Ctrl Pts',(-0.0819185358207136,0.137614067966164,
2.89207112814691));
#26424=CARTESIAN_POINT('Ctrl Pts',(0.0704458379293395,0.143825109443657,
2.88417389362108));
#26425=CARTESIAN_POINT('Ctrl Pts',(0.158941953936293,0.0196400989454948,
2.87627665909524));
#26426=CARTESIAN_POINT('Ctrl Pts',(0.103336644277317,-0.122351200276197,
2.86837942456941));
#26427=CARTESIAN_POINT('Ctrl Pts',(-0.0459566904838012,-0.153415320869716,
2.86048219004357));
#26428=CARTESIAN_POINT('Ctrl Pts',(-0.15358434501814,-0.0453886244947142,
2.85258495551773));
#26429=CARTESIAN_POINT('Ctrl Pts',(-0.12196793897581,0.103788729650472,
2.8446877209919));
#26430=CARTESIAN_POINT('Ctrl Pts',(0.0202281692278525,0.158868179420765,
2.83679048646607));
#26431=CARTESIAN_POINT('Ctrl Pts',(0.144084826979801,0.0699131001804741,
2.82889325194023));
#26432=CARTESIAN_POINT('Ctrl Pts',(0.137309965809371,-0.0824272614383206,
2.8209960174144));
#26433=CARTESIAN_POINT('Ctrl Pts',(0.00604587079450571,-0.160036617215166,
2.81309878288855));
#26434=CARTESIAN_POINT('Ctrl Pts',(-0.13069958468984,-0.0925521686083858,
2.80520154836272));
#26435=CARTESIAN_POINT('Ctrl Pts',(-0.148948978293633,0.0588429283123199,
2.79730431383689));
#26436=CARTESIAN_POINT('Ctrl Pts',(-0.0321568596417307,0.156889026971959,
2.78940707931105));
#26437=CARTESIAN_POINT('Ctrl Pts',(0.113789588276761,0.11269547822108,2.78150984478522));
#26438=CARTESIAN_POINT('Ctrl Pts',(0.156571105735832,-0.0336721169315741,
2.77361261025938));
#26439=CARTESIAN_POINT('Ctrl Pts',(0.0574006019132872,-0.149509606478216,
2.76571537573355));
#26440=CARTESIAN_POINT('Ctrl Pts',(-0.0938108208776064,-0.129801120743354,
2.75781814120771));
#26441=CARTESIAN_POINT('Ctrl Pts',(-0.159970889953977,0.00759618610887905,
2.74992090668187));
#26442=CARTESIAN_POINT('Ctrl Pts',(-0.0810961288046671,0.138092469595389,
2.74202367215604));
#26443=CARTESIAN_POINT('Ctrl Pts',(0.0713017137556289,0.143417209346961,
2.7341264376302));
#26444=CARTESIAN_POINT('Ctrl Pts',(0.15905734641679,0.0186634920416663,
2.72622920310437));
#26445=CARTESIAN_POINT('Ctrl Pts',(0.102603014582794,-0.122910436156766,
2.71833196857853));
#26446=CARTESIAN_POINT('Ctrl Pts',(-0.046866169218661,-0.153245551261449,
2.7104347340527));
#26447=CARTESIAN_POINT('Ctrl Pts',(-0.153865235852588,-0.044251842305808,
2.70253749952686));
#26448=CARTESIAN_POINT('Ctrl Pts',(-0.132147577876941,0.0545582339347279,
2.69727267650964));
#26449=CARTESIAN_POINT('Ctrl Pts',(-0.102845629995673,0.0885794229410579,
2.69464026500102));
#26450=CARTESIAN_POINT('Ctrl Pts',(-0.0326585063531101,-0.122159831625555,
3.61607920499693));
#26451=CARTESIAN_POINT('Ctrl Pts',(-0.0730688059534842,-0.111356443894347,
3.61344679348832));
#26452=CARTESIAN_POINT('Ctrl Pts',(-0.14165032915811,-0.0467073595218706,
3.60818197047109));
#26453=CARTESIAN_POINT('Ctrl Pts',(-0.116510840695994,0.0933444668908538,
3.60028473594526));
#26454=CARTESIAN_POINT('Ctrl Pts',(0.0144510225073566,0.148455262628371,
3.59238750141942));
#26455=CARTESIAN_POINT('Ctrl Pts',(0.132214796576289,0.0691267728047427,
3.58449026689359));
#26456=CARTESIAN_POINT('Ctrl Pts',(0.130158586375956,-0.0729536001473631,
3.57659303236775));
#26457=CARTESIAN_POINT('Ctrl Pts',(0.0100709301789295,-0.148850859489444,
3.56869579784192));
#26458=CARTESIAN_POINT('Ctrl Pts',(-0.119133887094416,-0.0898170014895561,
3.56079856331608));
#26459=CARTESIAN_POINT('Ctrl Pts',(-0.140335420978156,0.0506587129859461,
3.55290132879025));
#26460=CARTESIAN_POINT('Ctrl Pts',(-0.0343011264996069,0.145199969022934,
3.54500409426441));
#26461=CARTESIAN_POINT('Ctrl Pts',(0.102829686308464,0.108101692652402,
3.53710685973857));
#26462=CARTESIAN_POINT('Ctrl Pts',(0.146733077444168,-0.0270063042377832,
3.52920962521274));
#26463=CARTESIAN_POINT('Ctrl Pts',(0.0576034579497911,-0.137628783145524,
3.5213123906869));
#26464=CARTESIAN_POINT('Ctrl Pts',(-0.0837508770136032,-0.123473402818708,
3.51341515616107));
#26465=CARTESIAN_POINT('Ctrl Pts',(-0.149174354180752,0.00262679647348802,
3.50551792163523));
#26466=CARTESIAN_POINT('Ctrl Pts',(-0.0793519258428967,0.126345351176423,
3.4976206871094));
#26467=CARTESIAN_POINT('Ctrl Pts',(0.062413242922351,0.135515573231267,
3.48972345258356));
#26468=CARTESIAN_POINT('Ctrl Pts',(0.147592758922763,0.0218233809416831,
3.48182621805773));
#26469=CARTESIAN_POINT('Ctrl Pts',(0.0989603514472664,-0.111654510995544,
3.47392898353189));
#26470=CARTESIAN_POINT('Ctrl Pts',(-0.0393924007622622,-0.143903164855042,
3.46603174900606));
#26471=CARTESIAN_POINT('Ctrl Pts',(-0.14203085263069,-0.0456849948866295,
3.45813451448022));
#26472=CARTESIAN_POINT('Ctrl Pts',(-0.115899976628015,0.0939525258264977,
3.45023727995438));
#26473=CARTESIAN_POINT('Ctrl Pts',(0.0153092083952656,0.148409938978475,
3.44234004542855));
#26474=CARTESIAN_POINT('Ctrl Pts',(0.132638617559218,0.0683145587431124,
3.43444281090271));
#26475=CARTESIAN_POINT('Ctrl Pts',(0.129713975173039,-0.0737167988457132,
3.42654557637688));
#26476=CARTESIAN_POINT('Ctrl Pts',(0.00918684789252914,-0.148914349996519,
3.41864834185104));
#26477=CARTESIAN_POINT('Ctrl Pts',(-0.11966934452492,-0.0891017944951492,
3.4107511073252));
#26478=CARTESIAN_POINT('Ctrl Pts',(-0.140029807943649,0.0514930547460776,
3.40285387279937));
#26479=CARTESIAN_POINT('Ctrl Pts',(-0.0334351505744119,0.145402794020004,
3.39495663827353));
#26480=CARTESIAN_POINT('Ctrl Pts',(0.103472792541674,0.107486106102647,
3.3870594037477));
#26481=CARTESIAN_POINT('Ctrl Pts',(0.146569274581392,-0.0278806303748164,
3.37916216922186));
#26482=CARTESIAN_POINT('Ctrl Pts',(0.0567817640385731,-0.137969971640442,
3.37126493469603));
#26483=CARTESIAN_POINT('Ctrl Pts',(-0.0844857550745595,-0.122971699960107,
3.36336770017019));
#26484=CARTESIAN_POINT('Ctrl Pts',(-0.14915601679542,0.00351631274646034,
3.35547046564435));
#26485=CARTESIAN_POINT('Ctrl Pts',(-0.0785970697591793,0.126816333439056,
3.34757323111852));
#26486=CARTESIAN_POINT('Ctrl Pts',(0.0632202802738586,0.13514095590797,
3.33967599659268));
#26487=CARTESIAN_POINT('Ctrl Pts',(0.147720274543826,0.0209428338656845,
3.33177876206685));
#26488=CARTESIAN_POINT('Ctrl Pts',(0.0982927459879567,-0.112242674094044,
3.32388152754101));
#26489=CARTESIAN_POINT('Ctrl Pts',(-0.0402498618796406,-0.143665689781173,
3.31598429301518));
#26490=CARTESIAN_POINT('Ctrl Pts',(-0.142300767357216,-0.0448371878152361,
3.30808705848934));
#26491=CARTESIAN_POINT('Ctrl Pts',(-0.115337633785478,0.0946420204475735,
3.30018982396351));
#26492=CARTESIAN_POINT('Ctrl Pts',(0.0161939730658361,0.148316003984649,
3.29229258943767));
#26493=CARTESIAN_POINT('Ctrl Pts',(0.133043650140658,0.0675223589552513,
3.28439535491184));
#26494=CARTESIAN_POINT('Ctrl Pts',(0.129272061474707,-0.0744890322377149,
3.276498120386));
#26495=CARTESIAN_POINT('Ctrl Pts',(0.00829863969974947,-0.148966487441859,
3.26860088586017));
#26496=CARTESIAN_POINT('Ctrl Pts',(-0.120198571624367,-0.0883865667457073,
3.26070365133432));
#26497=CARTESIAN_POINT('Ctrl Pts',(-0.139720241205335,0.0523272013311878,
3.2528064168085));
#26498=CARTESIAN_POINT('Ctrl Pts',(-0.032567452245996,0.145599597718663,
3.24490918228265));
#26499=CARTESIAN_POINT('Ctrl Pts',(0.104111941761468,0.106867138935634,
3.23701194775683));
#26500=CARTESIAN_POINT('Ctrl Pts',(0.146400403313899,-0.0287541946706802,
3.22911471323098));
#26501=CARTESIAN_POINT('Ctrl Pts',(0.0559579759136239,-0.138306134112995,
3.22121747870515));
#26502=CARTESIAN_POINT('Ctrl Pts',(-0.085217589639859,-0.122465685878144,
3.21332024417931));
#26503=CARTESIAN_POINT('Ctrl Pts',(-0.149132395173076,0.00440573621240416,
3.20542300965348));
#26504=CARTESIAN_POINT('Ctrl Pts',(-0.077839408002832,0.127282788952003,
3.19752577512764));
#26505=CARTESIAN_POINT('Ctrl Pts',(0.0640250638484733,0.134761541252801,
3.18962854060181));
#26506=CARTESIAN_POINT('Ctrl Pts',(0.147842539602093,0.0200615374693747,
3.18173130607597));
#26507=CARTESIAN_POINT('Ctrl Pts',(0.0976216434508421,-0.112826843134018,
3.17383407155013));
#26508=CARTESIAN_POINT('Ctrl Pts',(-0.0411058908171925,-0.143423106721883,
3.1659368370243));
#26509=CARTESIAN_POINT('Ctrl Pts',(-0.142565621815174,-0.0439877855555886,
3.15803960249846));
#26510=CARTESIAN_POINT('Ctrl Pts',(-0.114771188963274,0.0953281489675947,
3.15014236797263));
#26511=CARTESIAN_POINT('Ctrl Pts',(0.0170781617196339,0.148216794574399,
3.14224513344679));
#26512=CARTESIAN_POINT('Ctrl Pts',(0.133443951323378,0.0667277577686799,
3.13434789892096));
#26513=CARTESIAN_POINT('Ctrl Pts',(0.128825550422286,-0.0752586165168258,
3.12645066439512));
#26514=CARTESIAN_POINT('Ctrl Pts',(0.00741013639610572,-0.149013327189962,
3.11855342986929));
#26515=CARTESIAN_POINT('Ctrl Pts',(-0.120723524088775,-0.0876681956767594,
3.11065619534345));
#26516=CARTESIAN_POINT('Ctrl Pts',(-0.139405705567482,0.0531594869883457,
3.10275896081762));
#26517=CARTESIAN_POINT('Ctrl Pts',(-0.0316985957176838,0.145791223436661,
3.09486172629178));
#26518=CARTESIAN_POINT('Ctrl Pts',(0.104747388431111,0.106244371232049,
3.08696449176594));
#26519=CARTESIAN_POINT('Ctrl Pts',(0.1462263255826,-0.0296267363751589,
3.07906725724011));
#26520=CARTESIAN_POINT('Ctrl Pts',(0.0551321977456556,-0.138637377980708,
3.07117002271428));
#26521=CARTESIAN_POINT('Ctrl Pts',(-0.0859463935972202,-0.121955316527256,
3.06327278818844));
#26522=CARTESIAN_POINT('Ctrl Pts',(-0.149103469929111,0.00529500299625034,
3.0553755536626));
#26523=CARTESIAN_POINT('Ctrl Pts',(-0.0770789780300003,0.127744717884859,
3.04747831913677));
#26524=CARTESIAN_POINT('Ctrl Pts',(0.064827570488531,0.134377334049259,
3.03958108461093));
#26525=CARTESIAN_POINT('Ctrl Pts',(0.147959546910171,0.0191795276211033,
3.0316838500851));
#26526=CARTESIAN_POINT('Ctrl Pts',(0.096947069178096,-0.11340699969318,
3.02378661555926));
#26527=CARTESIAN_POINT('Ctrl Pts',(-0.0419604578987403,-0.143175423081478,
3.01588938103343));
#26528=CARTESIAN_POINT('Ctrl Pts',(-0.142825406186904,-0.0431368189506033,
3.00799214650759));
#26529=CARTESIAN_POINT('Ctrl Pts',(-0.114200662513138,0.0960108873159227,
3.00009491198175));
#26530=CARTESIAN_POINT('Ctrl Pts',(0.0179617430197712,0.148112314104285,
2.99219767745592));
#26531=CARTESIAN_POINT('Ctrl Pts',(0.133839506815442,0.065930783531127,
2.98430044293008));
#26532=CARTESIAN_POINT('Ctrl Pts',(0.128374457924208,-0.0760255243605117,
2.97640320840425));
#26533=CARTESIAN_POINT('Ctrl Pts',(0.00652136956448273,-0.149054867551042,
2.96850597387841));
#26534=CARTESIAN_POINT('Ctrl Pts',(-0.121244183241318,-0.0869467068482327,
2.96060873935258));
#26535=CARTESIAN_POINT('Ctrl Pts',(-0.139086212220049,0.0539898821250478,
2.95271150482674));
#26536=CARTESIAN_POINT('Ctrl Pts',(-0.0308286118866713,0.145977664356358,
2.9448142703009));
#26537=CARTESIAN_POINT('Ctrl Pts',(0.10537910995104,0.105617825140169,2.93691703577507));
#26538=CARTESIAN_POINT('Ctrl Pts',(0.146047047578745,-0.0304982244567401,
2.92901980124923));
#26539=CARTESIAN_POINT('Ctrl Pts',(0.0543044589018171,-0.138963691467009,
2.9211225667234));
#26540=CARTESIAN_POINT('Ctrl Pts',(-0.0866721410281989,-0.121440610050369,
2.91322533219756));
#26541=CARTESIAN_POINT('Ctrl Pts',(-0.149069242091714,0.0061840814582022,
2.90532809767173));
#26542=CARTESIAN_POINT('Ctrl Pts',(-0.0763158068850386,0.128202103838321,
2.89743086314589));
#26543=CARTESIAN_POINT('Ctrl Pts',(0.0656277716564218,0.133988347906315,
2.88953362862006));
#26544=CARTESIAN_POINT('Ctrl Pts',(0.14807129230288,0.0182968357931569,
2.88163639409422));
#26545=CARTESIAN_POINT('Ctrl Pts',(0.0962690471674858,-0.113983123341786,
2.87373915956838));
#26546=CARTESIAN_POINT('Ctrl Pts',(-0.0428135327481091,-0.142922647278798,
2.86584192504255));
#26547=CARTESIAN_POINT('Ctrl Pts',(-0.14308011120489,-0.0422843190129418,
2.85794469051671));
#26548=CARTESIAN_POINT('Ctrl Pts',(-0.113626074780142,0.0966902126544859,
2.85004745599088));
#26549=CARTESIAN_POINT('Ctrl Pts',(0.0188446856497688,0.1480025635149,2.84215022146504));
#26550=CARTESIAN_POINT('Ctrl Pts',(0.134230302344763,0.0651314699250072,
2.8342529869392));
#26551=CARTESIAN_POINT('Ctrl Pts',(0.127918800416957,-0.0767897387687304,
2.82635575241337));
#26552=CARTESIAN_POINT('Ctrl Pts',(0.00563237005377145,-0.149091087280386,
2.81845851788753));
#26553=CARTESIAN_POINT('Ctrl Pts',(-0.121760529106313,-0.0862221639528271,
2.8105612833617));
#26554=CARTESIAN_POINT('Ctrl Pts',(-0.138761775333226,0.0548184303911556,
2.80266404883586));
#26555=CARTESIAN_POINT('Ctrl Pts',(-0.0299575262895149,0.146158773039815,
2.79476681431003));
#26556=CARTESIAN_POINT('Ctrl Pts',(0.106007073459698,0.104987793868287,
2.7868695797842));
#26557=CARTESIAN_POINT('Ctrl Pts',(0.145862595679981,-0.0313691492092156,
2.77897234525835));
#26558=CARTESIAN_POINT('Ctrl Pts',(0.0534747503335104,-0.139284059964419,
2.77107511073252));
#26559=CARTESIAN_POINT('Ctrl Pts',(-0.0873947320724949,-0.120923514621786,
2.76317787620668));
#26560=CARTESIAN_POINT('Ctrl Pts',(-0.149029855363559,0.00707665324264049,
2.75528064168085));
#26561=CARTESIAN_POINT('Ctrl Pts',(-0.0755496475001239,0.128647785709752,
2.74738340715502));
#26562=CARTESIAN_POINT('Ctrl Pts',(0.0664251107887961,0.133608345691969,
2.73948617262918));
#26563=CARTESIAN_POINT('Ctrl Pts',(0.148178792640495,0.0173870228536497,
2.73158893810334));
#26564=CARTESIAN_POINT('Ctrl Pts',(0.0955855932759896,-0.114504110894079,
2.72369170357751));
#26565=CARTESIAN_POINT('Ctrl Pts',(-0.0436608086765693,-0.142764488877777,
2.71579446905167));
#26566=CARTESIAN_POINT('Ctrl Pts',(-0.143341790816993,-0.0412252858023288,
2.70789723452584));
#26567=CARTESIAN_POINT('Ctrl Pts',(-0.123109488378236,0.0508267830136028,
2.70263241150861));
#26568=CARTESIAN_POINT('Ctrl Pts',(-0.0958116152722464,0.0825211298936403,
2.7));
#26569=CARTESIAN_POINT('Ctrl Pts',(-0.126320239448181,8.84447983197572E-5,
3.55565803263806));
#26570=CARTESIAN_POINT('Ctrl Pts',(-0.126416389705588,0.0147241557759941,
3.55473913135546));
#26571=CARTESIAN_POINT('Ctrl Pts',(-0.124064907197002,0.029329993953288,
3.55382023007285));
#26572=CARTESIAN_POINT('Ctrl Pts',(-0.119129449584441,0.0430029699128602,
3.55290132879025));
#26573=CARTESIAN_POINT('Ctrl Pts',(-0.104990656151973,0.0821724649982754,
3.55026891728164));
#26574=CARTESIAN_POINT('Ctrl Pts',(-0.0696458913257897,0.113686217010605,
3.54763650577302));
#26575=CARTESIAN_POINT('Ctrl Pts',(-0.0291183734446862,0.123260046955014,
3.54500409426441));
#26576=CARTESIAN_POINT('Ctrl Pts',(0.011409144436417,0.132833876899423,
3.5423716827558));
#26577=CARTESIAN_POINT('Ctrl Pts',(0.0571194153724406,0.120467784775912,
3.53973927124719));
#26578=CARTESIAN_POINT('Ctrl Pts',(0.0872917826964029,0.0917667392324598,
3.53710685973857));
#26579=CARTESIAN_POINT('Ctrl Pts',(0.117464150020365,0.0630656936890069,
3.53447444822996));
#26580=CARTESIAN_POINT('Ctrl Pts',(0.132098613732267,0.0180296947256118,
3.53184203672135));
#26581=CARTESIAN_POINT('Ctrl Pts',(0.124560909005821,-0.0229253845740426,
3.52920962521274));
#26582=CARTESIAN_POINT('Ctrl Pts',(0.117023204279375,-0.0638804638736969,
3.52657721370413));
#26583=CARTESIAN_POINT('Ctrl Pts',(0.0873133311145834,-0.100754623509611,
3.52394480219552));
#26584=CARTESIAN_POINT('Ctrl Pts',(0.048899338704955,-0.116832473273098,
3.5213123906869));
#26585=CARTESIAN_POINT('Ctrl Pts',(0.0104853462953266,-0.132910323036586,
3.51867997917829));
#26586=CARTESIAN_POINT('Ctrl Pts',(-0.0366327653591382,-0.128191862927647,
3.51604756766968));
#26587=CARTESIAN_POINT('Ctrl Pts',(-0.0710957340475621,-0.104815932991145,
3.51341515616107));
#26588=CARTESIAN_POINT('Ctrl Pts',(-0.104947268304411,-0.0818547336764444,
3.51082944832006));
#26589=CARTESIAN_POINT('Ctrl Pts',(-0.126588725667586,-0.0408922251827605,
3.50824374047906));
#26590=CARTESIAN_POINT('Ctrl Pts',(-0.12665116202208,1.34725138570783E-5,
3.50565803263806));
#26591=CARTESIAN_POINT('Ctrl Pts',(-0.0398513841857247,-0.149064942821851,
3.6));
#26592=CARTESIAN_POINT('Ctrl Pts',(-0.0498814435786606,-0.145400000402268,
3.6));
#26593=CARTESIAN_POINT('Ctrl Pts',(-0.059436150936811,-0.14063603073288,
3.6));
#26594=CARTESIAN_POINT('Ctrl Pts',(-0.0684043669488933,-0.134923276476459,
3.6));
#26595=CARTESIAN_POINT('Ctrl Pts',(-0.0756266237179617,-0.130322698385691,
3.6));
#26596=CARTESIAN_POINT('Ctrl Pts',(-0.0824683814027756,-0.125105404214097,
3.6));
#26597=CARTESIAN_POINT('Ctrl Pts',(-0.0888542192956036,-0.119334036703677,
3.6));
#26598=CARTESIAN_POINT('Ctrl Pts',(-0.091539386939335,-0.116907246428204,
3.6));
#26599=CARTESIAN_POINT('Ctrl Pts',(-0.0941378270474737,-0.114387469535812,
3.6));
#26600=CARTESIAN_POINT('Ctrl Pts',(-0.0966394276056281,-0.111785621852247,
3.6));
#26601=CARTESIAN_POINT('Ctrl Pts',(-0.103848676908048,-0.104287474901247,
3.6));
#26602=CARTESIAN_POINT('Ctrl Pts',(-0.110272002565724,-0.0960958678941195,
3.6));
#26603=CARTESIAN_POINT('Ctrl Pts',(-0.115776223647425,-0.0873309061633839,
3.6));
#26604=CARTESIAN_POINT('Ctrl Pts',(-0.118162872674894,-0.0835303888731155,
3.6));
#26605=CARTESIAN_POINT('Ctrl Pts',(-0.120376124201495,-0.0796218141710604,
3.6));
#26606=CARTESIAN_POINT('Ctrl Pts',(-0.122402049312502,-0.0756142631648066,
3.6));
#26607=CARTESIAN_POINT('Ctrl Pts',(-0.123825086107396,-0.0727993059344893,
3.6));
#26608=CARTESIAN_POINT('Ctrl Pts',(-0.125154691418473,-0.0699368314187636,
3.6));
#26609=CARTESIAN_POINT('Ctrl Pts',(-0.126381872197889,-0.0670411886576404,
3.6));
#26610=CARTESIAN_POINT('Ctrl Pts',(-0.129549149387792,-0.0595677149679855,
3.6));
#26611=CARTESIAN_POINT('Ctrl Pts',(-0.132046086846552,-0.0518539539453467,
3.6));
#26612=CARTESIAN_POINT('Ctrl Pts',(-0.133799060139059,-0.0439576297154888,
3.6));
#26613=CARTESIAN_POINT('Ctrl Pts',(-0.135388531616607,-0.0367978046374413,
3.6));
#26614=CARTESIAN_POINT('Ctrl Pts',(-0.136365840160023,-0.0294873792206846,
3.6));
#26615=CARTESIAN_POINT('Ctrl Pts',(-0.13674259160829,-0.0221011370783161,
3.6));
#26616=CARTESIAN_POINT('Ctrl Pts',(-0.136915659814306,-0.0187081211187088,
3.6));
#26617=CARTESIAN_POINT('Ctrl Pts',(-0.136961265679344,-0.0153067045798101,
3.6));
#26618=CARTESIAN_POINT('Ctrl Pts',(-0.136881936917631,-0.0119112232715221,
3.6));
#26619=CARTESIAN_POINT('Ctrl Pts',(-0.136684990383263,-0.0034813894794369,
3.6));
#26620=CARTESIAN_POINT('Ctrl Pts',(-0.135720534319688,0.00492632812693493,
3.6));
#26621=CARTESIAN_POINT('Ctrl Pts',(-0.134014244604164,0.0131981027910972,
3.6));
#26622=CARTESIAN_POINT('Ctrl Pts',(-0.133007067351581,0.0180807104774909,
3.6));
#26623=CARTESIAN_POINT('Ctrl Pts',(-0.131740913976379,0.0229158302155836,
3.6));
#26624=CARTESIAN_POINT('Ctrl Pts',(-0.130217237780107,0.0276776331326924,
3.6));
#26625=CARTESIAN_POINT('Ctrl Pts',(-0.129150755329031,0.0310106111361586,
3.6));
#26626=CARTESIAN_POINT('Ctrl Pts',(-0.127957851528495,0.0343071390648417,
3.6));
#26627=CARTESIAN_POINT('Ctrl Pts',(-0.126644351454204,0.0375455932808108,
3.6));
#26628=CARTESIAN_POINT('Ctrl Pts',(-0.12454778430103,0.0427147111736446,
3.6));
#26629=CARTESIAN_POINT('Ctrl Pts',(-0.122141614879321,0.0477447959908898,
3.6));
#26630=CARTESIAN_POINT('Ctrl Pts',(-0.11942949850221,0.0525991124010946,
3.6));
#26631=CARTESIAN_POINT('Ctrl Pts',(-0.116867678035268,0.0571844197417489,
3.6));
#26632=CARTESIAN_POINT('Ctrl Pts',(-0.11402973916396,0.0616160698651957,
3.6));
#26633=CARTESIAN_POINT('Ctrl Pts',(-0.110933547566151,0.0658375038383711,
3.6));
#26634=CARTESIAN_POINT('Ctrl Pts',(-0.107383747559623,0.0706774001665366,
3.6));
#26635=CARTESIAN_POINT('Ctrl Pts',(-0.103491800365401,0.0752476578095535,
3.6));
#26636=CARTESIAN_POINT('Ctrl Pts',(-0.0992594032733973,0.0794964740507377,
3.6));
#26637=CARTESIAN_POINT('Ctrl Pts',(-0.0981916513129811,0.080568368245057,
3.6));
#26638=CARTESIAN_POINT('Ctrl Pts',(-0.0971022039419119,0.081619760070457,
3.6));
#26639=CARTESIAN_POINT('Ctrl Pts',(-0.0959917963302726,0.0826503396631628,
3.6));
#26640=CARTESIAN_POINT('Origin',(0.,0.,3.1));
#26641=CARTESIAN_POINT('Origin',(0.,0.,2.6));
#26642=CARTESIAN_POINT('Origin',(4.61329551933804E-18,0.,1.7));
#26643=CARTESIAN_POINT('Ctrl Pts',(0.163512932725146,-0.0319230454628286,
1.7));
#26644=CARTESIAN_POINT('Ctrl Pts',(0.162868713265022,-0.0402193660776135,
1.7));
#26645=CARTESIAN_POINT('Ctrl Pts',(0.161556142957416,-0.0484298106643142,
1.7));
#26646=CARTESIAN_POINT('Ctrl Pts',(0.159633648446255,-0.0565030284772356,
1.7));
#26647=CARTESIAN_POINT('Ctrl Pts',(0.15857220935963,-0.0609603774536462,
1.7));
#26648=CARTESIAN_POINT('Ctrl Pts',(0.15732455882578,-0.0653759608776499,
1.7));
#26649=CARTESIAN_POINT('Ctrl Pts',(0.155898537051345,-0.0697413060244838,
1.7));
#26650=CARTESIAN_POINT('Ctrl Pts',(0.154359565759251,-0.0744524128122629,
1.7));
#26651=CARTESIAN_POINT('Ctrl Pts',(0.152615240924071,-0.0790971028454583,
1.7));
#26652=CARTESIAN_POINT('Ctrl Pts',(0.150679159438777,-0.0836586618069671,
1.7));
#26653=CARTESIAN_POINT('Ctrl Pts',(0.147458757270998,-0.0912461804520635,
1.7));
#26654=CARTESIAN_POINT('Ctrl Pts',(0.143706663154478,-0.098609365081655,
1.7));
#26655=CARTESIAN_POINT('Ctrl Pts',(0.139465780840256,-0.105699927668597,
1.7));
#26656=CARTESIAN_POINT('Ctrl Pts',(0.137613322919106,-0.108797153164702,
1.7));
#26657=CARTESIAN_POINT('Ctrl Pts',(0.135667748856481,-0.111841429389798,
1.7));
#26658=CARTESIAN_POINT('Ctrl Pts',(0.133638504154441,-0.114820282936825,
1.7));
#26659=CARTESIAN_POINT('Ctrl Pts',(0.126764362615545,-0.124911259587064,
1.7));
#26660=CARTESIAN_POINT('Ctrl Pts',(0.118918297697151,-0.134279562536914,
1.7));
#26661=CARTESIAN_POINT('Ctrl Pts',(0.110233695412878,-0.142776634038112,
1.7));
#26662=CARTESIAN_POINT('Ctrl Pts',(0.1060042704444,-0.146914731004415,1.7));
#26663=CARTESIAN_POINT('Ctrl Pts',(0.101575189643516,-0.150846009251356,
1.7));
#26664=CARTESIAN_POINT('Ctrl Pts',(0.0969579219100265,-0.154551255269456,
1.7));
#26665=CARTESIAN_POINT('Ctrl Pts',(0.0930558717128837,-0.157682556460965,
1.7));
#26666=CARTESIAN_POINT('Ctrl Pts',(0.089014879864356,-0.160654885938173,
1.7));
#26667=CARTESIAN_POINT('Ctrl Pts',(0.084867234382875,-0.163439189909414,
1.7));
#26668=CARTESIAN_POINT('Ctrl Pts',(0.0797924645177416,-0.166845870145637,
1.7));
#26669=CARTESIAN_POINT('Ctrl Pts',(0.0745525511585738,-0.169976381556328,
1.7));
#26670=CARTESIAN_POINT('Ctrl Pts',(0.069162704388918,-0.172812601917057,
1.7));
#26671=CARTESIAN_POINT('Ctrl Pts',(0.0615917910053332,-0.176796533113158,
1.7));
#26672=CARTESIAN_POINT('Ctrl Pts',(0.0537253644412386,-0.180200415745643,
1.7));
#26673=CARTESIAN_POINT('Ctrl Pts',(0.0456302879589726,-0.183039981733068,
1.7));
#26674=CARTESIAN_POINT('Ctrl Pts',(0.039725979220554,-0.185111076961087,
1.7));
#26675=CARTESIAN_POINT('Ctrl Pts',(0.0336998028892366,-0.186881755092485,
1.7));
#26676=CARTESIAN_POINT('Ctrl Pts',(0.027575472779275,-0.188354488495274,
1.7));
#26677=CARTESIAN_POINT('Ctrl Pts',(0.0240503901388611,-0.189202174178265,
1.7));
#26678=CARTESIAN_POINT('Ctrl Pts',(0.0204971902089821,-0.189949869388286,
1.7));
#26679=CARTESIAN_POINT('Ctrl Pts',(0.0169287682122467,-0.190597281499825,
1.7));
#26680=CARTESIAN_POINT('Ctrl Pts',(0.00540716645046445,-0.192687624102725,
1.7));
#26681=CARTESIAN_POINT('Ctrl Pts',(-0.00629626416002409,-0.193741044106324,
1.7));
#26682=CARTESIAN_POINT('Ctrl Pts',(-0.0180243092057446,-0.193790924616578,
1.7));
#26683=CARTESIAN_POINT('Ctrl Pts',(-0.0246815057039127,-0.193819238317361,
1.7));
#26684=CARTESIAN_POINT('Ctrl Pts',(-0.0313470218059255,-0.19352361589825,
1.7));
#26685=CARTESIAN_POINT('Ctrl Pts',(-0.0379937712674718,-0.192905366089908,
1.7));
#26686=CARTESIAN_POINT('Ctrl Pts',(-0.0421040672802865,-0.192523045417697,
1.7));
#26687=CARTESIAN_POINT('Ctrl Pts',(-0.0462092418665425,-0.192016959216387,
1.7));
#26688=CARTESIAN_POINT('Ctrl Pts',(-0.0502964475671879,-0.191387744025229,
1.7));
#26689=CARTESIAN_POINT('Ctrl Pts',(-0.0635557644152557,-0.189346505047739,
1.7));
#26690=CARTESIAN_POINT('Ctrl Pts',(-0.076538642829352,-0.186027878905466,
1.7));
#26691=CARTESIAN_POINT('Ctrl Pts',(-0.0890304894083597,-0.181464562959599,
1.7));
#26692=CARTESIAN_POINT('Ctrl Pts',(-0.0993708472336289,-0.177687193500922,
1.7));
#26693=CARTESIAN_POINT('Ctrl Pts',(-0.109375752092602,-0.173056097632409,
1.7));
#26694=CARTESIAN_POINT('Ctrl Pts',(-0.118921685270779,-0.167562801749516,
1.7));
#26695=CARTESIAN_POINT('Ctrl Pts',(-0.120076087508369,-0.166898490263086,
1.7));
#26696=CARTESIAN_POINT('Ctrl Pts',(-0.121223766120909,-0.16622153952215,
1.7));
#26697=CARTESIAN_POINT('Ctrl Pts',(-0.122364641233049,-0.165532117868825,
1.7));
#26698=CARTESIAN_POINT('Ctrl Pts',(-0.188262750966375,-0.0823232180103074,
1.7));
#26699=CARTESIAN_POINT('Ctrl Pts',(-0.190918693248964,-0.0742705707004131,
1.7));
#26700=CARTESIAN_POINT('Ctrl Pts',(-0.193028471001937,-0.0660604959755095,
1.7));
#26701=CARTESIAN_POINT('Ctrl Pts',(-0.194604369739905,-0.0577442961437627,
1.7));
#26702=CARTESIAN_POINT('Ctrl Pts',(-0.195791431603972,-0.0514800334494749,
1.7));
#26703=CARTESIAN_POINT('Ctrl Pts',(-0.196675380086104,-0.0451554970342283,
1.7));
#26704=CARTESIAN_POINT('Ctrl Pts',(-0.197258353741452,-0.0387928833243269,
1.7));
#26705=CARTESIAN_POINT('Ctrl Pts',(-0.197694864529353,-0.0340287752070089,
1.7));
#26706=CARTESIAN_POINT('Ctrl Pts',(-0.197962173616876,-0.0292446940334784,
1.7));
#26707=CARTESIAN_POINT('Ctrl Pts',(-0.198061149421263,-0.0244622127102265,
1.7));
#26708=CARTESIAN_POINT('Ctrl Pts',(-0.198268317226716,-0.0144519261913088,
1.7));
#26709=CARTESIAN_POINT('Ctrl Pts',(-0.197740578304783,-0.00443368324017007,
1.7));
#26710=CARTESIAN_POINT('Ctrl Pts',(-0.196485470149517,0.00550410801291526,
1.7));
#26711=CARTESIAN_POINT('Ctrl Pts',(-0.19583094903621,0.0106865252950324,
1.7));
#26712=CARTESIAN_POINT('Ctrl Pts',(-0.194977340636945,0.0158499464463904,
1.7));
#26713=CARTESIAN_POINT('Ctrl Pts',(-0.193930228257619,0.0209568152791792,
1.7));
#26714=CARTESIAN_POINT('Ctrl Pts',(-0.191365358848382,0.0334659326431063,
1.7));
#26715=CARTESIAN_POINT('Ctrl Pts',(-0.187640262305008,0.0456682931313192,
1.7));
#26716=CARTESIAN_POINT('Ctrl Pts',(-0.18276823303275,0.0573755743540122,
1.7));
#26717=CARTESIAN_POINT('Ctrl Pts',(-0.180530605205125,0.0627524998168591,
1.7));
#26718=CARTESIAN_POINT('Ctrl Pts',(-0.178050427357818,0.0680246443278264,
1.7));
#26719=CARTESIAN_POINT('Ctrl Pts',(-0.175326059031915,0.0731713030262629,
1.7));
#26720=CARTESIAN_POINT('Ctrl Pts',(-0.173546095954943,0.0765338668785476,
1.7));
#26721=CARTESIAN_POINT('Ctrl Pts',(-0.171660782837765,0.0798445731517242,
1.7));
#26722=CARTESIAN_POINT('Ctrl Pts',(-0.169672721187811,0.0830915804684565,
1.7));
#26723=CARTESIAN_POINT('Ctrl Pts',(-0.165401890376176,0.0900669269795776,
1.7));
#26724=CARTESIAN_POINT('Ctrl Pts',(-0.160674569826176,0.0967219627994757,
1.7));
#26725=CARTESIAN_POINT('Ctrl Pts',(-0.15549277623518,0.103004446710986,
1.7));
#26726=CARTESIAN_POINT('Ctrl Pts',(-0.149788864011586,0.109919955047648,
1.7));
#26727=CARTESIAN_POINT('Ctrl Pts',(-0.143534087392955,0.116384355174537,
1.7));
#26728=CARTESIAN_POINT('Ctrl Pts',(-0.1368007840805,0.122364607652698,1.7));
#26729=CARTESIAN_POINT('Ctrl Pts',(-0.132573081040691,0.126119485519849,
1.7));
#26730=CARTESIAN_POINT('Ctrl Pts',(-0.128156557788873,0.129683253321797,
1.7));
#26731=CARTESIAN_POINT('Ctrl Pts',(-0.123568264594465,0.133044997940945,
1.7));
#26732=CARTESIAN_POINT('Ctrl Pts',(-0.120777285576228,0.135089888774893,
1.7));
#26733=CARTESIAN_POINT('Ctrl Pts',(-0.117925900172203,0.137057490795076,
1.7));
#26734=CARTESIAN_POINT('Ctrl Pts',(-0.115025210475747,0.138941543144738,
1.7));
#26735=CARTESIAN_POINT('Ctrl Pts',(-0.106405133477763,0.144540444792911,
1.7));
#26736=CARTESIAN_POINT('Ctrl Pts',(-0.0973325886051703,0.149416450333531,
1.7));
#26737=CARTESIAN_POINT('Ctrl Pts',(-0.0879171639429846,0.15351829690281,
1.7));
#26738=CARTESIAN_POINT('Ctrl Pts',(-0.0791136675584941,0.157353555825057,
1.7));
#26739=CARTESIAN_POINT('Ctrl Pts',(-0.0700097444331976,0.160511945106675,
1.7));
#26740=CARTESIAN_POINT('Ctrl Pts',(-0.0606944403481407,0.162929898574301,
1.7));
#26741=CARTESIAN_POINT('Ctrl Pts',(-0.0571572012739495,0.163848052121106,
1.7));
#26742=CARTESIAN_POINT('Ctrl Pts',(-0.0535976091548405,0.16465702786045,
1.7));
#26743=CARTESIAN_POINT('Ctrl Pts',(-0.0500249348171965,0.165353504526832,
1.7));
#26744=CARTESIAN_POINT('Ctrl Pts',(-0.0389427731093366,0.16751392171383,
1.7));
#26745=CARTESIAN_POINT('Ctrl Pts',(-0.0277208597802445,0.168598940439913,
1.7));
#26746=CARTESIAN_POINT('Ctrl Pts',(-0.016510036378599,0.168511954471149,
1.7));
#26747=CARTESIAN_POINT('Ctrl Pts',(-0.0103145529256217,0.168463883057408,
1.7));
#26748=CARTESIAN_POINT('Ctrl Pts',(-0.00412256070196868,0.168057036314866,
1.7));
#26749=CARTESIAN_POINT('Ctrl Pts',(0.00203815650313415,0.16726854038896,
1.7));
#26750=CARTESIAN_POINT('Ctrl Pts',(0.00311390584534565,0.167130857722252,
1.7));
#26751=CARTESIAN_POINT('Ctrl Pts',(0.00418869523159273,0.166981526327298,
1.7));
#26752=CARTESIAN_POINT('Ctrl Pts',(0.00526237188779194,0.16682061735739,
1.7));
#26753=CARTESIAN_POINT('Origin',(0.,0.,0.645407471946233));
#26754=CARTESIAN_POINT('Ctrl Pts',(0.205654271051376,0.000148184871923513,
0.820407471946232));
#26755=CARTESIAN_POINT('Ctrl Pts',(0.20573642152142,0.00997667026911825,
0.820941869468311));
#26756=CARTESIAN_POINT('Ctrl Pts',(0.200629007389055,0.0878566204334846,
0.825180863342659));
#26757=CARTESIAN_POINT('Ctrl Pts',(0.101090873180113,0.220844643128561,
0.833124453569275));
#26758=CARTESIAN_POINT('Ctrl Pts',(-0.130696704329673,0.204681987270635,
0.844238242626078));
#26759=CARTESIAN_POINT('Ctrl Pts',(-0.242858579725743,0.00121498249237738,
0.855352031682883));
#26760=CARTESIAN_POINT('Ctrl Pts',(-0.132727951496213,-0.203386773400678,
0.866465820739686));
#26761=CARTESIAN_POINT('Ctrl Pts',(0.0988894015246068,-0.221814471640749,
0.877579609796491));
#26762=CARTESIAN_POINT('Ctrl Pts',(0.200212227802606,-0.0892608439806378,
0.885560160198673));
#26763=CARTESIAN_POINT('Ctrl Pts',(0.205725385245381,-0.0106740336596208,
0.889836114248587));
#26764=CARTESIAN_POINT('Ctrl Pts',(0.205635165348036,-0.000160487501855345,
0.890407471946233));
#26765=CARTESIAN_POINT('Ctrl Pts',(0.205269394176581,-0.000252214316689755,
0.814592528053767));
#26766=CARTESIAN_POINT('Ctrl Pts',(0.204912576919524,0.0467765744646069,
0.817137544740381));
#26767=CARTESIAN_POINT('Ctrl Pts',(0.165648098003252,0.162976258711784,
0.823387157779263));
#26768=CARTESIAN_POINT('Ctrl Pts',(-0.0272119409517698,0.241262826763902,
0.833341367170412));
#26769=CARTESIAN_POINT('Ctrl Pts',(-0.217470922739143,0.108102090643486,
0.844455156227217));
#26770=CARTESIAN_POINT('Ctrl Pts',(-0.208759451561279,-0.124141896006793,
0.85556894528402));
#26771=CARTESIAN_POINT('Ctrl Pts',(-0.00892472216375234,-0.242686445659381,
0.866682734340826));
#26772=CARTESIAN_POINT('Ctrl Pts',(0.172122246966409,-0.152544606240875,
0.87635726193074));
#26773=CARTESIAN_POINT('Ctrl Pts',(0.20498850808804,-0.0417917950361515,
0.882327193168388));
#26774=CARTESIAN_POINT('Ctrl Pts',(0.205205445749305,0.000116004416325009,
0.884592528053768));
#26775=CARTESIAN_POINT('Ctrl Pts',(-0.126907087985236,0.107935865304854,
0.8));
#26776=CARTESIAN_POINT('Ctrl Pts',(-0.162798331100657,0.0657362393039544,
0.803704596352268));
#26777=CARTESIAN_POINT('Ctrl Pts',(-0.188554427056889,-0.0565517713871986,
0.811113789056805));
#26778=CARTESIAN_POINT('Ctrl Pts',(-0.0544936724634594,-0.189356862721456,
0.822227578113607));
#26779=CARTESIAN_POINT('Ctrl Pts',(0.12941144825895,-0.14834225030535,0.833341367170414));
#26780=CARTESIAN_POINT('Ctrl Pts',(0.194879695227305,0.0282018585329969,
0.844455156227216));
#26781=CARTESIAN_POINT('Ctrl Pts',(0.0819649080024663,0.179061771725117,
0.855568945284021));
#26782=CARTESIAN_POINT('Ctrl Pts',(-0.105969441252334,0.165957021921342,
0.866682734340825));
#26783=CARTESIAN_POINT('Ctrl Pts',(-0.196910764727139,0.000985112949166876,
0.877796523397629));
#26784=CARTESIAN_POINT('Ctrl Pts',(-0.107616385055452,-0.164906857031527,
0.888910312454434));
#26785=CARTESIAN_POINT('Ctrl Pts',(0.0801799454629491,-0.179848112789142,
0.900024101511237));
#26786=CARTESIAN_POINT('Ctrl Pts',(0.194586948216313,-0.0301773643334041,
0.911137890568042));
#26787=CARTESIAN_POINT('Ctrl Pts',(0.13088616131906,0.147117686303235,0.922251679624846));
#26788=CARTESIAN_POINT('Ctrl Pts',(-0.0526161354638876,0.18975288262963,
0.93336546868165));
#26789=CARTESIAN_POINT('Ctrl Pts',(-0.187958327447607,0.0587058278606146,
0.944479257738454));
#26790=CARTESIAN_POINT('Ctrl Pts',(-0.151260109468812,-0.126075710016806,
0.955593046795258));
#26791=CARTESIAN_POINT('Ctrl Pts',(0.0238881910101356,-0.195458525846084,
0.966706835852062));
#26792=CARTESIAN_POINT('Ctrl Pts',(0.177171365146215,-0.0859360381031547,
0.977820624908868));
#26793=CARTESIAN_POINT('Ctrl Pts',(0.168287576475019,0.102244733060238,
0.98893441396567));
#26794=CARTESIAN_POINT('Ctrl Pts',(0.00536826212740452,0.196839712751384,
1.00004820302248));
#26795=CARTESIAN_POINT('Ctrl Pts',(-0.162464684252001,0.111265085550637,
1.01116199207928));
#26796=CARTESIAN_POINT('Ctrl Pts',(-0.181591862229106,-0.076151743861926,
1.02227578113608));
#26797=CARTESIAN_POINT('Ctrl Pts',(-0.0345059495415616,-0.193866014541413,
1.03338957019289));
#26798=CARTESIAN_POINT('Ctrl Pts',(0.144163650203206,-0.134132525587662,
1.04450335924969));
#26799=CARTESIAN_POINT('Ctrl Pts',(0.190878625928487,0.0483739862822188,
1.0556171483065));
#26800=CARTESIAN_POINT('Ctrl Pts',(0.062880230662697,0.186603239345861,
1.0667309373633));
#26801=CARTESIAN_POINT('Ctrl Pts',(-0.122673152855754,0.154032431506053,
1.07784472642011));
#26802=CARTESIAN_POINT('Ctrl Pts',(-0.195942408348395,-0.019526007891641,
1.08895851547691));
#26803=CARTESIAN_POINT('Ctrl Pts',(-0.0898633553462809,-0.175212070745787,
1.10007230453371));
#26804=CARTESIAN_POINT('Ctrl Pts',(0.0984686459264395,-0.170524538248248,
1.11118609359052));
#26805=CARTESIAN_POINT('Ctrl Pts',(0.196671178871044,-0.00975396199037572,
1.12229988264732));
#26806=CARTESIAN_POINT('Ctrl Pts',(0.114858351392768,0.159944526283292,
1.13341367170412));
#26807=CARTESIAN_POINT('Ctrl Pts',(-0.0720856276979479,0.183243975761544,
1.14452746076093));
#26808=CARTESIAN_POINT('Ctrl Pts',(-0.193048814249935,0.0388181360941049,
1.15564124981773));
#26809=CARTESIAN_POINT('Ctrl Pts',(-0.13731223179659,-0.141138383766243,
1.16675503887454));
#26810=CARTESIAN_POINT('Ctrl Pts',(0.0441077936468435,-0.191909340348063,
1.17786882793134));
#26811=CARTESIAN_POINT('Ctrl Pts',(0.185155455348894,-0.0670235013089116,
1.18898261698815));
#26812=CARTESIAN_POINT('Ctrl Pts',(0.156728228964436,0.119209708576257,
1.20009640604495));
#26813=CARTESIAN_POINT('Ctrl Pts',(-0.0151541228101832,0.196328920271653,
1.21121019510176));
#26814=CARTESIAN_POINT('Ctrl Pts',(-0.173165734117196,0.0937460447209521,
1.22232398415856));
#26815=CARTESIAN_POINT('Ctrl Pts',(-0.172676785153749,-0.0946436487152594,
1.23343777321536));
#26816=CARTESIAN_POINT('Ctrl Pts',(-0.0141348164511399,-0.196404937150434,
1.24455156227217));
#26817=CARTESIAN_POINT('Ctrl Pts',(0.157344910048918,-0.118394559228326,
1.25566535132897));
#26818=CARTESIAN_POINT('Ctrl Pts',(0.184805055968556,0.0679837014410847,
1.26677914038578));
#26819=CARTESIAN_POINT('Ctrl Pts',(0.0431110383282961,0.192135709193865,
1.27789292944258));
#26820=CARTESIAN_POINT('Ctrl Pts',(-0.138043001606285,0.140423723354349,
1.28900671849938));
#26821=CARTESIAN_POINT('Ctrl Pts',(-0.192844716656512,-0.0398196889847226,
1.30012050755619));
#26822=CARTESIAN_POINT('Ctrl Pts',(-0.0711334755432105,-0.183615688410121,
1.31123429661299));
#26823=CARTESIAN_POINT('Ctrl Pts',(0.115687042443292,-0.159346165890141,
1.32234808566979));
#26824=CARTESIAN_POINT('Ctrl Pts',(0.196617898501115,0.0107747093774004,
1.3334618747266));
#26825=CARTESIAN_POINT('Ctrl Pts',(0.0975821622623196,0.171033370958511,
1.3445756637834));
#26826=CARTESIAN_POINT('Ctrl Pts',(-0.0907716337523168,0.174743248450528,
1.35568945284021));
#26827=CARTESIAN_POINT('Ctrl Pts',(-0.196041123972824,0.0185086489133565,
1.36680324189701));
#26828=CARTESIAN_POINT('Ctrl Pts',(-0.121871950164007,-0.1546671268781,
1.37791703095382));
#26829=CARTESIAN_POINT('Ctrl Pts',(0.0638480017529153,-0.186274327390575,
1.38903082001062));
#26830=CARTESIAN_POINT('Ctrl Pts',(0.191127153577756,-0.0473825235535316,
1.40014460906743));
#26831=CARTESIAN_POINT('Ctrl Pts',(0.143465454207459,0.134879041457197,
1.41125839812423));
#26832=CARTESIAN_POINT('Ctrl Pts',(-0.0355118024153517,0.193684290169161,
1.42237218718103));
#26833=CARTESIAN_POINT('Ctrl Pts',(-0.181984703541769,0.0752081115995363,
1.43348597623784));
#26834=CARTESIAN_POINT('Ctrl Pts',(-0.16188494169705,-0.112106904510744,
1.44459976529464));
#26835=CARTESIAN_POINT('Ctrl Pts',(0.00638994323583646,-0.196809199398823,
1.45571355435144));
#26836=CARTESIAN_POINT('Ctrl Pts',(0.168816040557079,-0.101369802386164,
1.46682734340825));
#26837=CARTESIAN_POINT('Ctrl Pts',(0.17672290164568,0.0868545248928826,
1.47794113246505));
#26838=CARTESIAN_POINT('Ctrl Pts',(0.0228732863137639,0.195579919524334,
1.48905492152186));
#26839=CARTESIAN_POINT('Ctrl Pts',(-0.15191250667306,0.125288797732896,
1.50016871057866));
#26840=CARTESIAN_POINT('Ctrl Pts',(-0.187651060854054,-0.0596805852186566,
1.51128249963547));
#26841=CARTESIAN_POINT('Ctrl Pts',(-0.0516304683294577,-0.190023644566662,
1.52239628869227));
#26842=CARTESIAN_POINT('Ctrl Pts',(0.131648072412201,-0.146435920677088,
1.53351007774908));
#26843=CARTESIAN_POINT('Ctrl Pts',(0.194427649007747,0.0311862882363455,
1.54462386680588));
#26844=CARTESIAN_POINT('Ctrl Pts',(0.0792453752737409,0.180263283819487,
1.55573765586268));
#26845=CARTESIAN_POINT('Ctrl Pts',(-0.108471054243311,0.164343347185408,
1.56685144491949));
#26846=CARTESIAN_POINT('Ctrl Pts',(-0.196902764500876,-0.00200210229874768,
1.57796523397629));
#26847=CARTESIAN_POINT('Ctrl Pts',(-0.105107013422145,-0.16651465373019,
1.5890790230331));
#26848=CARTESIAN_POINT('Ctrl Pts',(0.0828941340502818,-0.178615126425815,
1.6001928120899));
#26849=CARTESIAN_POINT('Ctrl Pts',(0.195021809584276,-0.0272258612485208,
1.61130660114671));
#26850=CARTESIAN_POINT('Ctrl Pts',(0.128642913099457,0.149081079408297,
1.62242039020351));
#26851=CARTESIAN_POINT('Ctrl Pts',(-0.0554825813599488,0.188937135031884,
1.63353417926031));
#26852=CARTESIAN_POINT('Ctrl Pts',(-0.188827531603801,0.0558478560140352,
1.64464796831712));
#26853=CARTESIAN_POINT('Ctrl Pts',(-0.149330198326453,-0.128342305854753,
1.65576175737392));
#26854=CARTESIAN_POINT('Ctrl Pts',(0.0268386909069323,-0.195092411199392,
1.66687554643073));
#26855=CARTESIAN_POINT('Ctrl Pts',(0.178464943022445,-0.0832088009083063,
1.67798933548753));
#26856=CARTESIAN_POINT('Ctrl Pts',(0.166695798680381,0.104715122443915,
1.68910312454433));
#26857=CARTESIAN_POINT('Ctrl Pts',(0.00243441762381693,0.197027042329472,
1.70021691360114));
#26858=CARTESIAN_POINT('Ctrl Pts',(-0.164232046005026,0.108529764925501,
1.71133070265794));
#26859=CARTESIAN_POINT('Ctrl Pts',(-0.174839538171076,-0.0159901738299179,
1.71873989536248));
#26860=CARTESIAN_POINT('Ctrl Pts',(-0.152644235605294,-0.0667480137268189,
1.72244449171475));
#26861=CARTESIAN_POINT('Ctrl Pts',(-0.136778062465881,0.116331236980977,
0.792518502761751));
#26862=CARTESIAN_POINT('Ctrl Pts',(-0.175460966397852,0.0708492771249652,
0.796223099114019));
#26863=CARTESIAN_POINT('Ctrl Pts',(-0.203220400149799,-0.0609504310764289,
0.803632291818556));
#26864=CARTESIAN_POINT('Ctrl Pts',(-0.0587322509288797,-0.204085250153022,
0.814746080875359));
#26865=CARTESIAN_POINT('Ctrl Pts',(0.139477214667647,-0.159880475556692,
0.825859869932165));
#26866=CARTESIAN_POINT('Ctrl Pts',(0.210037654715023,0.0303954304627091,
0.836973658988967));
#26867=CARTESIAN_POINT('Ctrl Pts',(0.0883402297283485,0.192989395526265,
0.848087448045772));
#26868=CARTESIAN_POINT('Ctrl Pts',(-0.114211862278114,0.178865343704439,
0.859201237102576));
#26869=CARTESIAN_POINT('Ctrl Pts',(-0.212226703060007,0.00106173613023704,
0.87031502615938));
#26870=CARTESIAN_POINT('Ctrl Pts',(-0.115986907202372,-0.177733495821244,
0.881428815216186));
#26871=CARTESIAN_POINT('Ctrl Pts',(0.0864164308168349,-0.193836899073011,
0.892542604272987));
#26872=CARTESIAN_POINT('Ctrl Pts',(0.209722137515851,-0.0325245933019137,
0.903656393329794));
#26873=CARTESIAN_POINT('Ctrl Pts',(0.141066632550109,0.158560663604232,
0.914770182386597));
#26874=CARTESIAN_POINT('Ctrl Pts',(-0.0567086770128242,0.204512072930204,
0.925883971443401));
#26875=CARTESIAN_POINT('Ctrl Pts',(-0.20257793524978,0.0632720324586165,
0.936997760500206));
#26876=CARTESIAN_POINT('Ctrl Pts',(-0.163025289051846,-0.135882018994204,
0.948111549557009));
#26877=CARTESIAN_POINT('Ctrl Pts',(0.025746241081202,-0.210661507423248,
0.959225338613814));
#26878=CARTESIAN_POINT('Ctrl Pts',(0.190951951020682,-0.0926202387459321,
0.970339127670618));
#26879=CARTESIAN_POINT('Ctrl Pts',(0.181377171383915,0.110197442139303,
0.981452916727422));
#26880=CARTESIAN_POINT('Ctrl Pts',(0.00578581152757031,0.212150124582537,
0.992566705784226));
#26881=CARTESIAN_POINT('Ctrl Pts',(-0.175101368126144,0.119919407681051,
1.00368049484103));
#26882=CARTESIAN_POINT('Ctrl Pts',(-0.195716279284241,-0.0820749112141317,
1.01479428389783));
#26883=CARTESIAN_POINT('Ctrl Pts',(-0.0371898606828745,-0.208945128817718,
1.02590807295464));
#26884=CARTESIAN_POINT('Ctrl Pts',(0.15537685929014,-0.144565502642925,
1.03702186201144));
#26885=CARTESIAN_POINT('Ctrl Pts',(0.205725377795173,0.0521365687486478,
1.04813565106825));
#26886=CARTESIAN_POINT('Ctrl Pts',(0.0677711249544383,0.201117446888019,
1.05924944012505));
#26887=CARTESIAN_POINT('Ctrl Pts',(-0.132214807152008,0.166013245381199,
1.07036322918185));
#26888=CARTESIAN_POINT('Ctrl Pts',(-0.211183026844882,-0.0210447625070621,
1.08147701823866));
#26889=CARTESIAN_POINT('Ctrl Pts',(-0.0968530270931527,-0.188840260522183,
1.09259080729546));
#26890=CARTESIAN_POINT('Ctrl Pts',(0.106127646747548,-0.183788126532363,
1.10370459635227));
#26891=CARTESIAN_POINT('Ctrl Pts',(0.211968481949499,-0.0105126360047333,
1.11481838540907));
#26892=CARTESIAN_POINT('Ctrl Pts',(0.123792161737694,0.172385189467092,
1.12593217446588));
#26893=CARTESIAN_POINT('Ctrl Pts',(-0.0776925280115889,0.197496896045118,
1.13704596352268));
#26894=CARTESIAN_POINT('Ctrl Pts',(-0.208064365778478,0.0418374539025449,
1.14815975257949));
#26895=CARTESIAN_POINT('Ctrl Pts',(-0.147992529938032,-0.152116284264268,
1.15927354163629));
#26896=CARTESIAN_POINT('Ctrl Pts',(0.0475385469041886,-0.206836262328918,
1.17038733069309));
#26897=CARTESIAN_POINT('Ctrl Pts',(0.199557052641187,-0.0722366638006762,
1.1815011197499));
#26898=CARTESIAN_POINT('Ctrl Pts',(0.168918724964821,0.12848197232356,1.1926149088067));
#26899=CARTESIAN_POINT('Ctrl Pts',(-0.0163328273404871,0.211599602095504,
1.2037286978635));
#26900=CARTESIAN_POINT('Ctrl Pts',(-0.186634757554183,0.101037716366665,
1.21484248692031));
#26901=CARTESIAN_POINT('Ctrl Pts',(-0.18610777759643,-0.102005136998184,
1.22595627597711));
#26902=CARTESIAN_POINT('Ctrl Pts',(-0.0152342381989151,-0.211681531651681,
1.23707006503392));
#26903=CARTESIAN_POINT('Ctrl Pts',(0.169583372190078,-0.127603419752538,
1.24818385409072));
#26904=CARTESIAN_POINT('Ctrl Pts',(0.199179398807247,0.0732715493672994,
1.25929764314753));
#26905=CARTESIAN_POINT('Ctrl Pts',(0.046464262848129,0.207080238395369,
1.27041143220433));
#26906=CARTESIAN_POINT('Ctrl Pts',(-0.148780139836465,0.151346036770516,
1.28152522126114));
#26907=CARTESIAN_POINT('Ctrl Pts',(-0.207844393247192,-0.0429169086911673,
1.29263901031794));
#26908=CARTESIAN_POINT('Ctrl Pts',(-0.0766663164030391,-0.197897520917011,
1.30375279937474));
#26909=CARTESIAN_POINT('Ctrl Pts',(0.124685309300001,-0.171740287936918,
1.31486658843155));
#26910=CARTESIAN_POINT('Ctrl Pts',(0.211911057373125,0.0116127782590458,
1.32598037748835));
#26911=CARTESIAN_POINT('Ctrl Pts',(0.105172211397869,0.184336536816879,
1.33709416654516));
#26912=CARTESIAN_POINT('Ctrl Pts',(-0.0978319524040202,0.188334972707259,
1.34820795560196));
#26913=CARTESIAN_POINT('Ctrl Pts',(-0.211289420680394,0.0199482722156909,
1.35932174465877));
#26914=CARTESIAN_POINT('Ctrl Pts',(-0.131351286023602,-0.166697308065347,
1.37043553371557));
#26915=CARTESIAN_POINT('Ctrl Pts',(0.068814170356646,-0.200762951794954,
1.38154932277237));
#26916=CARTESIAN_POINT('Ctrl Pts',(0.205993236201476,-0.0510679889459757,
1.39266311182918));
#26917=CARTESIAN_POINT('Ctrl Pts',(0.154624356833139,0.14537008334725,1.40377690088598));
#26918=CARTESIAN_POINT('Ctrl Pts',(-0.0382739499121438,0.208749269721634,
1.41489068994279));
#26919=CARTESIAN_POINT('Ctrl Pts',(-0.196139676231217,0.0810578821846344,
1.42600447899959));
#26920=CARTESIAN_POINT('Ctrl Pts',(-0.174476532550337,-0.120826704256352,
1.43711826805639));
#26921=CARTESIAN_POINT('Ctrl Pts',(0.00688696012917997,-0.212117237867469,
1.4482320571132));
#26922=CARTESIAN_POINT('Ctrl Pts',(0.181946739990165,-0.109254458384087,
1.45934584617));
#26923=CARTESIAN_POINT('Ctrl Pts',(0.190468605530186,0.0936101664599312,
1.47045963522681));
#26924=CARTESIAN_POINT('Ctrl Pts',(0.0246523959685209,0.210792343236835,
1.48157342428361));
#26925=CARTESIAN_POINT('Ctrl Pts',(-0.163728430436396,0.135033899797455,
1.49268721334042));
#26926=CARTESIAN_POINT('Ctrl Pts',(-0.202246769118763,-0.0643226075283309,
1.50380100239722));
#26927=CARTESIAN_POINT('Ctrl Pts',(-0.0556463435921781,-0.204803895031906,
1.51491479145403));
#26928=CARTESIAN_POINT('Ctrl Pts',(0.141887805935659,-0.157825869489257,
1.52602858051082));
#26929=CARTESIAN_POINT('Ctrl Pts',(0.209550447837631,0.0336119924283981,
1.53714236956763));
#26930=CARTESIAN_POINT('Ctrl Pts',(0.0854091687186523,0.194284362567952,
1.54825615862443));
#26931=CARTESIAN_POINT('Ctrl Pts',(-0.116908053510435,0.177126155552421,
1.55936994768124));
#26932=CARTESIAN_POINT('Ctrl Pts',(-0.212218080567246,-0.00215782804277307,
1.57048373673804));
#26933=CARTESIAN_POINT('Ctrl Pts',(-0.113282353851889,-0.179466348735714,
1.58159752579485));
#26934=CARTESIAN_POINT('Ctrl Pts',(0.089341732011876,-0.192508009658716,
1.59271131485165));
#26935=CARTESIAN_POINT('Ctrl Pts',(0.210190822884773,-0.0293435190237031,
1.60382510390846));
#26936=CARTESIAN_POINT('Ctrl Pts',(0.138648901988495,0.160676771609172,
1.61493889296526));
#26937=CARTESIAN_POINT('Ctrl Pts',(-0.0597980782594448,0.203632875576831,
1.62605268202207));
#26938=CARTESIAN_POINT('Ctrl Pts',(-0.203514747072184,0.0601917643824736,
1.63716647107887));
#26939=CARTESIAN_POINT('Ctrl Pts',(-0.160945267273914,-0.13832491317789,
1.64828026013567));
#26940=CARTESIAN_POINT('Ctrl Pts',(0.0289262341422404,-0.210266915972054,
1.65939404919248));
#26941=CARTESIAN_POINT('Ctrl Pts',(0.19234614482316,-0.0896808740081667,
1.67050783824928));
#26942=CARTESIAN_POINT('Ctrl Pts',(0.179661583341645,0.112859981157414,
1.68162162730609));
#26943=CARTESIAN_POINT('Ctrl Pts',(0.00262376933475311,0.212352024863603,
1.69273541636289));
#26944=CARTESIAN_POINT('Ctrl Pts',(-0.177006197242412,0.116971330774799,
1.7038492054197));
#26945=CARTESIAN_POINT('Ctrl Pts',(-0.188438751949388,-0.0172339073385976,
1.71125839812423));
#26946=CARTESIAN_POINT('Ctrl Pts',(-0.164517074058987,-0.0719397484879835,
1.7149629944765));
#26947=CARTESIAN_POINT('Ctrl Pts',(-0.146649036946525,0.124726608657099,
0.785037005523502));
#26948=CARTESIAN_POINT('Ctrl Pts',(-0.188123601695047,0.0759623149459762,
0.78874160187577));
#26949=CARTESIAN_POINT('Ctrl Pts',(-0.217886373242709,-0.0653490907656594,
0.796150794580307));
#26950=CARTESIAN_POINT('Ctrl Pts',(-0.0629708293942997,-0.218813637584587,
0.807264583637111));
#26951=CARTESIAN_POINT('Ctrl Pts',(0.149542981076344,-0.171418700808033,
0.818378372693914));
#26952=CARTESIAN_POINT('Ctrl Pts',(0.225195614202741,0.0325890023924215,
0.829492161750719));
#26953=CARTESIAN_POINT('Ctrl Pts',(0.0947155514542305,0.206917019327413,
0.840605950807523));
#26954=CARTESIAN_POINT('Ctrl Pts',(-0.122454283303893,0.191773665487537,
0.851719739864327));
#26955=CARTESIAN_POINT('Ctrl Pts',(-0.227542641392875,0.00113835931130726,
0.862833528921131));
#26956=CARTESIAN_POINT('Ctrl Pts',(-0.124357429349293,-0.190560134610961,
0.873947317977936));
#26957=CARTESIAN_POINT('Ctrl Pts',(0.0926529161707207,-0.20782568535688,
0.885061107034739));
#26958=CARTESIAN_POINT('Ctrl Pts',(0.224857326815389,-0.0348718222704234,
0.896174896091545));
#26959=CARTESIAN_POINT('Ctrl Pts',(0.151247103781158,0.170003640905229,
0.907288685148347));
#26960=CARTESIAN_POINT('Ctrl Pts',(-0.0608012185617612,0.219271263230777,
0.918402474205154));
#26961=CARTESIAN_POINT('Ctrl Pts',(-0.217197543051952,0.0678382370566187,
0.929516263261956));
#26962=CARTESIAN_POINT('Ctrl Pts',(-0.174790468634879,-0.145688327971602,
0.940630052318761));
#26963=CARTESIAN_POINT('Ctrl Pts',(0.0276042911522686,-0.225864489000412,
0.951743841375564));
#26964=CARTESIAN_POINT('Ctrl Pts',(0.20473253689515,-0.0993044393887096,
0.962857630432368));
#26965=CARTESIAN_POINT('Ctrl Pts',(0.194466766292811,0.118150151218368,
0.973971419489174));
#26966=CARTESIAN_POINT('Ctrl Pts',(0.00620336092773602,0.227460536413689,
0.985085208545976));
#26967=CARTESIAN_POINT('Ctrl Pts',(-0.187738052000287,0.128573729811465,
0.996198997602783));
#26968=CARTESIAN_POINT('Ctrl Pts',(-0.209840696339377,-0.0879980785663373,
1.00731278665958));
#26969=CARTESIAN_POINT('Ctrl Pts',(-0.0398737718241875,-0.224024243094024,
1.01842657571639));
#26970=CARTESIAN_POINT('Ctrl Pts',(0.166590068377075,-0.154998479698188,
1.02954036477319));
#26971=CARTESIAN_POINT('Ctrl Pts',(0.22057212966186,0.055899151215077,1.04065415383));
#26972=CARTESIAN_POINT('Ctrl Pts',(0.0726620192461797,0.215631654430176,
1.0517679428868));
#26973=CARTESIAN_POINT('Ctrl Pts',(-0.141756461448261,0.177994059256345,
1.06288173194361));
#26974=CARTESIAN_POINT('Ctrl Pts',(-0.226423645341368,-0.0225635171224834,
1.07399552100041));
#26975=CARTESIAN_POINT('Ctrl Pts',(-0.103842698840025,-0.202468450298578,
1.08510931005722));
#26976=CARTESIAN_POINT('Ctrl Pts',(0.113786647568658,-0.197051714816478,
1.09622309911402));
#26977=CARTESIAN_POINT('Ctrl Pts',(0.227265785027954,-0.0112713100190907,
1.10733688817082));
#26978=CARTESIAN_POINT('Ctrl Pts',(0.132725972082619,0.184825852650891,
1.11845067722763));
#26979=CARTESIAN_POINT('Ctrl Pts',(-0.0832994283252297,0.211749816328691,
1.12956446628443));
#26980=CARTESIAN_POINT('Ctrl Pts',(-0.223079917307022,0.0448567717109849,
1.14067825534124));
#26981=CARTESIAN_POINT('Ctrl Pts',(-0.158672828079473,-0.163094184762292,
1.15179204439804));
#26982=CARTESIAN_POINT('Ctrl Pts',(0.0509693001615336,-0.221763184309772,
1.16290583345485));
#26983=CARTESIAN_POINT('Ctrl Pts',(0.213958649933481,-0.0774498262924409,
1.17401962251165));
#26984=CARTESIAN_POINT('Ctrl Pts',(0.181109220965206,0.137754236070862,
1.18513341156845));
#26985=CARTESIAN_POINT('Ctrl Pts',(-0.0175115318707909,0.226870283919355,
1.19624720062525));
#26986=CARTESIAN_POINT('Ctrl Pts',(-0.20010378099117,0.108329388012377,
1.20736098968206));
#26987=CARTESIAN_POINT('Ctrl Pts',(-0.199538770039111,-0.109366625281109,
1.21847477873886));
#26988=CARTESIAN_POINT('Ctrl Pts',(-0.0163336599466904,-0.226958126152927,
1.22958856779567));
#26989=CARTESIAN_POINT('Ctrl Pts',(0.181821834331238,-0.13681228027675,
1.24070235685247));
#26990=CARTESIAN_POINT('Ctrl Pts',(0.213553741645938,0.0785593972935142,
1.25181614590928));
#26991=CARTESIAN_POINT('Ctrl Pts',(0.0498174873679621,0.222024767596873,
1.26292993496608));
#26992=CARTESIAN_POINT('Ctrl Pts',(-0.159517278066646,0.162268350186683,
1.27404372402289));
#26993=CARTESIAN_POINT('Ctrl Pts',(-0.222844069837872,-0.0460141283976122,
1.28515751307969));
#26994=CARTESIAN_POINT('Ctrl Pts',(-0.0821991572628677,-0.212179353423901,
1.29627130213649));
#26995=CARTESIAN_POINT('Ctrl Pts',(0.13368357615671,-0.184134409983696,
1.3073850911933));
#26996=CARTESIAN_POINT('Ctrl Pts',(0.227204216245135,0.0124508471406916,
1.3184988802501));
#26997=CARTESIAN_POINT('Ctrl Pts',(0.112762260533419,0.197639702675246,
1.32961266930691));
#26998=CARTESIAN_POINT('Ctrl Pts',(-0.104892271055723,0.20192669696399,
1.34072645836371));
#26999=CARTESIAN_POINT('Ctrl Pts',(-0.226537717387964,0.0213878955180253,
1.35184024742052));
#27000=CARTESIAN_POINT('Ctrl Pts',(-0.140830621883197,-0.178727489252595,
1.36295403647732));
#27001=CARTESIAN_POINT('Ctrl Pts',(0.0737803389603765,-0.215251576199333,
1.37406782553412));
#27002=CARTESIAN_POINT('Ctrl Pts',(0.220859318825196,-0.0547534543384197,
1.38518161459093));
#27003=CARTESIAN_POINT('Ctrl Pts',(0.165783259458819,0.155861125237303,
1.39629540364773));
#27004=CARTESIAN_POINT('Ctrl Pts',(-0.0410360974089359,0.223814249274108,
1.40740919270454));
#27005=CARTESIAN_POINT('Ctrl Pts',(-0.210294648920666,0.0869076527697323,
1.41852298176134));
#27006=CARTESIAN_POINT('Ctrl Pts',(-0.187068123403623,-0.129546504001961,
1.42963677081815));
#27007=CARTESIAN_POINT('Ctrl Pts',(0.0073839770225235,-0.227425276336115,
1.44075055987495));
#27008=CARTESIAN_POINT('Ctrl Pts',(0.195077439423252,-0.117139114382011,
1.45186434893176));
#27009=CARTESIAN_POINT('Ctrl Pts',(0.204214309414691,0.10036580802698,1.46297813798855));
#27010=CARTESIAN_POINT('Ctrl Pts',(0.0264315056232782,0.226004766949337,
1.47409192704536));
#27011=CARTESIAN_POINT('Ctrl Pts',(-0.175544354199732,0.144779001862013,
1.48520571610217));
#27012=CARTESIAN_POINT('Ctrl Pts',(-0.216842477383471,-0.0689646298380053,
1.49631950515897));
#27013=CARTESIAN_POINT('Ctrl Pts',(-0.0596622188548986,-0.21958414549715,
1.50743329421577));
#27014=CARTESIAN_POINT('Ctrl Pts',(0.152127539459117,-0.169215818301425,
1.51854708327258));
#27015=CARTESIAN_POINT('Ctrl Pts',(0.224673246667516,0.0360376966204509,
1.52966087232938));
#27016=CARTESIAN_POINT('Ctrl Pts',(0.0915729621635637,0.208305441316416,
1.54077466138618));
#27017=CARTESIAN_POINT('Ctrl Pts',(-0.125345052777559,0.189908963919433,
1.55188845044299));
#27018=CARTESIAN_POINT('Ctrl Pts',(-0.227533396633615,-0.00231355378679829,
1.56300223949979));
#27019=CARTESIAN_POINT('Ctrl Pts',(-0.121457694281633,-0.192418043741239,
1.5741160285566));
#27020=CARTESIAN_POINT('Ctrl Pts',(0.09578932997347,-0.206400892891616,
1.5852298176134));
#27021=CARTESIAN_POINT('Ctrl Pts',(0.225359836185271,-0.0314611767988859,
1.59634360667021));
#27022=CARTESIAN_POINT('Ctrl Pts',(0.148654890877534,0.172272463810048,
1.60745739572701));
#27023=CARTESIAN_POINT('Ctrl Pts',(-0.0641135751589405,0.218328616121778,
1.61857118478381));
#27024=CARTESIAN_POINT('Ctrl Pts',(-0.218201962540567,0.0645356727509123,
1.62968497384062));
#27025=CARTESIAN_POINT('Ctrl Pts',(-0.172560336221374,-0.148307520501026,
1.64079876289742));
#27026=CARTESIAN_POINT('Ctrl Pts',(0.0310137773775485,-0.225441420744716,
1.65191255195423));
#27027=CARTESIAN_POINT('Ctrl Pts',(0.206227346623875,-0.0961529471080275,
1.66302634101103));
#27028=CARTESIAN_POINT('Ctrl Pts',(0.192627368002909,0.121004839870914,
1.67414013006784));
#27029=CARTESIAN_POINT('Ctrl Pts',(0.00281312104568935,0.227677007397733,
1.68525391912464));
#27030=CARTESIAN_POINT('Ctrl Pts',(-0.189780348479797,0.125412896624096,
1.69636770818145));
#27031=CARTESIAN_POINT('Ctrl Pts',(-0.202037965727701,-0.0184776408472769,
1.70377690088598));
#27032=CARTESIAN_POINT('Ctrl Pts',(-0.17638991251268,-0.0771314832491481,
1.70748149723825));
#27033=CARTESIAN_POINT('Ctrl Pts',(-0.156520011427169,0.133121980333222,
0.777555508285253));
#27034=CARTESIAN_POINT('Ctrl Pts',(-0.200786236992242,0.081075352766987,
0.781260104637521));
#27035=CARTESIAN_POINT('Ctrl Pts',(-0.232552346335619,-0.0697477504548899,
0.788669297342057));
#27036=CARTESIAN_POINT('Ctrl Pts',(-0.06720940785972,-0.233542025016153,
0.799783086398862));
#27037=CARTESIAN_POINT('Ctrl Pts',(0.159608747485041,-0.182956926059375,
0.810896875455666));
#27038=CARTESIAN_POINT('Ctrl Pts',(0.240353573690459,0.0347825743221341,
0.82201066451247));
#27039=CARTESIAN_POINT('Ctrl Pts',(0.101090873180113,0.220844643128561,
0.833124453569275));
#27040=CARTESIAN_POINT('Ctrl Pts',(-0.130696704329673,0.204681987270635,
0.844238242626078));
#27041=CARTESIAN_POINT('Ctrl Pts',(-0.242858579725743,0.00121498249237738,
0.855352031682883));
#27042=CARTESIAN_POINT('Ctrl Pts',(-0.132727951496213,-0.203386773400678,
0.866465820739686));
#27043=CARTESIAN_POINT('Ctrl Pts',(0.0988894015246068,-0.221814471640749,
0.877579609796491));
#27044=CARTESIAN_POINT('Ctrl Pts',(0.239992516114928,-0.0372190512389329,
0.888693398853296));
#27045=CARTESIAN_POINT('Ctrl Pts',(0.161427575012208,0.181446618206226,
0.899807187910099));
#27046=CARTESIAN_POINT('Ctrl Pts',(-0.0648937601106981,0.234030453531351,
0.910920976966904));
#27047=CARTESIAN_POINT('Ctrl Pts',(-0.231817150854124,0.0724044416546206,
0.922034766023707));
#27048=CARTESIAN_POINT('Ctrl Pts',(-0.186555648217912,-0.155494636948999,
0.933148555080512));
#27049=CARTESIAN_POINT('Ctrl Pts',(0.029462341223335,-0.241067470577576,
0.944262344137316));
#27050=CARTESIAN_POINT('Ctrl Pts',(0.218513122769618,-0.105988640031487,
0.95537613319412));
#27051=CARTESIAN_POINT('Ctrl Pts',(0.207556361201707,0.126102860297433,
0.966489922250924));
#27052=CARTESIAN_POINT('Ctrl Pts',(0.00662091032790181,0.242770948244842,
0.977603711307729));
#27053=CARTESIAN_POINT('Ctrl Pts',(-0.200374735874429,0.13722805194188,
0.988717500364533));
#27054=CARTESIAN_POINT('Ctrl Pts',(-0.223965113394512,-0.0939212459185429,
0.999831289421336));
#27055=CARTESIAN_POINT('Ctrl Pts',(-0.0425576829655005,-0.239103357370329,
1.01094507847814));
#27056=CARTESIAN_POINT('Ctrl Pts',(0.177803277464009,-0.16543145675345,
1.02205886753495));
#27057=CARTESIAN_POINT('Ctrl Pts',(0.235418881528546,0.0596617336815061,
1.03317265659175));
#27058=CARTESIAN_POINT('Ctrl Pts',(0.0775529135379212,0.230145861972334,
1.04428644564855));
#27059=CARTESIAN_POINT('Ctrl Pts',(-0.151298115744515,0.18997487313149,
1.05540023470536));
#27060=CARTESIAN_POINT('Ctrl Pts',(-0.241664263837854,-0.0240822717379046,
1.06651402376216));
#27061=CARTESIAN_POINT('Ctrl Pts',(-0.110832370586897,-0.216096640074974,
1.07762781281897));
#27062=CARTESIAN_POINT('Ctrl Pts',(0.121445648389767,-0.210315303100593,
1.08874160187577));
#27063=CARTESIAN_POINT('Ctrl Pts',(0.242563088106409,-0.0120299840334481,
1.09985539093258));
#27064=CARTESIAN_POINT('Ctrl Pts',(0.141659782427545,0.197266515834691,
1.11096917998938));
#27065=CARTESIAN_POINT('Ctrl Pts',(-0.0889063286388705,0.226002736612265,
1.12208296904618));
#27066=CARTESIAN_POINT('Ctrl Pts',(-0.238095468835566,0.0478760895194249,
1.13319675810299));
#27067=CARTESIAN_POINT('Ctrl Pts',(-0.169353126220915,-0.174072085260317,
1.14431054715979));
#27068=CARTESIAN_POINT('Ctrl Pts',(0.0544000534188783,-0.236690106290626,
1.1554243362166));
#27069=CARTESIAN_POINT('Ctrl Pts',(0.228360247225775,-0.0826629887842052,
1.1665381252734));
#27070=CARTESIAN_POINT('Ctrl Pts',(0.193299716965591,0.147026499818165,
1.1776519143302));
#27071=CARTESIAN_POINT('Ctrl Pts',(-0.0186902364010947,0.242140965743205,
1.18876570338701));
#27072=CARTESIAN_POINT('Ctrl Pts',(-0.213572804428157,0.115621059658089,
1.19987949244381));
#27073=CARTESIAN_POINT('Ctrl Pts',(-0.212969762481792,-0.116728113564033,
1.21099328150062));
#27074=CARTESIAN_POINT('Ctrl Pts',(-0.0174330816944656,-0.242234720654174,
1.22210707055742));
#27075=CARTESIAN_POINT('Ctrl Pts',(0.194060296472398,-0.146021140800962,
1.23322085961423));
#27076=CARTESIAN_POINT('Ctrl Pts',(0.227928084484629,0.0838472452197288,
1.24433464867103));
#27077=CARTESIAN_POINT('Ctrl Pts',(0.053170711887795,0.236969296798376,
1.25544843772783));
#27078=CARTESIAN_POINT('Ctrl Pts',(-0.170254416296827,0.17319066360285,
1.26656222678464));
#27079=CARTESIAN_POINT('Ctrl Pts',(-0.237843746428552,-0.0491113481040567,
1.27767601584144));
#27080=CARTESIAN_POINT('Ctrl Pts',(-0.0877319981226961,-0.226461185930791,
1.28878980489824));
#27081=CARTESIAN_POINT('Ctrl Pts',(0.142681843013418,-0.196528532030473,
1.29990359395505));
#27082=CARTESIAN_POINT('Ctrl Pts',(0.242497375117146,0.0132889160223372,
1.31101738301185));
#27083=CARTESIAN_POINT('Ctrl Pts',(0.120352309668968,0.210942868533614,
1.32213117206866));
#27084=CARTESIAN_POINT('Ctrl Pts',(-0.111952589707427,0.215518421220722,
1.33324496112546));
#27085=CARTESIAN_POINT('Ctrl Pts',(-0.241786014095534,0.0228275188203595,
1.34435875018226));
#27086=CARTESIAN_POINT('Ctrl Pts',(-0.150309957742793,-0.190757670439842,
1.35547253923907));
#27087=CARTESIAN_POINT('Ctrl Pts',(0.0787465075641072,-0.229740200603712,
1.36658632829588));
#27088=CARTESIAN_POINT('Ctrl Pts',(0.235725401448916,-0.0584389197308638,
1.37770011735268));
#27089=CARTESIAN_POINT('Ctrl Pts',(0.176942162084499,0.166352167127356,
1.38881390640948));
#27090=CARTESIAN_POINT('Ctrl Pts',(-0.0437982449057285,0.238879228826581,
1.39992769546629));
#27091=CARTESIAN_POINT('Ctrl Pts',(-0.224449621610114,0.0927574233548304,
1.41104148452309));
#27092=CARTESIAN_POINT('Ctrl Pts',(-0.199659714256911,-0.13826630374757,
1.42215527357989));
#27093=CARTESIAN_POINT('Ctrl Pts',(0.00788099391586731,-0.242733314804761,
1.4332690626367));
#27094=CARTESIAN_POINT('Ctrl Pts',(0.208208138856338,-0.125023770379934,
1.4443828516935));
#27095=CARTESIAN_POINT('Ctrl Pts',(0.217960013299196,0.107121449594028,
1.45549664075031));
#27096=CARTESIAN_POINT('Ctrl Pts',(0.028210615278035,0.241217190661839,
1.46661042980711));
#27097=CARTESIAN_POINT('Ctrl Pts',(-0.187360277963068,0.154524103926572,
1.47772421886392));
#27098=CARTESIAN_POINT('Ctrl Pts',(-0.23143818564818,-0.0736066521476796,
1.48883800792072));
#27099=CARTESIAN_POINT('Ctrl Pts',(-0.0636780941176189,-0.234364395962394,
1.49995179697753));
#27100=CARTESIAN_POINT('Ctrl Pts',(0.162367272982574,-0.180605767113594,
1.51106558603433));
#27101=CARTESIAN_POINT('Ctrl Pts',(0.2397960454974,0.0384634008125035,1.52217937509113));
#27102=CARTESIAN_POINT('Ctrl Pts',(0.0977367556084749,0.222326520064881,
1.53329316414794));
#27103=CARTESIAN_POINT('Ctrl Pts',(-0.133782052044684,0.202691772286445,
1.54440695320474));
#27104=CARTESIAN_POINT('Ctrl Pts',(-0.242848712699985,-0.00246927953082339,
1.55552074226155));
#27105=CARTESIAN_POINT('Ctrl Pts',(-0.129633034711377,-0.205369738746763,
1.56663453131835));
#27106=CARTESIAN_POINT('Ctrl Pts',(0.102236927935064,-0.220293776124516,
1.57774832037515));
#27107=CARTESIAN_POINT('Ctrl Pts',(0.240528849485768,-0.0335788345740686,
1.58886210943196));
#27108=CARTESIAN_POINT('Ctrl Pts',(0.158660879766572,0.183868156010923,
1.59997589848876));
#27109=CARTESIAN_POINT('Ctrl Pts',(-0.0684290720584363,0.233024356666725,
1.61108968754557));
#27110=CARTESIAN_POINT('Ctrl Pts',(-0.23288917800895,0.0688795811193509,
1.62220347660237));
#27111=CARTESIAN_POINT('Ctrl Pts',(-0.184175405168835,-0.158290127824162,
1.63331726565918));
#27112=CARTESIAN_POINT('Ctrl Pts',(0.0331013206128567,-0.240615925517378,
1.64443105471598));
#27113=CARTESIAN_POINT('Ctrl Pts',(0.220108548424591,-0.102625020207888,
1.65554484377279));
#27114=CARTESIAN_POINT('Ctrl Pts',(0.205593152664173,0.129149698584414,
1.66665863282959));
#27115=CARTESIAN_POINT('Ctrl Pts',(0.00300247275662535,0.243001989931863,
1.67777242188639));
#27116=CARTESIAN_POINT('Ctrl Pts',(-0.202554499717183,0.133854462473394,
1.6888862109432));
#27117=CARTESIAN_POINT('Ctrl Pts',(-0.215637179506013,-0.0197213743559566,
1.69629540364773));
#27118=CARTESIAN_POINT('Ctrl Pts',(-0.188262750966373,-0.0823232180103128,
1.7));
#27119=CARTESIAN_POINT('Ctrl Pts',(-0.126907087985236,0.107935865304854,
0.8));
#27120=CARTESIAN_POINT('Ctrl Pts',(-0.135120815820747,0.100273328983374,
0.8));
#27121=CARTESIAN_POINT('Ctrl Pts',(-0.142440162795362,0.0917707005673423,
0.8));
#27122=CARTESIAN_POINT('Ctrl Pts',(-0.148860420961125,0.0826220371750322,
0.8));
#27123=CARTESIAN_POINT('Ctrl Pts',(-0.153630780718642,0.0758244264629785,
0.8));
#27124=CARTESIAN_POINT('Ctrl Pts',(-0.157904437427575,0.0686688635836137,
0.8));
#27125=CARTESIAN_POINT('Ctrl Pts',(-0.161669292800466,0.0612205436816197,
0.8));
#27126=CARTESIAN_POINT('Ctrl Pts',(-0.163886790527543,0.0568334873893247,
0.8));
#27127=CARTESIAN_POINT('Ctrl Pts',(-0.165929164676721,0.0523396591094527,
0.8));
#27128=CARTESIAN_POINT('Ctrl Pts',(-0.167781485419322,0.0477808011974605,
0.8));
#27129=CARTESIAN_POINT('Ctrl Pts',(-0.172341905336402,0.0365568776388491,
0.8));
#27130=CARTESIAN_POINT('Ctrl Pts',(-0.175769282371032,0.024914892102173,
0.8));
#27131=CARTESIAN_POINT('Ctrl Pts',(-0.178035222124413,0.0130530737274266,
0.8));
#27132=CARTESIAN_POINT('Ctrl Pts',(-0.179475251863618,0.00551475714368376,
0.8));
#27133=CARTESIAN_POINT('Ctrl Pts',(-0.180445476974817,-0.00211322491662525,
0.8));
#27134=CARTESIAN_POINT('Ctrl Pts',(-0.180929041702956,-0.00978511330991493,
0.8));
#27135=CARTESIAN_POINT('Ctrl Pts',(-0.181154762272538,-0.0133662326867636,
0.8));
#27136=CARTESIAN_POINT('Ctrl Pts',(-0.181273901675413,-0.0169534510679824,
0.8));
#27137=CARTESIAN_POINT('Ctrl Pts',(-0.181285306139082,-0.0205319858475477,
0.8));
#27138=CARTESIAN_POINT('Ctrl Pts',(-0.18132084415518,-0.0316832359459324,
0.8));
#27139=CARTESIAN_POINT('Ctrl Pts',(-0.180314596981932,-0.0427772557222799,
0.8));
#27140=CARTESIAN_POINT('Ctrl Pts',(-0.178232649680767,-0.053673233795859,
0.8));
#27141=CARTESIAN_POINT('Ctrl Pts',(-0.177072367625385,-0.0597456294936455,
0.8));
#27142=CARTESIAN_POINT('Ctrl Pts',(-0.175577442236952,-0.0657567536750286,
0.8));
#27143=CARTESIAN_POINT('Ctrl Pts',(-0.173766632602371,-0.0716904360104152,
0.8));
#27144=CARTESIAN_POINT('Ctrl Pts',(-0.17263375533703,-0.0754026615746807,
0.8));
#27145=CARTESIAN_POINT('Ctrl Pts',(-0.171376588698951,-0.0790860937830887,
0.8));
#27146=CARTESIAN_POINT('Ctrl Pts',(-0.17000084111904,-0.0827319119339195,
0.8));
#27147=CARTESIAN_POINT('Ctrl Pts',(-0.165618690539351,-0.0943448882941177,
0.8));
#27148=CARTESIAN_POINT('Ctrl Pts',(-0.160069009775015,-0.105495622492882,
0.8));
#27149=CARTESIAN_POINT('Ctrl Pts',(-0.153517412526831,-0.116061366452211,
0.8));
#27150=CARTESIAN_POINT('Ctrl Pts',(-0.149177021710609,-0.123061103510275,
0.8));
#27151=CARTESIAN_POINT('Ctrl Pts',(-0.144395700078728,-0.129804236115551,
0.8));
#27152=CARTESIAN_POINT('Ctrl Pts',(-0.139210064136084,-0.136252864813496,
0.8));
#27153=CARTESIAN_POINT('Ctrl Pts',(-0.13649895134849,-0.139624285391187,
0.8));
#27154=CARTESIAN_POINT('Ctrl Pts',(-0.133675938748059,-0.142916515743411,
0.8));
#27155=CARTESIAN_POINT('Ctrl Pts',(-0.130749381376745,-0.146119375612755,
0.8));
#27156=CARTESIAN_POINT('Ctrl Pts',(-0.124483125872831,-0.152977241609597,
0.8));
#27157=CARTESIAN_POINT('Ctrl Pts',(-0.117767487241387,-0.159399582279811,
0.8));
#27158=CARTESIAN_POINT('Ctrl Pts',(-0.110656616745505,-0.165335584860524,
0.8));
#27159=CARTESIAN_POINT('Ctrl Pts',(-0.106173937599239,-0.169077629522446,
0.8));
#27160=CARTESIAN_POINT('Ctrl Pts',(-0.10153394483554,-0.172626328540978,
0.8));
#27161=CARTESIAN_POINT('Ctrl Pts',(-0.0967480797506452,-0.175967583788754,
0.8));
#27162=CARTESIAN_POINT('Ctrl Pts',(-0.0926327467056763,-0.178840706597052,
0.8));
#27163=CARTESIAN_POINT('Ctrl Pts',(-0.0884162860091264,-0.181555556620875,
0.8));
#27164=CARTESIAN_POINT('Ctrl Pts',(-0.0841104480426287,-0.184101786598396,
0.8));
#27165=CARTESIAN_POINT('Ctrl Pts',(-0.0753786167196158,-0.189265299681399,
0.8));
#27166=CARTESIAN_POINT('Ctrl Pts',(-0.0662752406232737,-0.193739549767325,
0.8));
#27167=CARTESIAN_POINT('Ctrl Pts',(-0.0568593821206139,-0.197450435399565,
0.8));
#27168=CARTESIAN_POINT('Ctrl Pts',(-0.0556199805901397,-0.197938896152316,
0.8));
#27169=CARTESIAN_POINT('Ctrl Pts',(-0.0543751496950137,-0.198414110578975,
0.8));
#27170=CARTESIAN_POINT('Ctrl Pts',(-0.0531250805644623,-0.198876136975596,
0.8));
#27171=CARTESIAN_POINT('Ctrl Pts',(0.166729862742343,-0.000130123946020723,
0.912851963660979));
#27172=CARTESIAN_POINT('Ctrl Pts',(0.166803013417109,-0.0086545516860567,
0.912280605963333));
#27173=CARTESIAN_POINT('Ctrl Pts',(0.166205714872852,-0.0171686904331816,
0.911709248265688));
#27174=CARTESIAN_POINT('Ctrl Pts',(0.164902316607877,-0.0255733139699205,
0.911137890568042));
#27175=CARTESIAN_POINT('Ctrl Pts',(0.156451280631859,-0.08006761381865,
0.907433294215774));
#27176=CARTESIAN_POINT('Ctrl Pts',(0.118315613047404,-0.129957863303896,
0.903728697863506));
#27177=CARTESIAN_POINT('Ctrl Pts',(0.0679483908354429,-0.152412778753583,
0.900024101511237));
#27178=CARTESIAN_POINT('Ctrl Pts',(0.017581168623482,-0.17486769420327,
0.896319505158969));
#27179=CARTESIAN_POINT('Ctrl Pts',(-0.045017608215985,-0.169887275617398,
0.892614908806701));
#27180=CARTESIAN_POINT('Ctrl Pts',(-0.0911993932476663,-0.139748404661014,
0.888910312454434));
#27181=CARTESIAN_POINT('Ctrl Pts',(-0.137381178279348,-0.109609533704629,
0.885205716102165));
#27182=CARTESIAN_POINT('Ctrl Pts',(-0.167145971503243,-0.0543122103777309,
0.881501119749897));
#27183=CARTESIAN_POINT('Ctrl Pts',(-0.16687148086939,0.000831769447747308,
0.877796523397629));
#27184=CARTESIAN_POINT('Ctrl Pts',(-0.166596990235537,0.0559757492732252,
0.874091927045361));
#27185=CARTESIAN_POINT('Ctrl Pts',(-0.136283215743936,0.110966385597283,
0.870387330693093));
#27186=CARTESIAN_POINT('Ctrl Pts',(-0.0898039369556689,0.140645828726608,
0.866682734340825));
#27187=CARTESIAN_POINT('Ctrl Pts',(-0.0433246581674013,0.170325271855933,
0.862978137988557));
#27188=CARTESIAN_POINT('Ctrl Pts',(0.0193201249175325,0.174693521790525,
0.859273541636289));
#27189=CARTESIAN_POINT('Ctrl Pts',(0.0694616476641393,0.151734327892468,
0.855568945284021));
#27190=CARTESIAN_POINT('Ctrl Pts',(0.119603170410746,0.12877513399441,0.851864348931753));
#27191=CARTESIAN_POINT('Ctrl Pts',(0.157241432819026,0.0784884962637034,
0.848159752579484));
#27192=CARTESIAN_POINT('Ctrl Pts',(0.16514918952844,0.0239211592586256,
0.844455156227216));
#27193=CARTESIAN_POINT('Ctrl Pts',(0.166289903708577,0.0160496809897125,
0.843920758705137));
#27194=CARTESIAN_POINT('Ctrl Pts',(0.16681196167645,0.00808912649634021,
0.843386361183058));
#27195=CARTESIAN_POINT('Ctrl Pts',(0.166745353727506,0.000120148921586877,
0.842851963660979));
#27196=CARTESIAN_POINT('Ctrl Pts',(0.0530170217188587,-0.198517432567173,
0.8));
#27197=CARTESIAN_POINT('Ctrl Pts',(0.119028790974553,-0.18088801151799,
0.803704596352268));
#27198=CARTESIAN_POINT('Ctrl Pts',(0.230942256426658,-0.0749063428374961,
0.811113789056804));
#27199=CARTESIAN_POINT('Ctrl Pts',(0.188114631577322,0.153856547759368,
0.822227578113608));
#27200=CARTESIAN_POINT('Ctrl Pts',(-0.0272119409517698,0.241262826763902,
0.833341367170412));
#27201=CARTESIAN_POINT('Ctrl Pts',(-0.217470922739143,0.108102090643486,
0.844455156227217));
#27202=CARTESIAN_POINT('Ctrl Pts',(-0.208759451561279,-0.124141896006793,
0.85556894528402));
#27203=CARTESIAN_POINT('Ctrl Pts',(-0.00892472216375234,-0.242686445659381,
0.866682734340826));
#27204=CARTESIAN_POINT('Ctrl Pts',(0.199056267666047,-0.139134372529335,
0.877796523397629));
#27205=CARTESIAN_POINT('Ctrl Pts',(0.224850619698646,0.091788306500609,
0.888910312454433));
#27206=CARTESIAN_POINT('Ctrl Pts',(0.0448304764247631,0.238686010114805,
0.900024101511237));
#27207=CARTESIAN_POINT('Ctrl Pts',(-0.176220286722883,0.167116974718297,
0.911137890568042));
#27208=CARTESIAN_POINT('Ctrl Pts',(-0.235976306336092,-0.0574188764093974,
0.922251679624847));
#27209=CARTESIAN_POINT('Ctrl Pts',(-0.0797396575425977,-0.229397140881452,
0.933365468681649));
#27210=CARTESIAN_POINT('Ctrl Pts',(0.14948314505928,-0.19140635164143,0.944479257738454));
#27211=CARTESIAN_POINT('Ctrl Pts',(0.241882569451173,0.0217812340617926,
0.955593046795258));
#27212=CARTESIAN_POINT('Ctrl Pts',(0.112884009708659,0.215032004451281,
0.966706835852063));
#27213=CARTESIAN_POINT('Ctrl Pts',(-0.119438498942156,0.211461649464463,
0.977820624908867));
#27214=CARTESIAN_POINT('Ctrl Pts',(-0.242437629122786,0.0143379927471741,
0.988934413965671));
#27215=CARTESIAN_POINT('Ctrl Pts',(-0.143530830111561,-0.195909362177039,
1.00004820302247));
#27216=CARTESIAN_POINT('Ctrl Pts',(0.086751356142284,-0.226838671363958,
1.01116199207928));
#27217=CARTESIAN_POINT('Ctrl Pts',(0.237629047152892,-0.05013996417456,
1.02227578113608));
#27218=CARTESIAN_POINT('Ctrl Pts',(0.1710021738693,0.172452416697446,1.03338957019289));
#27219=CARTESIAN_POINT('Ctrl Pts',(-0.0521449271278155,0.237197146991165,
1.04450335924969));
#27220=CARTESIAN_POINT('Ctrl Pts',(-0.227563185653378,0.0848326375129703,
1.0556171483065));
#27221=CARTESIAN_POINT('Ctrl Pts',(-0.194690279246867,-0.145180146557101,
1.0667309373633));
#27222=CARTESIAN_POINT('Ctrl Pts',(0.0163848475034698,-0.242307896337387,
1.0778447264201));
#27223=CARTESIAN_POINT('Ctrl Pts',(0.212462737615647,-0.117648480480376,
1.08895851547691));
#27224=CARTESIAN_POINT('Ctrl Pts',(0.214071074445423,0.114695923700636,
1.10007230453371));
#27225=CARTESIAN_POINT('Ctrl Pts',(0.019737729131079,0.242057848222183,
1.11118609359052));
#27226=CARTESIAN_POINT('Ctrl Pts',(-0.192661783512051,0.147861479120299,
1.12229988264732));
#27227=CARTESIAN_POINT('Ctrl Pts',(-0.228715780766039,-0.0816741786716276,
1.13341367170413));
#27228=CARTESIAN_POINT('Ctrl Pts',(-0.0554236300753314,-0.236452534483491,
1.14452746076093));
#27229=CARTESIAN_POINT('Ctrl Pts',(0.168598397772042,-0.174803203925221,
1.15564124981773));
#27230=CARTESIAN_POINT('Ctrl Pts',(0.238300400101745,0.0468454815872605,
1.16675503887454));
#27231=CARTESIAN_POINT('Ctrl Pts',(0.0898833437085198,0.225615966539919,
1.17786882793134));
#27232=CARTESIAN_POINT('Ctrl Pts',(-0.140804956527845,0.197877598659039,
1.18898261698814));
#27233=CARTESIAN_POINT('Ctrl Pts',(-0.242612883217311,-0.0109803793588139,
1.20009640604495));
#27234=CARTESIAN_POINT('Ctrl Pts',(-0.12235448648082,-0.2097878916237,1.21121019510175));
#27235=CARTESIAN_POINT('Ctrl Pts',(0.109896359325859,-0.21657416752884,
1.22232398415856));
#27236=CARTESIAN_POINT('Ctrl Pts',(0.241557821132076,-0.0251276517767584,
1.23343777321536));
#27237=CARTESIAN_POINT('Ctrl Pts',(0.152118669804104,0.189318488613562,
1.24455156227217));
#27238=CARTESIAN_POINT('Ctrl Pts',(-0.0765564251386213,0.230479269358191,
1.25566535132897));
#27239=CARTESIAN_POINT('Ctrl Pts',(-0.23515855594305,0.0606797610465845,
1.26677914038578));
#27240=CARTESIAN_POINT('Ctrl Pts',(-0.178517393613401,-0.164660620706261,
1.27789292944258));
#27241=CARTESIAN_POINT('Ctrl Pts',(0.0415227636155418,-0.239285268948212,
1.28900671849938));
#27242=CARTESIAN_POINT('Ctrl Pts',(0.223556664406995,-0.0948893968423596,
1.30012050755619));
#27243=CARTESIAN_POINT('Ctrl Pts',(0.200966614961749,0.136359816312279,
1.31123429661299));
#27244=CARTESIAN_POINT('Ctrl Pts',(-0.00557045627447471,0.242797343170749,
1.3223480856698));
#27245=CARTESIAN_POINT('Ctrl Pts',(-0.207008825709279,0.126999708315969,
1.3334618747266));
#27246=CARTESIAN_POINT('Ctrl Pts',(-0.218969669332857,-0.105042199835232,
1.3445756637834));
#27247=CARTESIAN_POINT('Ctrl Pts',(-0.0305050913306782,-0.240937791217362,
1.35568945284021));
#27248=CARTESIAN_POINT('Ctrl Pts',(0.185881142716884,-0.15630028987845,
1.36680324189701));
#27249=CARTESIAN_POINT('Ctrl Pts',(0.23212825880178,0.0714006393532108,
1.37791703095382));
#27250=CARTESIAN_POINT('Ctrl Pts',(0.0659057470887793,0.233747753644337,
1.38903082001062));
#27251=CARTESIAN_POINT('Ctrl Pts',(-0.160641042350602,0.182142898149225,
1.40014460906743));
#27252=CARTESIAN_POINT('Ctrl Pts',(-0.240151263944613,-0.0361794176709605,
1.41125839812423));
#27253=CARTESIAN_POINT('Ctrl Pts',(-0.0998483101275995,-0.221386302178844,
1.42237218718103));
#27254=CARTESIAN_POINT('Ctrl Pts',(0.131846934264022,-0.203955793640817,
1.43348597623784));
#27255=CARTESIAN_POINT('Ctrl Pts',(0.242861184558351,0.00015776588975909,
1.44459976529464));
#27256=CARTESIAN_POINT('Ctrl Pts',(0.13158183823911,0.204126920402922,1.45571355435144));
#27257=CARTESIAN_POINT('Ctrl Pts',(-0.10013585656473,0.221256389923926,
1.46682734340825));
#27258=CARTESIAN_POINT('Ctrl Pts',(-0.240198066802314,0.0358673761285168,
1.47794113246505));
#27259=CARTESIAN_POINT('Ctrl Pts',(-0.160404261381875,-0.182351453033287,
1.48905492152186));
#27260=CARTESIAN_POINT('Ctrl Pts',(0.0662093815164626,-0.233661930697804,
1.50016871057866));
#27261=CARTESIAN_POINT('Ctrl Pts',(0.232220830617013,-0.0710989904726924,
1.51128249963547));
#27262=CARTESIAN_POINT('Ctrl Pts',(0.185677912288661,0.156541656658069,
1.52239628869227));
#27263=CARTESIAN_POINT('Ctrl Pts',(-0.0308180903310451,0.240897960470908,
1.53351007774908));
#27264=CARTESIAN_POINT('Ctrl Pts',(-0.219105973246366,0.104757609325286,
1.54462386680588));
#27265=CARTESIAN_POINT('Ctrl Pts',(-0.206843620635952,-0.127268531807556,
1.55573765586268));
#27266=CARTESIAN_POINT('Ctrl Pts',(-0.00525505851706014,-0.242804414954791,
1.56685144491949));
#27267=CARTESIAN_POINT('Ctrl Pts',(0.201143714017778,-0.136098524667356,
1.57796523397629));
#27268=CARTESIAN_POINT('Ctrl Pts',(0.223432989115882,0.0951796228419585,
1.5890790230331));
#27269=CARTESIAN_POINT('Ctrl Pts',(0.041212233239435,0.2393392912824,1.6001928120899));
#27270=CARTESIAN_POINT('Ctrl Pts',(-0.178731921787321,0.164428017156146,
1.6113066011467));
#27271=CARTESIAN_POINT('Ctrl Pts',(-0.235078089364662,-0.0609842187918821,
1.62242039020351));
#27272=CARTESIAN_POINT('Ctrl Pts',(-0.0762596568913861,-0.230580482955351,
1.63353417926032));
#27273=CARTESIAN_POINT('Ctrl Pts',(0.15236975797671,-0.18911696954633,1.64464796831712));
#27274=CARTESIAN_POINT('Ctrl Pts',(0.241514918660579,0.0254343397173533,
1.65576175737392));
#27275=CARTESIAN_POINT('Ctrl Pts',(0.109634140470589,0.216730418270261,
1.66687554643072));
#27276=CARTESIAN_POINT('Ctrl Pts',(-0.122663843019391,0.209602590285094,
1.67798933548753));
#27277=CARTESIAN_POINT('Ctrl Pts',(-0.242556018767321,0.0107153659861808,
1.68910312454434));
#27278=CARTESIAN_POINT('Ctrl Pts',(-0.140685982558438,-0.198157528783211,
1.70021691360114));
#27279=CARTESIAN_POINT('Ctrl Pts',(0.0904627772969653,-0.225303732602113,
1.71133070265794));
#27280=CARTESIAN_POINT('Ctrl Pts',(0.188575434363683,-0.106431345694512,
1.71873989536248));
#27281=CARTESIAN_POINT('Ctrl Pts',(0.201667586144654,-0.0393720754290199,
1.72244449171475));
#27282=CARTESIAN_POINT('Ctrl Pts',(0.0496734897087673,-0.185997880000277,
0.792518502761751));
#27283=CARTESIAN_POINT('Ctrl Pts',(0.111522209883364,-0.169480262890401,
0.796223099114019));
#27284=CARTESIAN_POINT('Ctrl Pts',(0.216377824064917,-0.0701823552026538,
0.803632291818555));
#27285=CARTESIAN_POINT('Ctrl Pts',(0.176251134310715,0.144153545294923,
0.814746080875359));
#27286=CARTESIAN_POINT('Ctrl Pts',(-0.025495812948363,0.226047524998972,
0.825859869932164));
#27287=CARTESIAN_POINT('Ctrl Pts',(-0.203756063475674,0.101284604698293,
0.836973658988968));
#27288=CARTESIAN_POINT('Ctrl Pts',(-0.195593983451704,-0.116312855641356,
0.848087448045772));
#27289=CARTESIAN_POINT('Ctrl Pts',(-0.0083618822819891,-0.227381363005354,
0.859201237102576));
#27290=CARTESIAN_POINT('Ctrl Pts',(0.186502733326074,-0.130359827804384,
0.87031502615938));
#27291=CARTESIAN_POINT('Ctrl Pts',(0.210670357962369,0.0859996535173407,
0.881428815216184));
#27292=CARTESIAN_POINT('Ctrl Pts',(0.0420032309836913,0.223633215949719,
0.892542604272988));
#27293=CARTESIAN_POINT('Ctrl Pts',(-0.16510690935118,0.156577700042264,
0.903656393329793));
#27294=CARTESIAN_POINT('Ctrl Pts',(-0.221094400331606,-0.0537977403094414,
0.914770182386598));
#27295=CARTESIAN_POINT('Ctrl Pts',(-0.0747108556819193,-0.214930151626042,
0.925883971443401));
#27296=CARTESIAN_POINT('Ctrl Pts',(0.140055952352658,-0.179335261208594,
0.936997760500206));
#27297=CARTESIAN_POINT('Ctrl Pts',(0.226628183455449,0.0204075949748767,
0.948111549557009));
#27298=CARTESIAN_POINT('Ctrl Pts',(0.105764950816784,0.201470956192298,
0.959225338613814));
#27299=CARTESIAN_POINT('Ctrl Pts',(-0.111906079513391,0.198125766554245,
0.970339127670618));
#27300=CARTESIAN_POINT('Ctrl Pts',(-0.227148238147163,0.0134337635740443,
0.981452916727423));
#27301=CARTESIAN_POINT('Ctrl Pts',(-0.134479021666759,-0.183554288235144,
0.992566705784226));
#27302=CARTESIAN_POINT('Ctrl Pts',(0.0812803597193106,-0.212533032641853,
1.00368049484103));
#27303=CARTESIAN_POINT('Ctrl Pts',(0.222642910626845,-0.0469778745330203,
1.01479428389783));
#27304=CARTESIAN_POINT('Ctrl Pts',(0.160217878116906,0.161576661010844,
1.02590807295464));
#27305=CARTESIAN_POINT('Ctrl Pts',(-0.0488563939857563,0.222238248359082,
1.03702186201144));
#27306=CARTESIAN_POINT('Ctrl Pts',(-0.21321185525264,0.0794826455702088,
1.04813565106825));
#27307=CARTESIAN_POINT('Ctrl Pts',(-0.182412087081199,-0.136024323549586,
1.05924944012505));
#27308=CARTESIAN_POINT('Ctrl Pts',(0.0153515329125665,-0.227026686992996,
1.07036322918186));
#27309=CARTESIAN_POINT('Ctrl Pts',(0.199063720825595,-0.110228949022901,
1.08147701823866));
#27310=CARTESIAN_POINT('Ctrl Pts',(0.200570627482587,0.107462595990271,
1.09259080729546));
#27311=CARTESIAN_POINT('Ctrl Pts',(0.0184929642043311,0.226792408226016,
1.10370459635227));
#27312=CARTESIAN_POINT('Ctrl Pts',(-0.180511518947779,0.138536557190134,
1.11481838540907));
#27313=CARTESIAN_POINT('Ctrl Pts',(-0.214291761660261,-0.0765233757420587,
1.12593217446588));
#27314=CARTESIAN_POINT('Ctrl Pts',(-0.0519283246948251,-0.221540595029306,
1.13704596352268));
#27315=CARTESIAN_POINT('Ctrl Pts',(0.157965696772913,-0.163779195241938,
1.14815975257948));
#27316=CARTESIAN_POINT('Ctrl Pts',(0.22327192453058,0.0438911593311794,
1.15927354163629));
#27317=CARTESIAN_POINT('Ctrl Pts',(0.0842148276900768,0.211387438009701,
1.17038733069309));
#27318=CARTESIAN_POINT('Ctrl Pts',(-0.131925055996524,0.185398397380911,
1.1815011197499));
#27319=CARTESIAN_POINT('Ctrl Pts',(-0.227312439797474,-0.0102878989312292,
1.1926149088067));
#27320=CARTESIAN_POINT('Ctrl Pts',(-0.114638169553469,-0.196557564679025,
1.20372869786351));
#27321=CARTESIAN_POINT('Ctrl Pts',(0.102965717368131,-0.202915862361653,
1.21484248692031));
#27322=CARTESIAN_POINT('Ctrl Pts',(0.226323915472005,-0.0235429700022985,
1.22595627597712));
#27323=CARTESIAN_POINT('Ctrl Pts',(0.142525267056592,0.177379069795616,
1.23707006503392));
#27324=CARTESIAN_POINT('Ctrl Pts',(-0.071728374642188,0.215944035394125,
1.24818385409072));
#27325=CARTESIAN_POINT('Ctrl Pts',(-0.220328221575874,0.0568529764244717,
1.25929764314753));
#27326=CARTESIAN_POINT('Ctrl Pts',(-0.16725914860919,-0.154276256623111,
1.27041143220433));
#27327=CARTESIAN_POINT('Ctrl Pts',(0.0389041199272518,-0.224194682371805,
1.28152522126113));
#27328=CARTESIAN_POINT('Ctrl Pts',(0.209458006291536,-0.088905172804972,
1.29263901031794));
#27329=CARTESIAN_POINT('Ctrl Pts',(0.188292604081856,0.127760249683509,
1.30375279937474));
#27330=CARTESIAN_POINT('Ctrl Pts',(-0.0052191540273722,0.227485266736855,
1.31486658843155));
#27331=CARTESIAN_POINT('Ctrl Pts',(-0.193953761266,0.118990439287648,1.32598037748835));
#27332=CARTESIAN_POINT('Ctrl Pts',(-0.205160291232821,-0.0984176866850601,
1.33709416654516));
#27333=CARTESIAN_POINT('Ctrl Pts',(-0.028581279957875,-0.225742987902158,
1.34820795560196));
#27334=CARTESIAN_POINT('Ctrl Pts',(0.174158500995476,-0.146443172193371,
1.35932174465876));
#27335=CARTESIAN_POINT('Ctrl Pts',(0.217489030897462,0.0668977398036206,
1.37043553371557));
#27336=CARTESIAN_POINT('Ctrl Pts',(0.0617493843227067,0.219006391884312,
1.38154932277237));
#27337=CARTESIAN_POINT('Ctrl Pts',(-0.150510174002661,0.17065600977586,
1.39266311182918));
#27338=CARTESIAN_POINT('Ctrl Pts',(-0.225006063172667,-0.0338977534588365,
1.40377690088598));
#27339=CARTESIAN_POINT('Ctrl Pts',(-0.0935513509578539,-0.207424518511403,
1.41489068994279));
#27340=CARTESIAN_POINT('Ctrl Pts',(0.123531973693776,-0.191093269444383,
1.42600447899959));
#27341=CARTESIAN_POINT('Ctrl Pts',(0.22754508195105,0.000147816343643338,
1.43711826805639));
#27342=CARTESIAN_POINT('Ctrl Pts',(0.123283596017355,0.191253604053547,
1.4482320571132));
#27343=CARTESIAN_POINT('Ctrl Pts',(-0.0938207632055154,0.207302799206008,
1.45934584617));
#27344=CARTESIAN_POINT('Ctrl Pts',(-0.225049914396199,0.033605390895932,
1.4704596352268));
#27345=CARTESIAN_POINT('Ctrl Pts',(-0.150288325686177,-0.170851412092914,
1.48157342428361));
#27346=CARTESIAN_POINT('Ctrl Pts',(0.0620338699676892,-0.218925981383812,
1.49268721334041));
#27347=CARTESIAN_POINT('Ctrl Pts',(0.217575764647534,-0.066615114486764,
1.50380100239722));
#27348=CARTESIAN_POINT('Ctrl Pts',(0.173968087346094,0.146669317115412,
1.51491479145402));
#27349=CARTESIAN_POINT('Ctrl Pts',(-0.0288745395963744,0.225705669091897,
1.52602858051083));
#27350=CARTESIAN_POINT('Ctrl Pts',(-0.205287999105225,0.0981510439482811,
1.53714236956763));
#27351=CARTESIAN_POINT('Ctrl Pts',(-0.1937989748928,-0.119242309357106,
1.54825615862444));
#27352=CARTESIAN_POINT('Ctrl Pts',(-0.00492364691005069,-0.227491892537031,
1.55936994768124));
#27353=CARTESIAN_POINT('Ctrl Pts',(0.188458534340702,-0.127515436462881,
1.57048373673804));
#27354=CARTESIAN_POINT('Ctrl Pts',(0.209342130614232,0.0891770956278107,
1.58159752579485));
#27355=CARTESIAN_POINT('Ctrl Pts',(0.0386131732285934,0.224245297773695,
1.59271131485165));
#27356=CARTESIAN_POINT('Ctrl Pts',(-0.167460147509052,0.154058322275268,
1.60382510390846));
#27357=CARTESIAN_POINT('Ctrl Pts',(-0.220252829642796,-0.057138233464333,
1.61493889296526));
#27358=CARTESIAN_POINT('Ctrl Pts',(-0.0714503221602304,-0.21603886592994,
1.62605268202207));
#27359=CARTESIAN_POINT('Ctrl Pts',(0.14276052028949,-0.177190259579807,
1.63716647107887));
#27360=CARTESIAN_POINT('Ctrl Pts',(0.226283718655826,0.0238303165896214,
1.64828026013567));
#27361=CARTESIAN_POINT('Ctrl Pts',(0.102720035411913,0.203062259110174,
1.65939404919248));
#27362=CARTESIAN_POINT('Ctrl Pts',(-0.114928016442956,0.196383949416646,
1.67050783824928));
#27363=CARTESIAN_POINT('Ctrl Pts',(-0.227259161518541,0.0100395986945998,
1.68162162730609));
#27364=CARTESIAN_POINT('Ctrl Pts',(-0.131813585150871,-0.185660673640335,
1.69273541636289));
#27365=CARTESIAN_POINT('Ctrl Pts',(0.0847577191513361,-0.211094895184898,
1.70384920541969));
#27366=CARTESIAN_POINT('Ctrl Pts',(0.176682876451709,-0.0997192257060721,
1.71125839812423));
#27367=CARTESIAN_POINT('Ctrl Pts',(0.188949368338152,-0.0368890654402894,
1.7149629944765));
#27368=CARTESIAN_POINT('Ctrl Pts',(0.0463299576986758,-0.173478327433381,
0.785037005523502));
#27369=CARTESIAN_POINT('Ctrl Pts',(0.104015628792176,-0.158072514262811,
0.78874160187577));
#27370=CARTESIAN_POINT('Ctrl Pts',(0.201813391703176,-0.0654583675678116,
0.796150794580307));
#27371=CARTESIAN_POINT('Ctrl Pts',(0.164387637044107,0.134450542830478,
0.80726458363711));
#27372=CARTESIAN_POINT('Ctrl Pts',(-0.0237796849449563,0.210832223234042,
0.818378372693916));
#27373=CARTESIAN_POINT('Ctrl Pts',(-0.190041204212204,0.0944671187531002,
0.829492161750717));
#27374=CARTESIAN_POINT('Ctrl Pts',(-0.182428515342129,-0.10848381527592,
0.840605950807524));
#27375=CARTESIAN_POINT('Ctrl Pts',(-0.00779904240022581,-0.212076280351327,
0.851719739864326));
#27376=CARTESIAN_POINT('Ctrl Pts',(0.173949198986102,-0.121585283079433,
0.862833528921132));
#27377=CARTESIAN_POINT('Ctrl Pts',(0.196490096226091,0.0802110005340724,
0.873947317977935));
#27378=CARTESIAN_POINT('Ctrl Pts',(0.0391759855426195,0.208580421784633,
0.885061107034741));
#27379=CARTESIAN_POINT('Ctrl Pts',(-0.153993531979477,0.146038425366231,
0.896174896091543));
#27380=CARTESIAN_POINT('Ctrl Pts',(-0.206212494327119,-0.0501766042094856,
0.907288685148349));
#27381=CARTESIAN_POINT('Ctrl Pts',(-0.0696820538212414,-0.200463162370631,
0.918402474205152));
#27382=CARTESIAN_POINT('Ctrl Pts',(0.130628759646036,-0.167264170775759,
0.929516263261957));
#27383=CARTESIAN_POINT('Ctrl Pts',(0.211373797459724,0.0190339558879606,
0.94063005231876));
#27384=CARTESIAN_POINT('Ctrl Pts',(0.098645891924909,0.187909907933315,
0.951743841375565));
#27385=CARTESIAN_POINT('Ctrl Pts',(-0.104373660084627,0.184789883644027,
0.962857630432369));
#27386=CARTESIAN_POINT('Ctrl Pts',(-0.21185884717154,0.0125295344009149,
0.973971419489173));
#27387=CARTESIAN_POINT('Ctrl Pts',(-0.125427213221957,-0.17119921429325,
0.985085208545978));
#27388=CARTESIAN_POINT('Ctrl Pts',(0.0758093632963375,-0.198227393919747,
0.996198997602781));
#27389=CARTESIAN_POINT('Ctrl Pts',(0.207656774100798,-0.0438157848914807,
1.00731278665959));
#27390=CARTESIAN_POINT('Ctrl Pts',(0.149433582364513,0.150700905324243,
1.01842657571639));
#27391=CARTESIAN_POINT('Ctrl Pts',(-0.0455678608436973,0.207279349727,1.0295403647732));
#27392=CARTESIAN_POINT('Ctrl Pts',(-0.198860524851901,0.0741326536274474,
1.04065415383));
#27393=CARTESIAN_POINT('Ctrl Pts',(-0.170133894915531,-0.126868500542071,
1.0517679428868));
#27394=CARTESIAN_POINT('Ctrl Pts',(0.0143182183216636,-0.211745477648606,
1.06288173194361));
#27395=CARTESIAN_POINT('Ctrl Pts',(0.185664704035542,-0.102809417565425,
1.07399552100041));
#27396=CARTESIAN_POINT('Ctrl Pts',(0.187070180519752,0.100229268279905,
1.08510931005721));
#27397=CARTESIAN_POINT('Ctrl Pts',(0.017248199277583,0.211526968229848,
1.09622309911402));
#27398=CARTESIAN_POINT('Ctrl Pts',(-0.168361254383508,0.12921163525997,
1.10733688817082));
#27399=CARTESIAN_POINT('Ctrl Pts',(-0.199867742554481,-0.07137257281249,
1.11845067722763));
#27400=CARTESIAN_POINT('Ctrl Pts',(-0.0484330193143192,-0.206628655575122,
1.12956446628443));
#27401=CARTESIAN_POINT('Ctrl Pts',(0.147332995773784,-0.152755186558655,
1.14067825534124));
#27402=CARTESIAN_POINT('Ctrl Pts',(0.208243448959415,0.0409368370750985,
1.15179204439804));
#27403=CARTESIAN_POINT('Ctrl Pts',(0.0785463116716341,0.197158909479484,
1.16290583345485));
#27404=CARTESIAN_POINT('Ctrl Pts',(-0.123045155465202,0.172919196102783,
1.17401962251165));
#27405=CARTESIAN_POINT('Ctrl Pts',(-0.212011996377637,-0.00959541850364452,
1.18513341156845));
#27406=CARTESIAN_POINT('Ctrl Pts',(-0.106921852626119,-0.18332723773435,
1.19624720062526));
#27407=CARTESIAN_POINT('Ctrl Pts',(0.0960350754104022,-0.189257557194465,
1.20736098968206));
#27408=CARTESIAN_POINT('Ctrl Pts',(0.211090009811934,-0.0219582882278384,
1.21847477873886));
#27409=CARTESIAN_POINT('Ctrl Pts',(0.132931864309081,0.16543965097767,1.22958856779567));
#27410=CARTESIAN_POINT('Ctrl Pts',(-0.0669003241457547,0.201408801430058,
1.24070235685247));
#27411=CARTESIAN_POINT('Ctrl Pts',(-0.205497887208699,0.0530261918023587,
1.25181614590928));
#27412=CARTESIAN_POINT('Ctrl Pts',(-0.156000903604979,-0.143891892539961,
1.26292993496608));
#27413=CARTESIAN_POINT('Ctrl Pts',(0.0362854762389619,-0.209104095795397,
1.27404372402289));
#27414=CARTESIAN_POINT('Ctrl Pts',(0.195359348176077,-0.0829209487675844,
1.28515751307969));
#27415=CARTESIAN_POINT('Ctrl Pts',(0.175618593201963,0.119160683054738,
1.2962713021365));
#27416=CARTESIAN_POINT('Ctrl Pts',(-0.00486785178026968,0.212173190302961,
1.3073850911933));
#27417=CARTESIAN_POINT('Ctrl Pts',(-0.180898696822721,0.110981170259326,
1.3184988802501));
#27418=CARTESIAN_POINT('Ctrl Pts',(-0.191350913132785,-0.0917931735348885,
1.32961266930691));
#27419=CARTESIAN_POINT('Ctrl Pts',(-0.026657468585072,-0.210548184586953,
1.34072645836371));
#27420=CARTESIAN_POINT('Ctrl Pts',(0.162435859274068,-0.136586054508292,
1.35184024742051));
#27421=CARTESIAN_POINT('Ctrl Pts',(0.202849802993145,0.0623948402540306,
1.36295403647732));
#27422=CARTESIAN_POINT('Ctrl Pts',(0.057593021556634,0.204265030124287,
1.37406782553412));
#27423=CARTESIAN_POINT('Ctrl Pts',(-0.14037930565472,0.159169121402496,
1.38518161459093));
#27424=CARTESIAN_POINT('Ctrl Pts',(-0.209860862400721,-0.0316160892467124,
1.39629540364773));
#27425=CARTESIAN_POINT('Ctrl Pts',(-0.0872543917881084,-0.193462734843961,
1.40740919270454));
#27426=CARTESIAN_POINT('Ctrl Pts',(0.11521701312353,-0.178230745247949,
1.41852298176134));
#27427=CARTESIAN_POINT('Ctrl Pts',(0.212228979343748,0.000137866797527619,
1.42963677081814));
#27428=CARTESIAN_POINT('Ctrl Pts',(0.1149853537956,0.178380287704172,1.44075055987495));
#27429=CARTESIAN_POINT('Ctrl Pts',(-0.0875056698463009,0.19334920848809,
1.45186434893175));
#27430=CARTESIAN_POINT('Ctrl Pts',(-0.209901761990083,0.0313434056633472,
1.46297813798856));
#27431=CARTESIAN_POINT('Ctrl Pts',(-0.14017238999048,-0.159351371152542,
1.47409192704536));
#27432=CARTESIAN_POINT('Ctrl Pts',(0.0578583584189162,-0.204190032069821,
1.48520571610217));
#27433=CARTESIAN_POINT('Ctrl Pts',(0.202930698678054,-0.0621312385008357,
1.49631950515897));
#27434=CARTESIAN_POINT('Ctrl Pts',(0.162258262403527,0.136796977572755,
1.50743329421577));
#27435=CARTESIAN_POINT('Ctrl Pts',(-0.0269309888617035,0.210513377712887,
1.51854708327258));
#27436=CARTESIAN_POINT('Ctrl Pts',(-0.191470024964085,0.0915444785712757,
1.52966087232938));
#27437=CARTESIAN_POINT('Ctrl Pts',(-0.180754329149647,-0.111216086906656,
1.54077466138619));
#27438=CARTESIAN_POINT('Ctrl Pts',(-0.00459223530304152,-0.212179370119272,
1.55188845044299));
#27439=CARTESIAN_POINT('Ctrl Pts',(0.175773354663627,-0.118932348258406,
1.5630022394998));
#27440=CARTESIAN_POINT('Ctrl Pts',(0.195251272112581,0.0831745684136627,
1.5741160285566));
#27441=CARTESIAN_POINT('Ctrl Pts',(0.0360141132177518,0.20915130426499,
1.5852298176134));
#27442=CARTESIAN_POINT('Ctrl Pts',(-0.156188373230783,0.14368862739439,
1.59634360667021));
#27443=CARTESIAN_POINT('Ctrl Pts',(-0.20542756992093,-0.0532922481367839,
1.60745739572701));
#27444=CARTESIAN_POINT('Ctrl Pts',(-0.0666409874290749,-0.201497248904528,
1.61857118478382));
#27445=CARTESIAN_POINT('Ctrl Pts',(0.13315128260227,-0.165263549613285,
1.62968497384062));
#27446=CARTESIAN_POINT('Ctrl Pts',(0.211052518651072,0.0222262934618894,
1.64079876289742));
#27447=CARTESIAN_POINT('Ctrl Pts',(0.095805930353238,0.189394099950088,
1.65191255195423));
#27448=CARTESIAN_POINT('Ctrl Pts',(-0.107192189866521,0.183165308548198,
1.66302634101103));
#27449=CARTESIAN_POINT('Ctrl Pts',(-0.21196230426976,0.00936383140301889,
1.67414013006784));
#27450=CARTESIAN_POINT('Ctrl Pts',(-0.122941187743304,-0.173163818497459,
1.68525391912464));
#27451=CARTESIAN_POINT('Ctrl Pts',(0.0790526610057068,-0.196886057767682,
1.69636770818145));
#27452=CARTESIAN_POINT('Ctrl Pts',(0.164790318539736,-0.0930071057176319,
1.70377690088598));
#27453=CARTESIAN_POINT('Ctrl Pts',(0.176231150531649,-0.034406055451559,
1.70748149723825));
#27454=CARTESIAN_POINT('Ctrl Pts',(0.0429864256885843,-0.160958774866485,
0.777555508285253));
#27455=CARTESIAN_POINT('Ctrl Pts',(0.0965090477009877,-0.146664765635222,
0.781260104637521));
#27456=CARTESIAN_POINT('Ctrl Pts',(0.187248959341434,-0.0607343799329692,
0.788669297342056));
#27457=CARTESIAN_POINT('Ctrl Pts',(0.1525241397775,0.124747540366033,0.799783086398862));
#27458=CARTESIAN_POINT('Ctrl Pts',(-0.0220635569415495,0.195616921469113,
0.810896875455666));
#27459=CARTESIAN_POINT('Ctrl Pts',(-0.176326344948735,0.0876496328079073,
0.82201066451247));
#27460=CARTESIAN_POINT('Ctrl Pts',(-0.169263047232554,-0.100654774910484,
0.833124453569274));
#27461=CARTESIAN_POINT('Ctrl Pts',(-0.00723620251846265,-0.196771197697301,
0.844238242626078));
#27462=CARTESIAN_POINT('Ctrl Pts',(0.161395664646129,-0.112810738354482,
0.855352031682883));
#27463=CARTESIAN_POINT('Ctrl Pts',(0.182309834489814,0.0744223475508041,
0.866465820739686));
#27464=CARTESIAN_POINT('Ctrl Pts',(0.0363487401015477,0.193527627619547,
0.877579609796491));
#27465=CARTESIAN_POINT('Ctrl Pts',(-0.142880154607774,0.135499150690198,
0.888693398853294));
#27466=CARTESIAN_POINT('Ctrl Pts',(-0.191330588322633,-0.0465554681095297,
0.8998071879101));
#27467=CARTESIAN_POINT('Ctrl Pts',(-0.0646532519605634,-0.185996173115221,
0.910920976966903));
#27468=CARTESIAN_POINT('Ctrl Pts',(0.121201566939414,-0.155193080342923,
0.922034766023707));
#27469=CARTESIAN_POINT('Ctrl Pts',(0.196119411464,0.0176603168010446,0.933148555080512));
#27470=CARTESIAN_POINT('Ctrl Pts',(0.0915268330330338,0.174348859674332,
0.944262344137316));
#27471=CARTESIAN_POINT('Ctrl Pts',(-0.0968412406558618,0.17145400073381,
0.95537613319412));
#27472=CARTESIAN_POINT('Ctrl Pts',(-0.196569456195918,0.0116253052277854,
0.966489922250924));
#27473=CARTESIAN_POINT('Ctrl Pts',(-0.116375404777155,-0.158844140351355,
0.977603711307728));
#27474=CARTESIAN_POINT('Ctrl Pts',(0.0703383668733642,-0.183921755197642,
0.988717500364533));
#27475=CARTESIAN_POINT('Ctrl Pts',(0.19267063757475,-0.0406536952499414,
0.999831289421336));
#27476=CARTESIAN_POINT('Ctrl Pts',(0.13864928661212,0.139825149637642,1.01094507847814));
#27477=CARTESIAN_POINT('Ctrl Pts',(-0.0422793277016381,0.192320451094917,
1.02205886753494));
#27478=CARTESIAN_POINT('Ctrl Pts',(-0.184509194451163,0.0687826616846859,
1.03317265659175));
#27479=CARTESIAN_POINT('Ctrl Pts',(-0.157855702749863,-0.117712677534557,
1.04428644564855));
#27480=CARTESIAN_POINT('Ctrl Pts',(0.0132849037307607,-0.196464268304215,
1.05540023470536));
#27481=CARTESIAN_POINT('Ctrl Pts',(0.172265687245489,-0.0953898861079487,
1.06651402376216));
#27482=CARTESIAN_POINT('Ctrl Pts',(0.173569733556916,0.0929959405695393,
1.07762781281897));
#27483=CARTESIAN_POINT('Ctrl Pts',(0.0160034343508349,0.196261528233681,
1.08874160187577));
#27484=CARTESIAN_POINT('Ctrl Pts',(-0.156210989819237,0.119886713329805,
1.09985539093257));
#27485=CARTESIAN_POINT('Ctrl Pts',(-0.185443723448703,-0.066221769882921,
1.11096917998938));
#27486=CARTESIAN_POINT('Ctrl Pts',(-0.0449377139338128,-0.191716716120937,
1.12208296904618));
#27487=CARTESIAN_POINT('Ctrl Pts',(0.136700294774655,-0.141731177875371,
1.13319675810299));
#27488=CARTESIAN_POINT('Ctrl Pts',(0.193214973388251,0.0379825148190173,
1.14431054715979));
#27489=CARTESIAN_POINT('Ctrl Pts',(0.0728777956531908,0.182930380949266,
1.1554243362166));
#27490=CARTESIAN_POINT('Ctrl Pts',(-0.11416525493388,0.160439994824655,
1.1665381252734));
#27491=CARTESIAN_POINT('Ctrl Pts',(-0.196711552957801,-0.00890293807605981,
1.1776519143302));
#27492=CARTESIAN_POINT('Ctrl Pts',(-0.0992055356987686,-0.170096910789675,
1.18876570338701));
#27493=CARTESIAN_POINT('Ctrl Pts',(0.0891044334526734,-0.175599252027278,
1.19987949244381));
#27494=CARTESIAN_POINT('Ctrl Pts',(0.195856104151863,-0.0203736064533785,
1.21099328150062));
#27495=CARTESIAN_POINT('Ctrl Pts',(0.12333846156157,0.153500232159725,1.22210707055742));
#27496=CARTESIAN_POINT('Ctrl Pts',(-0.0620722736493212,0.186873567465992,
1.23322085961422));
#27497=CARTESIAN_POINT('Ctrl Pts',(-0.190667552841524,0.0491994071802457,
1.24433464867103));
#27498=CARTESIAN_POINT('Ctrl Pts',(-0.144742658600767,-0.13350752845681,
1.25544843772783));
#27499=CARTESIAN_POINT('Ctrl Pts',(0.0336668325506717,-0.194013509218991,
1.26656222678464));
#27500=CARTESIAN_POINT('Ctrl Pts',(0.181260690060617,-0.0769367247301966,
1.27767601584144));
#27501=CARTESIAN_POINT('Ctrl Pts',(0.16294458232207,0.110561116425968,1.28878980489824));
#27502=CARTESIAN_POINT('Ctrl Pts',(-0.00451654953316709,0.196861113869068,
1.29990359395505));
#27503=CARTESIAN_POINT('Ctrl Pts',(-0.167843632379442,0.102971901231004,
1.31101738301185));
#27504=CARTESIAN_POINT('Ctrl Pts',(-0.177541535032749,-0.0851686603847167,
1.32213117206866));
#27505=CARTESIAN_POINT('Ctrl Pts',(-0.0247336572122691,-0.195353381271748,
1.33324496112546));
#27506=CARTESIAN_POINT('Ctrl Pts',(0.15071321755266,-0.126728936823214,
1.34435875018226));
#27507=CARTESIAN_POINT('Ctrl Pts',(0.188210575088826,0.0578919407044404,
1.35547253923907));
#27508=CARTESIAN_POINT('Ctrl Pts',(0.0534366587905616,0.189523668364262,
1.36658632829587));
#27509=CARTESIAN_POINT('Ctrl Pts',(-0.130248437306779,0.147682233029131,
1.37770011735268));
#27510=CARTESIAN_POINT('Ctrl Pts',(-0.194715661628775,-0.0293344250345881,
1.38881390640948));
#27511=CARTESIAN_POINT('Ctrl Pts',(-0.0809574326183627,-0.17950095117652,
1.39992769546629));
#27512=CARTESIAN_POINT('Ctrl Pts',(0.106902052553284,-0.165368221051515,
1.41104148452309));
#27513=CARTESIAN_POINT('Ctrl Pts',(0.196912876736446,0.000127917251411783,
1.4221552735799));
#27514=CARTESIAN_POINT('Ctrl Pts',(0.106687111573845,0.165506971354797,
1.4332690626367));
#27515=CARTESIAN_POINT('Ctrl Pts',(-0.0811905764870862,0.179395617770172,
1.44438285169351));
#27516=CARTESIAN_POINT('Ctrl Pts',(-0.194753609583967,0.0290814204307625,
1.45549664075031));
#27517=CARTESIAN_POINT('Ctrl Pts',(-0.130056454294782,-0.14785133021217,
1.46661042980711));
#27518=CARTESIAN_POINT('Ctrl Pts',(0.053682846870143,-0.189454082755829,
1.47772421886392));
#27519=CARTESIAN_POINT('Ctrl Pts',(0.188285632708575,-0.0576473625149073,
1.48883800792072));
#27520=CARTESIAN_POINT('Ctrl Pts',(0.15054843746096,0.126924638030098,1.49995179697752));
#27521=CARTESIAN_POINT('Ctrl Pts',(-0.024987438127033,0.195321086333876,
1.51106558603433));
#27522=CARTESIAN_POINT('Ctrl Pts',(-0.177652050822945,0.0849379131942705,
1.52217937509113));
#27523=CARTESIAN_POINT('Ctrl Pts',(-0.167709683406495,-0.103189864456206,
1.53329316414794));
#27524=CARTESIAN_POINT('Ctrl Pts',(-0.00426082369603206,-0.196866847701512,
1.54440695320474));
#27525=CARTESIAN_POINT('Ctrl Pts',(0.163088174986552,-0.110349260053931,
1.55552074226154));
#27526=CARTESIAN_POINT('Ctrl Pts',(0.181160413610931,0.0771720411995148,
1.56663453131835));
#27527=CARTESIAN_POINT('Ctrl Pts',(0.03341505320691,0.194057310756286,1.57774832037515));
#27528=CARTESIAN_POINT('Ctrl Pts',(-0.144916598952513,0.133318932513512,
1.58886210943196));
#27529=CARTESIAN_POINT('Ctrl Pts',(-0.190602310199064,-0.049446262809235,
1.59997589848876));
#27530=CARTESIAN_POINT('Ctrl Pts',(-0.0618316526979189,-0.186955631879117,
1.61108968754557));
#27531=CARTESIAN_POINT('Ctrl Pts',(0.12354204491505,-0.153336839646763,
1.62220347660237));
#27532=CARTESIAN_POINT('Ctrl Pts',(0.195821318646319,0.0206222703341576,
1.63331726565918));
#27533=CARTESIAN_POINT('Ctrl Pts',(0.0888918252945621,0.175725940790001,
1.64443105471598));
#27534=CARTESIAN_POINT('Ctrl Pts',(-0.0994563632900866,0.16994666767975,
1.65554484377278));
#27535=CARTESIAN_POINT('Ctrl Pts',(-0.19666544702098,0.008688064111438,
1.66665863282959));
#27536=CARTESIAN_POINT('Ctrl Pts',(-0.114068790335738,-0.160666963354583,
1.67777242188639));
#27537=CARTESIAN_POINT('Ctrl Pts',(0.0733476028600775,-0.182677220350466,
1.6888862109432));
#27538=CARTESIAN_POINT('Ctrl Pts',(0.152897760627763,-0.0862949857291919,
1.69629540364773));
#27539=CARTESIAN_POINT('Ctrl Pts',(0.163512932725146,-0.0319230454628286,
1.7));
#27540=CARTESIAN_POINT('Ctrl Pts',(0.166381444272219,9.40568719243839E-5,
0.86214803633902));
#27541=CARTESIAN_POINT('Ctrl Pts',(0.166493197029431,0.0216823422355625,
0.863587297805909));
#27542=CARTESIAN_POINT('Ctrl Pts',(0.162594223870085,0.0432319486948127,
0.865026559272798));
#27543=CARTESIAN_POINT('Ctrl Pts',(0.154497290451155,0.0630677132447136,
0.866465820739686));
#27544=CARTESIAN_POINT('Ctrl Pts',(0.133656136360392,0.114124107573719,
0.870170417091954));
#27545=CARTESIAN_POINT('Ctrl Pts',(0.0850024382309698,0.153825867596633,
0.873875013444223));
#27546=CARTESIAN_POINT('Ctrl Pts',(0.0308041067147051,0.164005334786532,
0.877579609796491));
#27547=CARTESIAN_POINT('Ctrl Pts',(-0.0233942248015594,0.174184801976431,
0.881284206148759));
#27548=CARTESIAN_POINT('Ctrl Pts',(-0.0831371897046666,0.154841976333314,
0.884988802501027));
#27549=CARTESIAN_POINT('Ctrl Pts',(-0.12108374444203,0.114828127045135,
0.888693398853295));
#27550=CARTESIAN_POINT('Ctrl Pts',(-0.159030299179393,0.0748142777569551,
0.892397995205563));
#27551=CARTESIAN_POINT('Ctrl Pts',(-0.175180443751013,0.0141294048237127,
0.896102591557831));
#27552=CARTESIAN_POINT('Ctrl Pts',(-0.162142626643145,-0.039453149143857,
0.899807187910099));
#27553=CARTESIAN_POINT('Ctrl Pts',(-0.149104809535276,-0.0930357031114267,
0.903511784262367));
#27554=CARTESIAN_POINT('Ctrl Pts',(-0.10687903074792,-0.139515938113324,
0.907216380614635));
#27555=CARTESIAN_POINT('Ctrl Pts',(-0.0547903382042454,-0.157622206818889,
0.910920976966903));
#27556=CARTESIAN_POINT('Ctrl Pts',(-0.00270164566057092,-0.175728475524455,
0.914625573319171));
#27557=CARTESIAN_POINT('Ctrl Pts',(0.0592499606394216,-0.165460777933689,
0.918330169671439));
#27558=CARTESIAN_POINT('Ctrl Pts',(0.102712071210182,-0.131518029614312,
0.922034766023707));
#27559=CARTESIAN_POINT('Ctrl Pts',(0.142261505739626,-0.100630976850939,
0.925405856128812));
#27560=CARTESIAN_POINT('Ctrl Pts',(0.166500629757864,-0.0501396913203886,
0.928776946233916));
#27561=CARTESIAN_POINT('Ctrl Pts',(0.16681765906064,8.64047405809373E-5,
0.93214803633902));
#27562=CARTESIAN_POINT('Ctrl Pts',(0.0530170217188587,-0.198517432567173,
0.8));
#27563=CARTESIAN_POINT('Ctrl Pts',(0.0654219024915668,-0.193924365121538,
0.8));
#27564=CARTESIAN_POINT('Ctrl Pts',(0.0772726753754473,-0.188065368475528,
0.8));
#27565=CARTESIAN_POINT('Ctrl Pts',(0.0884514733522922,-0.181103303150236,
0.8));
#27566=CARTESIAN_POINT('Ctrl Pts',(0.09412650504638,-0.177568939128346,
0.8));
#27567=CARTESIAN_POINT('Ctrl Pts',(0.0996279181736098,-0.173749544851002,
0.8));
#27568=CARTESIAN_POINT('Ctrl Pts',(0.104936837602987,-0.16966283510169,
0.8));
#27569=CARTESIAN_POINT('Ctrl Pts',(0.10962098777257,-0.166057061380704,
0.8));
#27570=CARTESIAN_POINT('Ctrl Pts',(0.114155265023366,-0.162243133727946,
0.8));
#27571=CARTESIAN_POINT('Ctrl Pts',(0.118524756406352,-0.158232269033094,
0.8));
#27572=CARTESIAN_POINT('Ctrl Pts',(0.121396569737292,-0.155596160230106,
0.8));
#27573=CARTESIAN_POINT('Ctrl Pts',(0.124191187364035,-0.152880333162932,
0.8));
#27574=CARTESIAN_POINT('Ctrl Pts',(0.126901910586196,-0.150092210881471,
0.8));
#27575=CARTESIAN_POINT('Ctrl Pts',(0.135875513595552,-0.140862385316535,
0.8));
#27576=CARTESIAN_POINT('Ctrl Pts',(0.143945927205397,-0.130830324459656,
0.8));
#27577=CARTESIAN_POINT('Ctrl Pts',(0.150974563153614,-0.120127060905897,
0.8));
#27578=CARTESIAN_POINT('Ctrl Pts',(0.155531899783608,-0.113187111901085,
0.8));
#27579=CARTESIAN_POINT('Ctrl Pts',(0.159650421905677,-0.105964391211092,
0.8));
#27580=CARTESIAN_POINT('Ctrl Pts',(0.163280590687062,-0.0984918775736134,
0.8));
#27581=CARTESIAN_POINT('Ctrl Pts',(0.165013714615195,-0.0949243321044268,
0.8));
#27582=CARTESIAN_POINT('Ctrl Pts',(0.166631773157808,-0.0913069558365289,
0.8));
#27583=CARTESIAN_POINT('Ctrl Pts',(0.168128066663937,-0.0876495022602451,
0.8));
#27584=CARTESIAN_POINT('Ctrl Pts',(0.172146949722996,-0.0778259762228617,
0.8));
#27585=CARTESIAN_POINT('Ctrl Pts',(0.175295994023174,-0.0677004884915743,
0.8));
#27586=CARTESIAN_POINT('Ctrl Pts',(0.177480263226672,-0.0573468152173212,
0.8));
#27587=CARTESIAN_POINT('Ctrl Pts',(0.179333801272362,-0.048560843554235,
0.8));
#27588=CARTESIAN_POINT('Ctrl Pts',(0.180491858406323,-0.0396100717078052,
0.8));
#27589=CARTESIAN_POINT('Ctrl Pts',(0.18096708784323,-0.0305729202789466,
0.8));
#27590=CARTESIAN_POINT('Ctrl Pts',(0.181136159028966,-0.0273577955642423,
0.8));
#27591=CARTESIAN_POINT('Ctrl Pts',(0.181218443079545,-0.0241331712280784,
0.8));
#27592=CARTESIAN_POINT('Ctrl Pts',(0.181214870924098,-0.0209122942089756,
0.8));
#27593=CARTESIAN_POINT('Ctrl Pts',(0.1812018830209,-0.00920159472786908,
0.8));
#27594=CARTESIAN_POINT('Ctrl Pts',(0.180059445076844,0.00249593154933228,
0.8));
#27595=CARTESIAN_POINT('Ctrl Pts',(0.177833010924532,0.0140076329059244,
0.8));
#27596=CARTESIAN_POINT('Ctrl Pts',(0.176687470499003,0.019930610352574,
0.8));
#27597=CARTESIAN_POINT('Ctrl Pts',(0.17525426981669,0.0258042115192748,
0.8));
#27598=CARTESIAN_POINT('Ctrl Pts',(0.173535645755736,0.0316026384872638,
0.8));
#27599=CARTESIAN_POINT('Ctrl Pts',(0.171850920647243,0.0372866945438873,
0.8));
#27600=CARTESIAN_POINT('Ctrl Pts',(0.169889181319091,0.0429039115259332,
0.8));
#27601=CARTESIAN_POINT('Ctrl Pts',(0.167664346683561,0.0483972355746533,
0.8));
#27602=CARTESIAN_POINT('Ctrl Pts',(0.16420912784319,0.0569284928853236,
0.8));
#27603=CARTESIAN_POINT('Ctrl Pts',(0.160117674787075,0.065174591642692,
0.8));
#27604=CARTESIAN_POINT('Ctrl Pts',(0.155399354804051,0.073039643321633,
0.8));
#27605=CARTESIAN_POINT('Ctrl Pts',(0.15298274940935,0.0770679259275847,
0.8));
#27606=CARTESIAN_POINT('Ctrl Pts',(0.150400765188628,0.0809963604120499,
0.8));
#27607=CARTESIAN_POINT('Ctrl Pts',(0.147663479517856,0.0847983168718068,
0.8));
#27608=CARTESIAN_POINT('Ctrl Pts',(0.142228073022467,0.0923478317277872,
0.8));
#27609=CARTESIAN_POINT('Ctrl Pts',(0.136173701728632,0.0994134091821942,
0.8));
#27610=CARTESIAN_POINT('Ctrl Pts',(0.129505054411736,0.105883695181419,
0.8));
#27611=CARTESIAN_POINT('Ctrl Pts',(0.128726565799248,0.106639027369579,
0.8));
#27612=CARTESIAN_POINT('Ctrl Pts',(0.127939691591626,0.107386221438147,
0.8));
#27613=CARTESIAN_POINT('Ctrl Pts',(0.127144588893496,0.108125211870903,
0.8));
#27614=CARTESIAN_POINT('Origin',(0.,0.,1.3));
#27615=CARTESIAN_POINT('Origin',(0.,0.,1.8));
#27616=CARTESIAN_POINT('Origin',(0.4,0.6,0.8));
#27617=CARTESIAN_POINT('',(0.4,0.6,0.8));
#27618=CARTESIAN_POINT('',(-0.4,0.6,0.8));
#27619=CARTESIAN_POINT('',(0.4,0.6,0.8));
#27620=CARTESIAN_POINT('',(-0.4,0.6,3.6));
#27621=CARTESIAN_POINT('',(-0.4,0.6,0.8));
#27622=CARTESIAN_POINT('',(0.4,0.6,3.6));
#27623=CARTESIAN_POINT('',(0.4,0.6,3.6));
#27624=CARTESIAN_POINT('',(0.4,0.6,0.8));
#27625=CARTESIAN_POINT('Origin',(0.4,-0.6,0.8));
#27626=CARTESIAN_POINT('',(0.4,-0.6,0.8));
#27627=CARTESIAN_POINT('',(0.4,-0.6,0.8));
#27628=CARTESIAN_POINT('',(0.4,-0.6,3.6));
#27629=CARTESIAN_POINT('',(0.4,-0.6,3.6));
#27630=CARTESIAN_POINT('',(0.4,-0.6,0.8));
#27631=CARTESIAN_POINT('Origin',(-0.4,-0.6,0.8));
#27632=CARTESIAN_POINT('',(-0.4,-0.6,0.8));
#27633=CARTESIAN_POINT('',(-0.4,-0.6,0.8));
#27634=CARTESIAN_POINT('',(-0.4,-0.6,3.6));
#27635=CARTESIAN_POINT('',(-0.4,-0.6,3.6));
#27636=CARTESIAN_POINT('',(-0.4,-0.6,0.8));
#27637=CARTESIAN_POINT('Origin',(-0.4,0.6,0.8));
#27638=CARTESIAN_POINT('',(-0.4,0.6,0.8));
#27639=CARTESIAN_POINT('',(-0.4,0.6,3.6));
#27640=CARTESIAN_POINT('Origin',(0.,0.,3.6));
#27641=CARTESIAN_POINT('Origin',(0.,0.,0.8));
#36452=UNCERTAINTY_MEASURE_WITH_UNIT(LENGTH_MEASURE(0.001),#36483,
'DISTANCE_ACCURACY_VALUE',
'Maximum model space distance between geometric entities at asserted c
onnectivities');
#36463=UNCERTAINTY_MEASURE_WITH_UNIT(LENGTH_MEASURE(0.001),#36483,
'DISTANCE_ACCURACY_VALUE',
'Maximum model space distance between geometric entities at asserted c
onnectivities');
#36471=(
GEOMETRIC_REPRESENTATION_CONTEXT(3)
GLOBAL_UNCERTAINTY_ASSIGNED_CONTEXT((#36452))
GLOBAL_UNIT_ASSIGNED_CONTEXT((#36483,#36485,#36486))
REPRESENTATION_CONTEXT('','3D')
);
#36482=(
GEOMETRIC_REPRESENTATION_CONTEXT(3)
GLOBAL_UNCERTAINTY_ASSIGNED_CONTEXT((#36463))
GLOBAL_UNIT_ASSIGNED_CONTEXT((#36483,#36485,#36486))
REPRESENTATION_CONTEXT('','3D')
);
#36483=(
LENGTH_UNIT()
NAMED_UNIT(*)
SI_UNIT(.CENTI.,.METRE.)
);
#36485=(
NAMED_UNIT(*)
PLANE_ANGLE_UNIT()
SI_UNIT($,.RADIAN.)
);
#36486=(
NAMED_UNIT(*)
SI_UNIT($,.STERADIAN.)
SOLID_ANGLE_UNIT()
);
#36494=SHAPE_DEFINITION_REPRESENTATION(#36512,#36561);
#36512=PRODUCT_DEFINITION_SHAPE('',$,#36580);
#36561=SHAPE_REPRESENTATION('',(#10314),#36471);
#36572=PRODUCT_DEFINITION_CONTEXT('part definition',#36628,'design');
#36580=PRODUCT_DEFINITION('Terminal insulator','Terminal insulator',#36598,
#36572);
#36598=PRODUCT_DEFINITION_FORMATION('',$,#36637);
#36628=APPLICATION_CONTEXT(
'Core Data for Automotive Mechanical Design Process');
#36629=PRODUCT_CONTEXT('part definition',#36628,'mechanical');
#36637=PRODUCT('Terminal insulator','Terminal insulator',$,(#36629));
#36655=PRESENTATION_STYLE_ASSIGNMENT((#36669));
#36669=SURFACE_STYLE_USAGE(.BOTH.,#36683);
#36683=SURFACE_SIDE_STYLE('',(#36697));
#36697=SURFACE_STYLE_FILL_AREA(#36711);
#36711=FILL_AREA_STYLE('Insulator gray',(#36725));
#36725=FILL_AREA_STYLE_COLOUR('Insulator gray',#36739);
#36739=COLOUR_RGB('Insulator gray',0.576470588235294,0.615686274509804,
0.666666666666667);
ENDSEC;
END-ISO-10303-21;
